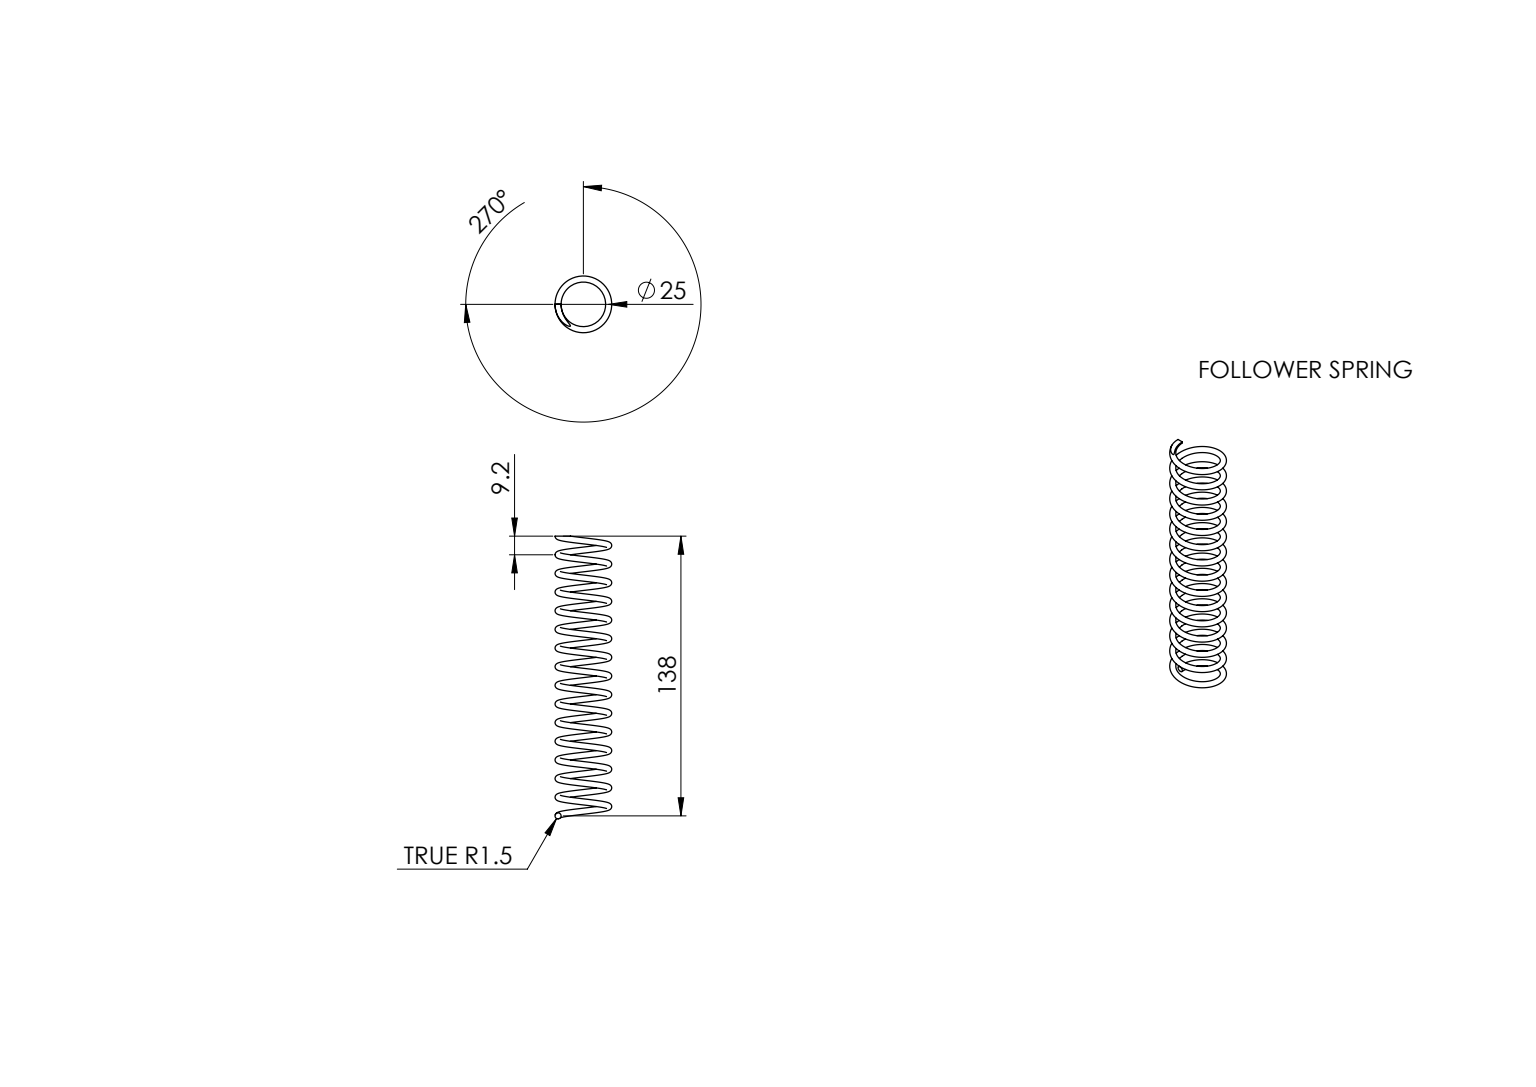
ISO-10303-21;
HEADER;
FILE_DESCRIPTION (('STEP AP214'),
    '1' );
FILE_NAME ('follower spring.step',
    '2026-10-31T03:36:27',
    ( '' ),
    ( '' ),
    'SwSTEP 2.0',
    'SolidWorks 2026',
    '' );
FILE_SCHEMA (( 'AUTOMOTIVE_DESIGN' ));
ENDSEC;

DATA;
#5=CARTESIAN_POINT ( 'NONE',  ( 6.840914352312096547, 71.36018628210143788, -6.594114490232313663 ) ) ;
#12=CARTESIAN_POINT ( 'NONE',  ( 1.715153634034445762, 36.67731371789854933, -9.534712964251895073 ) ) ;
#17=CARTESIAN_POINT ( 'NONE',  ( 6.932735513424201024, 37.25231371789855217, -10.69584247140429412 ) ) ;
#20=CARTESIAN_POINT ( 'NONE',  ( 13.23911966647199812, 140.7523137178985166, 8.632099005475788900 ) ) ;
#36=CARTESIAN_POINT ( 'NONE',  ( -13.23911966647199812, 25.75231371789854506, -8.632099005475788900 ) ) ;
#38=CARTESIAN_POINT ( 'NONE',  ( -9.500000000000005329, 141.5101862821014720, -0.1745138560725176813 ) ) ;
#39=CARTESIAN_POINT ( 'NONE',  ( 2.311890736173175753, 56.12268628210144072, 12.53471296425194836 ) ) ;
#49=CARTESIAN_POINT ( 'NONE',  ( 8.843639120294245259, 94.46481371789855075, 3.474262827703527901 ) ) ;
#56=CARTESIAN_POINT ( 'NONE',  ( -10.49813415416004858, 106.8273137178985479, 7.228626920338840023 ) ) ;
#60=CARTESIAN_POINT ( 'NONE',  ( 0.1745138560722779009, 68.58981371789856496, 12.50000000000000355 ) ) ;
#70=CARTESIAN_POINT ( 'NONE',  ( 12.53471296425194836, 44.62268628210144783, -2.311890736173178418 ) ) ;
#76=CARTESIAN_POINT ( 'NONE',  ( 0.1745138560722779009, 96.18981371789855928, 12.50000000000000355 ) ) ;
#82=CARTESIAN_POINT ( 'NONE',  ( -3.257655550456946880, 82.10231371789853938, -15.46528703574811736 ) ) ;
#86=CARTESIAN_POINT ( 'NONE',  ( -8.715434833791929847, 105.8601862821014521, -8.962234695871762469 ) ) ;
#87=CARTESIAN_POINT ( 'NONE',  ( 13.04141134922759804, 54.97268628210144215, 8.927990412390657937 ) ) ;
#92=CARTESIAN_POINT ( 'NONE',  ( -0.1745138560725817967, 74.81018628210145494, 15.50000000000000533 ) ) ;
#98=CARTESIAN_POINT ( 'NONE',  ( 11.48171059495397728, 45.48518628210145209, 4.944772684328674117 ) ) ;
#101=CARTESIAN_POINT ( 'NONE',  ( 9.534712964251900402, 140.1773137178985564, 1.715153634034445540 ) ) ;
#112=CARTESIAN_POINT ( 'NONE',  ( -12.53471296425194659, 67.62268628210145494, 2.311890736173176641 ) ) ;
#121=CARTESIAN_POINT ( 'NONE',  ( 8.632099005475788900, 46.45231371789854791, -13.23911966647199812 ) ) ;
#127=CARTESIAN_POINT ( 'NONE',  ( -3.474262827703527901, 23.16481371789855359, 8.843639120294245259 ) ) ;
#133=CARTESIAN_POINT ( 'NONE',  ( -3.257655550456946880, 137.3023137178985564, -15.46528703574811736 ) ) ;
#137=CARTESIAN_POINT ( 'NONE',  ( -4.622313124798576922, 42.03518628210144215, -11.61527771782819762 ) ) ;
#143=CARTESIAN_POINT ( 'NONE',  ( 8.710071997420127943, 82.28518628210146346, 3.796722387233375073 ) ) ;
#147=CARTESIAN_POINT ( 'NONE',  ( -12.53471296425194836, 86.02268628210146062, 2.311890736173176641 ) ) ;
#158=CARTESIAN_POINT ( 'NONE',  ( 0.1745138560722779009, 123.7898137178985678, 12.50000000000000355 ) ) ;
#159=CARTESIAN_POINT ( 'NONE',  ( -4.944772684328673229, 121.3851862821014578, 11.48171059495397728 ) ) ;
#166=CARTESIAN_POINT ( 'NONE',  ( -13.23911966647199812, 90.15231371789855075, -8.632099005475788900 ) ) ;
#171=CARTESIAN_POINT ( 'NONE',  ( 9.465287035748106703, 84.40231371789855075, -2.064181346179063237 ) ) ;
#174=CARTESIAN_POINT ( 'NONE',  ( 10.49813415416005213, 47.02731371789855075, -7.228626920338837358 ) ) ;
#178=CARTESIAN_POINT ( 'NONE',  ( 10.49813415415989581, 110.1726862821014521, 7.228626920339068285 ) ) ;
#181=CARTESIAN_POINT ( 'NONE',  ( -7.228626920339069173, 140.0726862821014720, 10.49813415415989581 ) ) ;
#183=CARTESIAN_POINT ( 'NONE',  ( -15.46528703574804986, 104.9976862821014549, -3.257655550457287497 ) ) ;
#184=CARTESIAN_POINT ( 'NONE',  ( 10.49813415415989581, 18.17268628210144499, 7.228626920339069173 ) ) ;
#187=CARTESIAN_POINT ( 'NONE',  ( 6.840914352312096547, 126.5601862821014834, -6.594114490232313663 ) ) ;
#192=CARTESIAN_POINT ( 'NONE',  ( -8.710071997420127943, 68.48518628210145209, -3.796722387233380402 ) ) ;
#202=CARTESIAN_POINT ( 'NONE',  ( -6.594114490232462877, 42.13981371789854791, 6.840914352311949109 ) ) ;
#207=CARTESIAN_POINT ( 'NONE',  ( -8.962234695871565293, 35.23981371789855643, -8.715434833792128799 ) ) ;
#210=CARTESIAN_POINT ( 'NONE',  ( 8.715434833792128799, 19.13981371789855146, -8.962234695871567070 ) ) ;
#225=CARTESIAN_POINT ( 'NONE',  ( -13.23911966647199812, 16.55231371789855643, -8.632099005475788900 ) ) ;
#228=CARTESIAN_POINT ( 'NONE',  ( 7.228626920339068285, 6.672686282101436106, -10.49813415415989581 ) ) ;
#229=CARTESIAN_POINT ( 'NONE',  ( 11.61527771782819940, 44.33518628210145351, -4.622313124798573369 ) ) ;
#241=CARTESIAN_POINT ( 'NONE',  ( -9.465287035748106703, 89.00231371789853085, 2.064181346179061460 ) ) ;
#246=CARTESIAN_POINT ( 'NONE',  ( -6.932735513424201912, 106.2523137178985593, 10.69584247140429412 ) ) ;
#250=CARTESIAN_POINT ( 'NONE',  ( -6.932735513424201912, 69.45231371789856212, 10.69584247140429412 ) ) ;
#258=CARTESIAN_POINT ( 'NONE',  ( 11.48171059495397728, 36.28518628210144925, 4.944772684328674117 ) ) ;
#265=CARTESIAN_POINT ( 'NONE',  ( 11.48171059495408208, 111.7148137178985650, -4.944772684328420986 ) ) ;
#270=CARTESIAN_POINT ( 'NONE',  ( 13.23911966647199812, 76.35231371789853938, 8.632099005475788900 ) ) ;
#274=CARTESIAN_POINT ( 'NONE',  ( -0.1745138560725500443, 111.6101862821014521, 12.50000000000000355 ) ) ;
#275=CARTESIAN_POINT ( 'NONE',  ( 3.257655550457285720, 52.09768628210144925, -15.46528703574804986 ) ) ;
#277=CARTESIAN_POINT ( 'NONE',  ( -13.23911966647218463, 67.04768628210143788, 8.632099005475506459 ) ) ;
#283=CARTESIAN_POINT ( 'NONE',  ( -7.228626920339069173, 48.07268628210143646, 10.49813415415989581 ) ) ;
#286=CARTESIAN_POINT ( 'NONE',  ( -6.840914352312096547, 11.56018628210145316, 6.594114490232313663 ) ) ;
#294=( BOUNDED_SURFACE ( )  B_SPLINE_SURFACE ( 3, 2, ( 
 ( #18814, #1535, #16329, #12732, #30357, #24662, #4381, #10074, #36214, #10256, #21466, #27877, #18433, #18626, #1349, #16146, #21832, #33386, #35842, #32814, #30167, #12921, #7426, #1908, #13478, #15771, #18995, #30552, #27696, #1724, #1160, #24484, #25030, #24849, #4194, #13293, #36399, #22020, #33573, #7609, #36589, #29974, #15579, #27133, #24299, #22575, #25406, #7981, #16516, #20099, #36957, #28063, #16704, #8533, #14222, #33939, #22389, #22760, #19554, #14040, #5486, #31648, #10818, #37144, #28252, #11003, #34121, #8171, #31103, #2098, #5675, #2466, #2281, #11186, #34309, #22946, #28609, #4934, #19746, #5124, #13858, #31283, #30915, #5311, #7796, #19926, #16889, #8353, #28425, #13676, #25589, #31464, #25224, #19373, #22207, #17069, #2646, #25772, #36773, #37324, #34492, #11374, #17256, #28795, #2833, #14405, #25961, #26889, #33756, #178, #26898, #12112, #21043, #17822, #35417, #8900, #545, #14592, #363, #20854, #5864, #23685, #18007, #29736, #12305, #26515, #35231, #26327, #9281, #34673, #20477, #29359, #11927, #32393, #23496, #6433, #3398, #35045, #9093, #6245, #20662, #26144, #29551, #3590, #14967, #15152, #26703, #23879, #734, #32208, #9468, #32580, #28981, #6621, #18197, #3770, #15344, #11556, #23130, #11744, #8718, #20290, #23313, #6047, #31830, #17442, #3022, #34860, #32016, #17633, #29165, #3209, #14783, #7565, #21417, #21604, #4335, #35987, #1117, #1490, #12683, #30311, #21789, #10402, #27092, #15914, #7011, #4153, #1302, #15724, #24254, #32772, #36355, #18770, #18580, #27463, #13064, #1679, #7380, #21233, #12871, #35798, #32960, #9840, #9655, #30122, #24065, #36169, #27274, #24621, #24438, #6807, #10023, #33153, #18383, #35611, #928, #7198, #10215, #33341, #29933, #18951, #13254, #30505, #4525, #21977, #16101, #27653, #24803, #3961, #33522, #19140, #16287, #30689, #4707, #12498, #15535, #25180, #16848, #30870, #16661, #37099, #22164, #2423, #34268, #8494, #28569, #5269, #28386, #5083, #13996, #13435, #36732, #8130, #28207, #25548, #2237, #11148, #34078, #13816, #25363, #22532, #36910, #4893, #22723, #8312, #19701, #19883, #31426, #2607, #31240, #10958, #5447, #25735, #7748, #17029, #14181, #37287, #11335, #22905, #34452, #16474, #20062, #1864, #28019, #22345, #31606, #5633, #27834, #2052, #24984, #10772, #33895, #36542, #10585, #33708, #7937, #19331, #13630, #19513, #31059, #23087, #11700, #3548, #9237, #28944, #6009, #32164, #23454, #17593, #3166, #11886, #31980, #20248, #3356, #23647, #35008, #506, #6202, #29507, #9051, #29124, #20622, #15111, #34631, #14739, #17774, #26287, #320, #29317, #14925, #31788, #26662, #28755, #17404, #23274, #26473, #12072, #35190, #5824, #32538, #14551, #34818, #20811, #692, #23834, #137, #32353, #6392, #17965, #12263, #8676, #8861, #35375, #9426, #2982, #26104, #21003, #20437, #17217, #2795, #14367, #25922, #37467, #11517, #9797, #6968, #21375, #29887, #883, #4982, #24394, #24207, #21563, #7656, #7842, #13524, #26854, #18536, #3918, #1073, #18339, #15301, #6765, #29695, #4799, #32914, #30776, #12643, #12455, #15491, #4110, #24024, #3729, #6578, #30075, #9982, #16377, #35569, #35942, #19415, #33108, #19233, #16565, #1953, #27923, #25080, #9614, #36635, #32728, #22437, #10674, #28110, #12826, #30964, #27047, #22253, #21188, #15682, #33805, #35752, #2141, #13721, #25270, #36821, #10863, #18154, #27233, #1257, #19601, #5356, #14273, #22807, #8580, #25452, #34541, #31511, #25824, #31150, #20149, #23178, #17306, #33983, #17492, #11791, #29027, #28659, #2333, #2697, #28295, #37192, #34171, #37005, #37372, #13904, #11424, #5534, #22991, #11235, #8027, #14641, #22624, #14453, #31696, #5724, #11603, #26190, #34723, #34356, #228, #17121, #28846, #3071, #8401, #11049, #5913, #8216, #2881, #5169, #26009, #19969 ),
 ( #38, #16747, #8767, #20341, #19791, #31883, #31328, #16934, #28476, #2515, #14086, #25637, #8956, #35276, #20902, #17681, #6673, #29218, #23738, #9333, #18246, #1166, #23359, #32443, #6487, #34911, #12164, #15015, #6097, #20527, #23550, #12357, #17869, #26566, #595, #32069, #27139, #24118, #3260, #29981, #3823, #14833, #35095, #26757, #26377, #18058, #29601, #29414, #411, #3638, #11978, #9522, #15208, #787, #23929, #32254, #32634, #35471, #21094, #4013, #29791, #9144, #15400, #26946, #20711, #976, #6295, #21284, #3445, #12552, #35661, #9708, #32820, #6865, #18440, #15585, #7431, #12738, #30173, #1356, #13115, #7245, #36038, #18633, #24305, #27328, #24491, #21651, #4576, #27702, #12927, #18819, #15965, #30363, #10082, #7063, #33205, #30558, #21839, #15778, #4387, #1543, #27518, #24669, #36221, #16153, #4201, #10263, #33391, #19001, #35848, #9890, #21474, #33013, #7003, #26887, #26694, #24055, #9646, #9831, #15527, #29351, #21034, #32385, #3581, #20843, #17809, #9272, #32200, #6799, #35409, #32763, #15144, #3390, #17999, #6612, #26506, #6235, #9085, #32571, #12488, #18373, #14960, #920, #21409, #35601, #21223, #18572, #3952, #29921, #27082, #12104, #1107, #35222, #24430, #12675, #30115, #15335, #32948, #6425, #24244, #23677, #9457, #35789, #538, #4144, #15716, #27267, #1292, #12864, #20654, #23868, #29542, #723, #12296, #18187, #29728, #3761, #7622, #13121, #7810, #10455, #36229, #25236, #21658, #16528, #33770, #10270, #18825, #10640, #1737, #21845, #36600, #33398, #2109, #30369, #7437, #25045, #15972, #22031, #33584, #27708, #4392, #19198, #27524, #19387, #30746, #16341, #13305, #30565, #30929, #4946, #22218, #2296, #28075, #19007, #27890, #13688, #4583, #36785, #1549, #24675, #10830, #4768, #13488, #16159, #22403, #33952, #7993, #33211, #5136, #36973, #16717, #1920, #24863, #19567, #36411, #31117, #28264, #13871, #25421, #7251, #25973, #8547, #5, #14239, #22591, #29183, #37160, #28995, #14419, #11571, #26159, #3225, #192, #25788, #14798, #31661, #5689, #6062, #37337, #5325, #20493, #28624, #34507, #2481, #34687, #11387, #25604, #14608, #11016, #5879, #23145, #11201, #8184, #8733, #2662, #22774, #20305, #34322, #14054, #17272, #2847, #26343, #31846, #11759, #34136, #17458, #8368, #32032, #19758, #19939, #31297, #16901, #28441, #22960, #20113, #31478, #3037, #5502, #28810, #23326, #34877, #17085, #8918, #17649, #12842, #16260, #27248, #30092, #20676, #379, #1087, #27430, #32931, #4124, #15697, #35061, #4678, #1653, #18354, #7539, #1271, #24409, #9110, #11946, #13227, #29903, #19111, #18925, #32743, #12657, #4307, #6779, #35958, #9996, #6983, #3933, #21577, #15507, #24592, #33123, #7168, #18740, #9812, #10185, #13037, #15886, #30661, #1463, #24222, #30281, #36143, #27061, #4497, #35768, #21390, #21762, #33312, #7352, #18552, #30476, #27623, #16074, #23515, #21948, #24776, #33493, #36326, #10373, #34051, #22135, #31030, #27991, #30842, #8098, #7721, #5239, #25335, #16816, #5051, #1838, #8460, #16446, #8280, #31210, #28358, #5415, #20030, #16996, #16634, #31575, #10929, #22504, #22872, #28176, #33681, #37256, #7910, #13787, #19304, #13968, #2206, #4866, #31396, #27810, #22693, #2394, #2021, #24956, #25517, #19483, #13599, #37070, #25149, #36704, #19671, #11116, #5598, #34237, #28536, #13407, #19853, #10743, #11304, #36514, #22316, #10558, #33868, #36883, #2580, #14150, #25704, #34423, #11486, #17556, #29091, #12039, #32499, #17184, #3134, #14702, #28724, #5976, #8831, #37437, #2762, #17370, #6166, #11665, #23055, #26251, #286, #23239, #25888, #11852, #14334, #3320, #23421, #34972, #20403, #26073, #26439, #29280, #32128, #35335, #17740, #28911, #9015, #14891, #5790, #20772, #34601, #8643, #471, #20585, #23606, #20211, #35152, #6357, #9203 ),
 ( #32316, #3508, #14517, #17928, #31760, #29472, #15076, #2947, #26625, #655, #9392, #12226, #23798, #20966, #31944, #101, #34787, #15456, #24361, #32880, #7298, #18689, #15644, #10136, #6927, #30038, #1219, #21341, #9578, #30231, #12986, #12792, #27380, #21528, #18872, #35904, #18499, #9947, #4443, #23989, #4072, #33074, #27194, #7118, #4256, #15832, #21152, #16022, #18118, #6733, #1035, #1410, #24543, #36092, #32689, #21892, #3882, #12606, #21709, #27571, #13168, #27008, #33259, #30421, #1600, #24723, #12418, #24172, #36274, #10319, #18306, #29846, #6545, #35716, #29660, #3696, #15264, #9764, #26817, #846, #35533, #33820, #36652, #19251, #19618, #22639, #16761, #33441, #16947, #11251, #28489, #28125, #1786, #2155, #27756, #10689, #33633, #36461, #13736, #13354, #10878, #30980, #22451, #22267, #7482, #14099, #22081, #13919, #36835, #33998, #11065, #25651, #34186, #7858, #37204, #16580, #25284, #2533, #19430, #24909, #5368, #13542, #4998, #10503, #31164, #8042, #7672, #37019, #19060, #28308, #5187, #30791, #30612, #2347, #25095, #4814, #25469, #16394, #27939, #8231, #19806, #4628, #31341, #16208, #1969, #32083, #34552, #6311, #31524, #8592, #22821, #17135, #8413, #34739, #20354, #28671, #6112, #2709, #23191, #8782, #17694, #610, #34370, #31896, #5925, #19982, #11616, #14467, #5550, #14285, #23003, #11805, #17318, #26021, #49, #25836, #26581, #23564, #37384, #29428, #3273, #11436, #20163, #26204, #31711, #17505, #29040, #28860, #5738, #3084, #2894, #8968, #14653, #241, #23375, #34924, #29233, #20540, #14846, #3462, #26394, #427, #11992, #35109, #9157, #20724, #32268, #17883, #15032, #9728, #4029, #9348, #32458, #3652, #12754, #21300, #15601, #20919, #35864, #1373, #33029, #12179, #33220, #27532, #7259, #6881, #18075, #18456, #6501, #15416, #12374, #15223, #29998, #29617, #27157, #32836, #1180, #26961, #23753, #30379, #803, #30189, #24322, #9906, #27342, #4401, #12944, #991, #15984, #21490, #7080, #18834, #12567, #26772, #21666, #29805, #35676, #23943, #18648, #24133, #35486, #15793, #35292, #4215, #24505, #9535, #21110, #36052, #3838, #32649, #10096, #6690, #18261, #33778, #30937, #16909, #4955, #16724, #13129, #10837, #13313, #22598, #10279, #24871, #1557, #33405, #24683, #13497, #36608, #7444, #22411, #19018, #1928, #25055, #33959, #36237, #21853, #10649, #22227, #30575, #27898, #30753, #4591, #16168, #1746, #28084, #33592, #4776, #16349, #27716, #5331, #2304, #36419, #8191, #19574, #10462, #22041, #16537, #7631, #7817, #19394, #19206, #2116, #13693, #25243, #36794, #8001, #31126, #5143, #28270, #13880, #25428, #36981, #19766, #11024, #34144, #31304, #29001, #17094, #32039, #29190, #17465, #3045, #387, #23334, #26166, #20313, #31486, #8742, #28633, #6269, #14614, #11953, #34695, #14806, #25795, #202, #5510, #17278, #11768, #22781, #34885, #8925, #9118, #3232, #5887, #20501, #5698, #6069, #14062, #37344, #31854, #28819, #26351, #17655, #12, #23522, #2854, #14426, #23153, #25982, #2671, #35069, #20684, #32230, #28450, #2487, #25611, #37168, #11578, #11208, #34330, #8374, #19946, #14246, #11395, #22967, #34514, #8554, #20121, #31669, #29384, #18032, #12328, #27114, #949, #6645, #20878, #33176, #15179, #23902, #18221, #27297, #24461, #760, #12524, #21256, #15369, #32606, #23711, #35444, #4175, #9862, #29575, #3613, #18407, #26726, #9679, #1137, #1328, #6461, #32795, #9492, #21068, #29761, #3792, #26919, #12136, #15746, #35632, #24087, #6831, #29955, #18603, #24277, #569, #3983, #15557, #12705, #35821, #26539, #21441, #3421, #32983, #7036, #30146, #12897, #35252, #36010, #10049, #9306, #14989, #17846, #21625, #32417, #16496, #15938, #36565, #28044, #1512, #7589, #19163, #2077, #22554, #7220, #30713, #4733, #18792, #33546, #36378, #27486 ),
 ( #10607, #13086, #16309, #27855, #13272, #24641, #1888, #4357, #30893, #13459, #25010, #10424, #16123, #13651, #19353, #22186, #25386, #33734, #7399, #7775, #4915, #33363, #10797, #36191, #10235, #25203, #36756, #22371, #21810, #33918, #7961, #19534, #30334, #28231, #18971, #2260, #31082, #30526, #5105, #4548, #21998, #27674, #1700, #16685, #24825, #13839, #36936, #10982, #37308, #8152, #14763, #22744, #14574, #37488, #23110, #11725, #26309, #23297, #11358, #345, #17238, #28779, #29147, #22929, #28407, #6031, #14205, #20084, #25570, #20273, #34474, #11170, #158, #34102, #28965, #8698, #34293, #31264, #34654, #25756, #8336, #11539, #19906, #37123, #2817, #25945, #11911, #31812, #34844, #19726, #5848, #31447, #17617, #5290, #5470, #16870, #2446, #14021, #8517, #31628, #17053, #8882, #28591, #17426, #2628, #3188, #5657, #14388, #3004, #26126, #20460, #32001, #21026, #17798, #6789, #29341, #23860, #35399, #18364, #1281, #23477, #9449, #32561, #35030, #12288, #15133, #6225, #9075, #23668, #12478, #17989, #26685, #715, #20644, #27258, #24233, #3380, #30104, #3942, #32191, #35213, #26878, #14948, #6603, #18178, #29532, #26496, #29718, #527, #9636, #3752, #15326, #909, #32377, #32752, #35591, #24046, #4135, #21213, #9262, #29912, #15518, #12094, #27072, #20834, #6416, #1097, #12665, #35778, #3573, #9821, #21399, #32939, #6993, #18563, #15707, #7921, #7548, #18750, #19121, #7178, #16083, #13047, #30672, #19314, #36524, #4688, #36715, #10196, #1848, #15896, #1662, #22144, #30292, #24965, #30852, #31042, #13612, #27819, #13417, #27633, #10567, #35969, #21772, #16270, #13236, #25160, #33692, #21958, #16457, #24786, #36336, #7731, #10382, #27442, #4877, #28001, #2033, #10755, #22327, #33879, #19495, #33503, #5561, #17146, #4317, #28682, #12853, #24421, #10006, #21588, #33135, #1473, #24603, #36152, #33322, #7361, #18933, #30486, #4507, #23573, #17702, #15042, #34933, #3095, #8978, #620, #20174, #14663, #20549, #26213, #17517, #29051, #23384, #17329, #12189, #14296, #2907, #34750, #12002, #32092, #250, #5750, #18084, #60, #8793, #11814, #23761, #9356, #23202, #6124, #29242, #3283, #14855, #8604, #20365, #26590, #32277, #14479, #26032, #26404, #11627, #437, #35118, #35300, #28872, #9167, #31908, #5938, #20734, #6320, #17892, #34564, #20927, #29437, #3473, #32466, #6509, #2721, #25849, #23014, #37397, #11447, #31722, #3847, #811, #29813, #15231, #27350, #18465, #15800, #35684, #12382, #999, #27164, #9544, #26781, #29625, #4036, #33038, #1380, #23952, #21497, #30387, #18655, #30196, #1564, #24512, #12951, #7087, #32657, #9913, #26970, #24329, #36060, #10104, #35871, #15991, #12575, #4222, #6698, #30006, #21673, #35494, #33227, #7266, #10286, #4408, #18841, #27539, #6889, #13136, #21118, #24142, #24691, #15608, #36244, #1187, #12761, #21860, #33413, #18269, #7451, #3660, #15424, #9736, #21308, #32844, #7825, #22049, #34337, #16358, #25063, #19402, #28458, #25618, #1937, #2124, #22419, #16546, #33787, #24879, #13505, #5339, #11031, #30762, #19216, #19581, #4784, #10845, #2313, #2494, #7639, #33966, #36616, #22236, #30946, #4964, #27906, #13321, #16917, #36802, #10657, #8008, #31133, #19774, #25436, #1755, #28092, #13701, #25252, #5150, #27725, #16731, #4598, #28277, #13887, #36988, #22606, #36428, #34151, #8198, #10471, #16175, #19025, #31311, #14069, #37175, #33600, #11216, #22788, #30582, #34893, #17852, #3240, #6078, #210, #11404, #26174, #5706, #3053, #14812, #32047, #14623, #32236, #17286, #8933, #22975, #34703, #17663, #2679, #20510, #26357, #26546, #9124, #23342, #29198, #23161, #393, #31494, #28827, #11776, #8750, #20691, #11959, #17474, #23529, #20321, #31862, #35075, #5896, #34523, #6275, #29391, #3427, #14995, #575, #12142, #23718, #29009, #8382 ),
 ( #2862, #19953, #5517, #17102, #28641, #14254, #14436, #25803, #37352, #20130, #8563, #31677, #25990, #20, #11586, #7227, #23909, #12714, #3799, #956, #35640, #12531, #21076, #29582, #33183, #15564, #15377, #24284, #35829, #36017, #4182, #18038, #9686, #32614, #29768, #9499, #6468, #35451, #20884, #32990, #24094, #21450, #26926, #3620, #6652, #32802, #15186, #32423, #35258, #21263, #1144, #7043, #26733, #27121, #10056, #9869, #18610, #18800, #30154, #15754, #27305, #767, #1336, #18228, #29962, #12906, #24470, #3990, #21632, #6838, #30341, #12335, #18416, #4366, #15945, #27498, #1519, #13093, #9313, #2086, #25212, #1895, #10805, #10242, #33557, #4922, #13466, #25394, #36763, #33742, #28240, #25018, #10616, #19360, #36574, #27681, #22378, #31089, #30901, #7968, #13659, #36944, #16503, #22195, #28051, #22561, #4556, #7782, #33926, #19542, #5113, #16692, #2269, #1707, #34108, #36198, #24833, #18979, #8160, #4740, #13846, #16131, #10989, #19734, #13279, #31272, #24648, #5297, #16878, #36385, #21818, #28413, #16316, #10432, #2454, #22005, #7596, #33370, #7407, #30536, #19172, #30720, #27863, #23304, #25762, #35036, #22750, #37315, #14027, #8342, #37130, #25952, #11546, #19912, #34850, #31454, #14395, #37495, #8889, #29348, #25576, #23119, #34662, #11176, #2824, #5665, #34299, #5477, #14213, #3011, #8525, #17245, #28787, #17060, #17805, #14771, #28597, #20651, #32007, #2634, #11365, #17432, #22936, #8707, #20280, #20091, #34482, #31819, #31636, #166, #5855, #28971, #14581, #26133, #20467, #11732, #6037, #32197, #17624, #29153, #3194, #26316, #353, #11918, #23484, #9081, #6231, #915, #32759, #533, #27079, #30111, #24240, #3387, #24427, #18756, #35975, #35598, #9268, #9643, #35219, #6609, #3578, #23865, #21405, #32382, #12100, #12484, #29917, #18183, #14957, #21593, #29539, #32945, #6795, #3948, #18569, #33143, #4141, #29724, #7186, #24052, #21220, #10012, #3758, #18370, #15524, #26503, #1104, #15713, #23674, #12672, #15138, #20840, #6422, #26691, #17996, #720, #12293, #15332, #35786, #35404, #9827, #9454, #26884, #6999, #27264, #21031, #32568, #1289, #12860, #8116, #19128, #21964, #13053, #30298, #30492, #19320, #24792, #33510, #7554, #27449, #34067, #31048, #10204, #36899, #10761, #1479, #4513, #33698, #24609, #30677, #4695, #36343, #36158, #16277, #21778, #16463, #27824, #24971, #1854, #1669, #2039, #4883, #7737, #10947, #30858, #16088, #36530, #28007, #18940, #33885, #33328, #7368, #13618, #13423, #22151, #27639, #25167, #19501, #36721, #4324, #13804, #15903, #25352, #10574, #13243, #22333, #10388, #7927, #5069, #16650, #28193, #2223, #22521, #17201, #8661, #22889, #31227, #304, #8297, #121, #23071, #20230, #34803, #11869, #8848, #34438, #23438, #2779, #14353, #14722, #8478, #13983, #29108, #37273, #5617, #11134, #5808, #20047, #34254, #23259, #19688, #14536, #31774, #19869, #16833, #17389, #11320, #31413, #34617, #5432, #22712, #31593, #25535, #14166, #5995, #11685, #17013, #28554, #28930, #2595, #11503, #2966, #3153, #25720, #26090, #28740, #25907, #37453, #20421, #31964, #37087, #17576, #26270, #34991, #5256, #28374, #2410, #15475, #29300, #20986, #32336, #3530, #20792, #17759, #9221, #32145, #6751, #35359, #32711, #15096, #3338, #17947, #6563, #26457, #6186, #9034, #32519, #12438, #18325, #14907, #867, #9783, #35553, #9598, #18520, #3903, #29869, #24007, #12057, #26838, #6374, #3714, #27029, #1053, #15284, #32899, #29492, #21171, #23630, #9410, #12627, #491, #24191, #35737, #27216, #21359, #6951, #30059, #23817, #4093, #35173, #26646, #15665, #18138, #1240, #12811, #29680, #24380, #20606, #675, #12246, #4464, #15852, #16227, #24929, #10342, #13374, #19079, #30811, #21913, #27591, #33462, #4834, #4277, #16042, #7504, #1620, #13191, #24745 ),
 ( #36294, #36482, #10711, #35925, #30631, #4647, #9967, #27778, #33093, #21547, #10155, #19271, #1807, #10524, #16413, #7138, #27960, #22102, #18710, #33651, #7690, #30250, #1991, #21730, #27399, #13563, #25116, #7319, #36674, #1430, #13007, #24563, #36114, #33280, #18893, #30443, #29419, #21291, #12365, #32449, #9716, #6493, #23744, #26952, #24124, #10088, #35666, #9896, #6303, #4020, #18067, #15785, #3452, #29609, #32259, #26572, #17874, #6681, #29797, #601, #15592, #12170, #32640, #18253, #27148, #15022, #35282, #3829, #15408, #9340, #21102, #23935, #20910, #3644, #15214, #32827, #26763, #35478, #9527, #794, #36044, #33019, #982, #1364, #12744, #12558, #6871, #18447, #29989, #1172, #24312, #35855, #21480, #7071, #18639, #30181, #4207, #27333, #12935, #24498, #18730, #18540, #6583, #1077, #1261, #29892, #27238, #9618, #23838, #12459, #12647, #21007, #26666, #3553, #15495, #6972, #12831, #12268, #32919, #4297, #30079, #4114, #13026, #35946, #24398, #15686, #18158, #21380, #887, #35757, #9986, #21567, #9801, #27419, #15115, #3733, #35573, #33112, #24212, #3922, #29699, #18914, #24028, #21193, #27051, #24582, #10175, #32732, #7156, #30271, #15874, #18344, #9429, #6769, #1451, #36134, #15306, #26858, #21750, #33302, #7341, #696, #35379, #32541, #7899, #36502, #33671, #30832, #7711, #16250, #24764, #28348, #10733, #10547, #19473, #31019, #31203, #36873, #13214, #4856, #27799, #24946, #8086, #5041, #33483, #27981, #28165, #19293, #16622, #22123, #36315, #1827, #2011, #10363, #16064, #30466, #16434, #33858, #2195, #1643, #22306, #5228, #13776, #25324, #2385, #10919, #22494, #34041, #7527, #19660, #13396, #25139, #16806, #13959, #36693, #25508, #13586, #37061, #19101, #11108, #22683, #21936, #34227, #8270, #4486, #27611, #30651, #4667, #34592, #5967, #5406, #28717, #92, #8635, #20576, #31935, #28902, #23412, #20203, #5782, #14507, #31752, #22864, #17546, #26242, #26063, #3124, #34778, #32119, #11654, #17360, #23230, #17729, #37246, #2937, #8821, #20394, #29082, #14692, #277, #34413, #29271, #11843, #34963, #12031, #9006, #6155, #23599, #3310, #14882, #26428, #23048, #14141, #463, #37427, #35144, #11295, #19843, #31386, #8452, #16988, #28528, #2570, #25695, #20021, #31567, #5589, #11476, #17176, #2754, #14325, #25879, #3874, #1026, #24535, #12599, #24354, #20763, #18490, #20958, #30222, #17919, #32489, #9195, #3499, #32308, #21143, #6725, #15068, #30030, #26618, #9569, #32681, #4062, #6349, #29463, #18298, #29838, #648, #35524, #839, #12218, #23789, #9382, #35707, #3689, #12407, #23980, #35328, #12978, #9939, #6537, #15822, #27186, #18110, #29653, #24163, #15256, #15448, #26999, #26809, #9758, #21333, #32872, #6919, #15635, #1211, #12784, #35896, #21519, #33065, #7109, #18680, #4248, #27372, #1402, #36642, #24716, #2147, #18864, #27563, #10681, #33623, #27930, #33250, #22260, #25276, #19422, #36084, #19608, #13910, #31156, #30783, #4434, #4806, #30411, #1779, #36266, #19053, #16571, #1592, #7290, #7664, #25087, #13345, #10127, #16753, #10311, #28116, #1961, #16386, #30972, #13532, #10870, #33812, #36453, #7849, #33990, #16015, #10493, #4988, #22072, #24902, #19241, #13728, #13160, #8034, #21701, #21883, #30604, #36828, #22443, #5176, #33433, #7474, #4621, #16199, #28301, #2339, #27749, #8406, #9104, #29371, #23510, #3220, #31333, #19973, #12317, #18019, #37197, #25643, #26527, #11240, #17835, #9294, #35432, #14091, #3409, #31516, #29178, #26339, #14792, #22813, #19797, #23891, #6258, #5540, #14978, #558, #26715, #32406, #8222, #374, #34360, #17127, #3601, #12124, #28482, #35056, #23699, #11941, #35242, #20671, #5361, #32219, #20867, #16939, #11056, #25460, #6446, #29564, #15167, #34178, #747, #9480, #21056, #32594, #6634, #18208, #29750, #3781 ),
 ( #37012, #22631, #2523, #16111, #30321, #15925, #30132, #1500, #938, #24265, #33163, #4164, #27663, #27474, #24448, #18961, #15734, #1315, #10034, #27284, #18394, #13076, #21800, #30515, #15355, #10225, #24631, #3972, #12512, #4346, #32970, #15545, #36180, #27103, #6819, #21613, #7209, #30699, #18781, #4535, #26910, #33352, #1127, #36366, #24076, #12692, #35621, #9667, #21244, #12883, #35998, #32783, #7388, #29944, #1687, #13262, #24814, #35809, #9851, #10413, #21988, #21429, #33535, #7023, #18590, #7575, #19151, #31252, #36743, #7947, #33906, #1875, #8506, #5457, #22175, #11345, #22731, #13447, #4902, #8140, #36553, #5093, #16672, #10783, #24997, #28219, #10594, #28395, #31070, #36922, #19523, #13639, #14006, #19893, #2064, #34280, #10968, #16484, #22542, #5279, #30880, #8323, #33720, #7761, #16858, #2247, #34090, #19341, #2433, #31435, #25558, #4719, #25744, #20071, #37296, #19712, #28032, #37110, #25191, #13826, #22357, #25373, #17039, #11158, #28578, #2616, #14192, #22917, #16296, #34462, #27844, #12082, #35018, #20633, #9249, #23848, #20822, #8871, #35386, #14752, #26296, #26672, #34829, #25933, #3560, #11710, #17605, #23098, #17786, #20448, #8686, #32177, #20260, #35199, #14375, #34641, #6213, #29136, #23465, #28765, #29329, #32363, #14937, #31616, #15121, #9435, #702, #332, #37476, #11898, #11528, #31990, #31798, #14562, #23656, #5836, #2805, #3176, #3366, #6019, #5644, #12275, #17414, #6402, #9062, #26484, #17975, #17227, #29519, #515, #28954, #2993, #26114, #147, #23285, #15312, #30473, #1084, #6980, #12465, #7165, #9809, #35579, #24589, #21013, #15883, #33120, #9624, #18164, #9993, #12654, #21201, #35955, #32740, #24034, #15694, #12840, #36323, #24406, #36141, #32547, #30278, #6776, #4494, #29705, #18351, #6590, #26865, #3739, #32928, #18549, #895, #4305, #29900, #21387, #30089, #27427, #3930, #15504, #4121, #27245, #27058, #1268, #24219, #35765, #21574, #18737, #1461, #13034, #10182, #21759, #33309, #24773, #7349, #18922, #27620, #16071, #1650, #13222, #13784, #4675, #10740, #22313, #16443, #19108, #33865, #7536, #34048, #36701, #5048, #2018, #19301, #19668, #25514, #7718, #28355, #16631, #10555, #28173, #2203, #25146, #13404, #8095, #16813, #25331, #31207, #36880, #22690, #10926, #7907, #22501, #8277, #27807, #19480, #5236, #31027, #2391, #13965, #37067, #24953, #19850, #21945, #22132, #4863, #11113, #34234, #31392, #36511, #25701, #30839, #27988, #5412, #16993, #28533, #13596, #2578, #14147, #10370, #33490, #16256, #30659, #1835, #33678, #11483, #37433, #283, #23052, #29088, #20582, #9202, #25885, #14699, #5787, #2944, #98, #14514, #34598, #31572, #35150, #17553, #17367, #26248, #11849, #469, #6163, #20027, #11662, #8640, #31757, #14888, #23418, #2759, #34784, #34969, #26070, #9012, #28908, #5595, #20208, #8828, #17181, #22869, #37253, #23236, #3131, #32126, #8457, #17737, #12037, #29277, #3317, #20770, #26435, #23605, #32314, #14331, #6355, #20400, #31941, #17926, #29470, #5973, #3506, #15074, #11301, #34419, #28721, #35902, #20964, #1217, #33072, #7296, #27378, #4070, #27192, #3880, #12790, #12224, #35531, #6925, #15453, #1408, #24359, #35714, #30229, #27006, #12605, #32497, #9945, #7116, #18870, #12984, #15642, #21525, #1033, #18687, #23795, #9576, #18496, #24170, #24540, #4254, #9763, #15829, #21339, #32878, #30036, #36090, #29658, #10134, #21707, #33257, #30419, #4440, #26624, #654, #35334, #9390, #6543, #18116, #3694, #15262, #26815, #844, #12415, #23987, #21149, #32687, #6731, #18304, #29844, #25282, #36649, #4812, #19058, #31339, #13352, #22079, #16392, #25467, #22637, #36459, #10687, #19428, #13539, #30789, #21890, #10499, #2345, #8040, #27754, #16206, #16577, #1784, #7855, #36833, #37017, #4626, #30978, #33630, #19248 ) ),
 .UNSPECIFIED., .T., .F., .F. ) 
 B_SPLINE_SURFACE_WITH_KNOTS ( ( 4, 3, 4 ),
 ( 3, 2, 2, 2, 2, 2, 2, 2, 2, 2, 2, 2, 2, 2, 2, 2, 2, 2, 2, 2, 2, 2, 2, 2, 2, 2, 2, 2, 2, 2, 2, 2, 2, 2, 2, 2, 2, 2, 2, 2, 2, 2, 2, 2, 2, 2, 2, 2, 2, 2, 2, 2, 2, 2, 2, 2, 2, 2, 2, 2, 2, 2, 2, 2, 2, 2, 2, 2, 2, 2, 2, 2, 2, 2, 2, 2, 2, 2, 2, 2, 2, 2, 2, 2, 2, 2, 2, 2, 2, 2, 2, 2, 2, 2, 2, 2, 2, 2, 2, 2, 2, 2, 2, 2, 2, 2, 2, 2, 2, 2, 2, 2, 2, 2, 2, 2, 2, 2, 2, 2, 2, 2, 2, 2, 2, 2, 2, 2, 2, 2, 2, 2, 2, 2, 2, 2, 2, 2, 2, 2, 2, 2, 2, 2, 2, 2, 2, 2, 2, 2, 2, 2, 2, 2, 2, 2, 2, 2, 2, 2, 2, 2, 2, 2, 2, 2, 2, 2, 2, 2, 2, 2, 2, 2, 2, 2, 2, 2, 2, 2, 2, 2, 2, 2, 2, 2, 2, 2, 2, 2, 2, 2, 2, 2, 2, 2, 2, 2, 2, 2, 2, 2, 2, 2, 2, 2, 2, 2, 2, 2, 2, 2, 2, 2, 2, 2, 2, 2, 2, 2, 2, 2, 2, 2, 2, 2, 2, 2, 2, 2, 2, 2, 2, 2, 2, 2, 2, 2, 2, 2, 3 ),
 ( 0.000000000000000000, 0.5000000000000000000, 1.000000000000000000 ),
 ( 0.000000000000000000, 0.004166666666666666609, 0.008333333333333333218, 0.01250000000000000069, 0.01666666666666666644, 0.02083333333333333218, 0.02500000000000000139, 0.02916666666666666713, 0.03333333333333333287, 0.03749999999999999861, 0.04166666666666666435, 0.04583333333333333010, 0.05000000000000000278, 0.05416666666666666852, 0.05833333333333333426, 0.06250000000000000000, 0.06666666666666666574, 0.07083333333333333148, 0.07499999999999999722, 0.07916666666666666297, 0.08333333333333332871, 0.08749999999999999445, 0.09166666666666666019, 0.09583333333333333981, 0.1000000000000000056, 0.1041666666666666713, 0.1083333333333333370, 0.1125000000000000028, 0.1166666666666666685, 0.1208333333333333343, 0.1250000000000000000, 0.1291666666666666796, 0.1333333333333333315, 0.1375000000000000111, 0.1416666666666666630, 0.1458333333333333426, 0.1499999999999999944, 0.1541666666666666741, 0.1583333333333333259, 0.1625000000000000056, 0.1666666666666666574, 0.1708333333333333370, 0.1749999999999999889, 0.1791666666666666685, 0.1833333333333333204, 0.1875000000000000000, 0.1916666666666666796, 0.1958333333333333315, 0.2000000000000000111, 0.2041666666666666630, 0.2083333333333333426, 0.2124999999999999944, 0.2166666666666666741, 0.2208333333333333259, 0.2250000000000000056, 0.2291666666666666574, 0.2333333333333333370, 0.2374999999999999889, 0.2416666666666666685, 0.2458333333333333204, 0.2500000000000000000, 0.2541666666666666519, 0.2583333333333333592, 0.2625000000000000111, 0.2666666666666666630, 0.2708333333333333148, 0.2750000000000000222, 0.2791666666666666741, 0.2833333333333333259, 0.2874999999999999778, 0.2916666666666666852, 0.2958333333333333370, 0.2999999999999999889, 0.3041666666666666408, 0.3083333333333333481, 0.3125000000000000000, 0.3166666666666666519, 0.3208333333333333592, 0.3250000000000000111, 0.3291666666666666630, 0.3333333333333333148, 0.3375000000000000222, 0.3416666666666666741, 0.3458333333333333259, 0.3499999999999999778, 0.3541666666666666852, 0.3583333333333333370, 0.3624999999999999889, 0.3666666666666666408, 0.3708333333333333481, 0.3750000000000000000, 0.3791666666666666519, 0.3833333333333333592, 0.3875000000000000111, 0.3916666666666666630, 0.3958333333333333148, 0.4000000000000000222, 0.4041666666666666741, 0.4083333333333333259, 0.4124999999999999778, 0.4166666666666666852, 0.4208333333333333370, 0.4249999999999999889, 0.4291666666666666408, 0.4333333333333333481, 0.4375000000000000000, 0.4416666666666666519, 0.4458333333333333592, 0.4500000000000000111, 0.4541666666666666630, 0.4583333333333333148, 0.4625000000000000222, 0.4666666666666666741, 0.4708333333333333259, 0.4749999999999999778, 0.4791666666666666852, 0.4833333333333333370, 0.4874999999999999889, 0.4916666666666666408, 0.4958333333333333481, 0.5000000000000000000, 0.5041666666666666519, 0.5083333333333333037, 0.5124999999999999556, 0.5166666666666667185, 0.5208333333333333703, 0.5250000000000000222, 0.5291666666666666741, 0.5333333333333333259, 0.5374999999999999778, 0.5416666666666666297, 0.5458333333333332815, 0.5500000000000000444, 0.5541666666666666963, 0.5583333333333333481, 0.5625000000000000000, 0.5666666666666666519, 0.5708333333333333037, 0.5749999999999999556, 0.5791666666666667185, 0.5833333333333333703, 0.5875000000000000222, 0.5916666666666666741, 0.5958333333333333259, 0.5999999999999999778, 0.6041666666666666297, 0.6083333333333332815, 0.6125000000000000444, 0.6166666666666666963, 0.6208333333333333481, 0.6250000000000000000, 0.6291666666666666519, 0.6333333333333333037, 0.6374999999999999556, 0.6416666666666667185, 0.6458333333333333703, 0.6500000000000000222, 0.6541666666666666741, 0.6583333333333333259, 0.6624999999999999778, 0.6666666666666666297, 0.6708333333333332815, 0.6750000000000000444, 0.6791666666666666963, 0.6833333333333333481, 0.6875000000000000000, 0.6916666666666666519, 0.6958333333333333037, 0.6999999999999999556, 0.7041666666666667185, 0.7083333333333333703, 0.7125000000000000222, 0.7166666666666666741, 0.7208333333333333259, 0.7249999999999999778, 0.7291666666666666297, 0.7333333333333332815, 0.7375000000000000444, 0.7416666666666666963, 0.7458333333333333481, 0.7500000000000000000, 0.7541666666666666519, 0.7583333333333333037, 0.7624999999999999556, 0.7666666666666667185, 0.7708333333333333703, 0.7750000000000000222, 0.7791666666666666741, 0.7833333333333333259, 0.7874999999999999778, 0.7916666666666666297, 0.7958333333333332815, 0.8000000000000000444, 0.8041666666666666963, 0.8083333333333333481, 0.8125000000000000000, 0.8166666666666666519, 0.8208333333333333037, 0.8249999999999999556, 0.8291666666666667185, 0.8333333333333333703, 0.8375000000000000222, 0.8416666666666666741, 0.8458333333333333259, 0.8499999999999999778, 0.8541666666666666297, 0.8583333333333332815, 0.8625000000000000444, 0.8666666666666666963, 0.8708333333333333481, 0.8750000000000000000, 0.8791666666666666519, 0.8833333333333333037, 0.8874999999999999556, 0.8916666666666667185, 0.8958333333333333703, 0.9000000000000000222, 0.9041666666666666741, 0.9083333333333333259, 0.9124999999999999778, 0.9166666666666666297, 0.9208333333333332815, 0.9250000000000000444, 0.9291666666666666963, 0.9333333333333333481, 0.9375000000000000000, 0.9416666666666666519, 0.9458333333333333037, 0.9499999999999999556, 0.9541666666666667185, 0.9583333333333333703, 0.9625000000000000222, 0.9666666666666666741, 0.9708333333333333259, 0.9749999999999999778, 0.9791666666666666297, 0.9833333333333332815, 0.9875000000000000444, 0.9916666666666666963, 0.9958333333333333481, 1.000000000000000000 ),
 .UNSPECIFIED. ) 
 GEOMETRIC_REPRESENTATION_ITEM ( )  RATIONAL_B_SPLINE_SURFACE ( (
 ( 1.000000000000000000, 0.9807852804032304306, 1.000000000000000000, 0.9807852804032304306, 1.000000000000000000, 0.9807852804032304306, 1.000000000000000000, 0.9807852804032304306, 1.000000000000000000, 0.9807852804032304306, 1.000000000000000000, 0.9807852804032304306, 1.000000000000000000, 0.9807852804032304306, 1.000000000000000000, 0.9807852804032304306, 1.000000000000000000, 0.9807852804032304306, 1.000000000000000000, 0.9807852804032304306, 1.000000000000000000, 0.9807852804032304306, 1.000000000000000000, 0.9807852804032304306, 1.000000000000000000, 0.9807852804032304306, 1.000000000000000000, 0.9807852804032304306, 1.000000000000000000, 0.9807852804032304306, 1.000000000000000000, 0.9807852804032304306, 1.000000000000000000, 0.9807852804032304306, 1.000000000000000000, 0.9807852804032304306, 1.000000000000000000, 0.9807852804032304306, 1.000000000000000000, 0.9807852804032304306, 1.000000000000000000, 0.9807852804032304306, 1.000000000000000000, 0.9807852804032304306, 1.000000000000000000, 0.9807852804032304306, 1.000000000000000000, 0.9807852804032304306, 1.000000000000000000, 0.9807852804032304306, 1.000000000000000000, 0.9807852804032304306, 1.000000000000000000, 0.9807852804032304306, 1.000000000000000000, 0.9807852804032304306, 1.000000000000000000, 0.9807852804032304306, 1.000000000000000000, 0.9807852804032304306, 1.000000000000000000, 0.9807852804032304306, 1.000000000000000000, 0.9807852804032304306, 1.000000000000000000, 0.9807852804032304306, 1.000000000000000000, 0.9807852804032304306, 1.000000000000000000, 0.9807852804032304306, 1.000000000000000000, 0.9807852804032304306, 1.000000000000000000, 0.9807852804032304306, 1.000000000000000000, 0.9807852804032304306, 1.000000000000000000, 0.9807852804032304306, 1.000000000000000000, 0.9807852804032304306, 1.000000000000000000, 0.9807852804032304306, 1.000000000000000000, 0.9807852804032304306, 1.000000000000000000, 0.9807852804032304306, 1.000000000000000000, 0.9807852804032304306, 1.000000000000000000, 0.9807852804032304306, 1.000000000000000000, 0.9807852804032304306, 1.000000000000000000, 0.9807852804032304306, 1.000000000000000000, 0.9807852804032304306, 1.000000000000000000, 0.9807852804032304306, 1.000000000000000000, 0.9807852804032304306, 1.000000000000000000, 0.9807852804032304306, 1.000000000000000000, 0.9807852804032304306, 1.000000000000000000, 0.9807852804032304306, 1.000000000000000000, 0.9807852804032304306, 1.000000000000000000, 0.9807852804032304306, 1.000000000000000000, 0.9807852804032304306, 1.000000000000000000, 0.9807852804032304306, 1.000000000000000000, 0.9807852804032304306, 1.000000000000000000, 0.9807852804032304306, 1.000000000000000000, 0.9807852804032304306, 1.000000000000000000, 0.9807852804032304306, 1.000000000000000000, 0.9807852804032304306, 1.000000000000000000, 0.9807852804032304306, 1.000000000000000000, 0.9807852804032304306, 1.000000000000000000, 0.9807852804032304306, 1.000000000000000000, 0.9807852804032304306, 1.000000000000000000, 0.9807852804032304306, 1.000000000000000000, 0.9807852804032304306, 1.000000000000000000, 0.9807852804032304306, 1.000000000000000000, 0.9807852804032304306, 1.000000000000000000, 0.9807852804032304306, 1.000000000000000000, 0.9807852804032304306, 1.000000000000000000, 0.9807852804032304306, 1.000000000000000000, 0.9807852804032304306, 1.000000000000000000, 0.9807852804032304306, 1.000000000000000000, 0.9807852804032304306, 1.000000000000000000, 0.9807852804032304306, 1.000000000000000000, 0.9807852804032304306, 1.000000000000000000, 0.9807852804032304306, 1.000000000000000000, 0.9807852804032304306, 1.000000000000000000, 0.9807852804032304306, 1.000000000000000000, 0.9807852804032304306, 1.000000000000000000, 0.9807852804032304306, 1.000000000000000000, 0.9807852804032304306, 1.000000000000000000, 0.9807852804032304306, 1.000000000000000000, 0.9807852804032304306, 1.000000000000000000, 0.9807852804032304306, 1.000000000000000000, 0.9807852804032304306, 1.000000000000000000, 0.9807852804032304306, 1.000000000000000000, 0.9807852804032304306, 1.000000000000000000, 0.9807852804032304306, 1.000000000000000000, 0.9807852804032304306, 1.000000000000000000, 0.9807852804032304306, 1.000000000000000000, 0.9807852804032304306, 1.000000000000000000, 0.9807852804032304306, 1.000000000000000000, 0.9807852804032304306, 1.000000000000000000, 0.9807852804032304306, 1.000000000000000000, 0.9807852804032304306, 1.000000000000000000, 0.9807852804032304306, 1.000000000000000000, 0.9807852804032304306, 1.000000000000000000, 0.9807852804032304306, 1.000000000000000000, 0.9807852804032304306, 1.000000000000000000, 0.9807852804032304306, 1.000000000000000000, 0.9807852804032304306, 1.000000000000000000, 0.9807852804032304306, 1.000000000000000000, 0.9807852804032304306, 1.000000000000000000, 0.9807852804032304306, 1.000000000000000000, 0.9807852804032304306, 1.000000000000000000, 0.9807852804032304306, 1.000000000000000000, 0.9807852804032304306, 1.000000000000000000, 0.9807852804032304306, 1.000000000000000000, 0.9807852804032304306, 1.000000000000000000, 0.9807852804032304306, 1.000000000000000000, 0.9807852804032304306, 1.000000000000000000, 0.9807852804032304306, 1.000000000000000000, 0.9807852804032304306, 1.000000000000000000, 0.9807852804032304306, 1.000000000000000000, 0.9807852804032304306, 1.000000000000000000, 0.9807852804032304306, 1.000000000000000000, 0.9807852804032304306, 1.000000000000000000, 0.9807852804032304306, 1.000000000000000000, 0.9807852804032304306, 1.000000000000000000, 0.9807852804032304306, 1.000000000000000000, 0.9807852804032304306, 1.000000000000000000, 0.9807852804032304306, 1.000000000000000000, 0.9807852804032304306, 1.000000000000000000, 0.9807852804032304306, 1.000000000000000000, 0.9807852804032304306, 1.000000000000000000, 0.9807852804032304306, 1.000000000000000000, 0.9807852804032304306, 1.000000000000000000, 0.9807852804032304306, 1.000000000000000000, 0.9807852804032304306, 1.000000000000000000, 0.9807852804032304306, 1.000000000000000000, 0.9807852804032304306, 1.000000000000000000, 0.9807852804032304306, 1.000000000000000000, 0.9807852804032304306, 1.000000000000000000, 0.9807852804032304306, 1.000000000000000000, 0.9807852804032304306, 1.000000000000000000, 0.9807852804032304306, 1.000000000000000000, 0.9807852804032304306, 1.000000000000000000, 0.9807852804032304306, 1.000000000000000000, 0.9807852804032304306, 1.000000000000000000, 0.9807852804032304306, 1.000000000000000000, 0.9807852804032304306, 1.000000000000000000, 0.9807852804032304306, 1.000000000000000000, 0.9807852804032304306, 1.000000000000000000, 0.9807852804032304306, 1.000000000000000000, 0.9807852804032304306, 1.000000000000000000, 0.9807852804032304306, 1.000000000000000000, 0.9807852804032304306, 1.000000000000000000, 0.9807852804032304306, 1.000000000000000000, 0.9807852804032304306, 1.000000000000000000, 0.9807852804032304306, 1.000000000000000000, 0.9807852804032304306, 1.000000000000000000, 0.9807852804032304306, 1.000000000000000000, 0.9807852804032304306, 1.000000000000000000, 0.9807852804032304306, 1.000000000000000000, 0.9807852804032304306, 1.000000000000000000, 0.9807852804032304306, 1.000000000000000000, 0.9807852804032304306, 1.000000000000000000, 0.9807852804032304306, 1.000000000000000000, 0.9807852804032304306, 1.000000000000000000, 0.9807852804032304306, 1.000000000000000000, 0.9807852804032304306, 1.000000000000000000, 0.9807852804032304306, 1.000000000000000000, 0.9807852804032304306, 1.000000000000000000, 0.9807852804032304306, 1.000000000000000000, 0.9807852804032304306, 1.000000000000000000, 0.9807852804032304306, 1.000000000000000000, 0.9807852804032304306, 1.000000000000000000, 0.9807852804032304306, 1.000000000000000000, 0.9807852804032304306, 1.000000000000000000, 0.9807852804032304306, 1.000000000000000000, 0.9807852804032304306, 1.000000000000000000, 0.9807852804032304306, 1.000000000000000000, 0.9807852804032304306, 1.000000000000000000, 0.9807852804032304306, 1.000000000000000000, 0.9807852804032304306, 1.000000000000000000, 0.9807852804032304306, 1.000000000000000000, 0.9807852804032304306, 1.000000000000000000, 0.9807852804032304306, 1.000000000000000000, 0.9807852804032304306, 1.000000000000000000, 0.9807852804032304306, 1.000000000000000000, 0.9807852804032304306, 1.000000000000000000, 0.9807852804032304306, 1.000000000000000000, 0.9807852804032304306, 1.000000000000000000, 0.9807852804032304306, 1.000000000000000000, 0.9807852804032304306, 1.000000000000000000, 0.9807852804032304306, 1.000000000000000000, 0.9807852804032304306, 1.000000000000000000, 0.9807852804032304306, 1.000000000000000000, 0.9807852804032304306, 1.000000000000000000, 0.9807852804032304306, 1.000000000000000000, 0.9807852804032304306, 1.000000000000000000, 0.9807852804032304306, 1.000000000000000000, 0.9807852804032304306, 1.000000000000000000, 0.9807852804032304306, 1.000000000000000000, 0.9807852804032304306, 1.000000000000000000, 0.9807852804032304306, 1.000000000000000000, 0.9807852804032304306, 1.000000000000000000, 0.9807852804032304306, 1.000000000000000000, 0.9807852804032304306, 1.000000000000000000, 0.9807852804032304306, 1.000000000000000000, 0.9807852804032304306, 1.000000000000000000, 0.9807852804032304306, 1.000000000000000000, 0.9807852804032304306, 1.000000000000000000, 0.9807852804032304306, 1.000000000000000000, 0.9807852804032304306, 1.000000000000000000, 0.9807852804032304306, 1.000000000000000000, 0.9807852804032304306, 1.000000000000000000, 0.9807852804032304306, 1.000000000000000000, 0.9807852804032304306, 1.000000000000000000, 0.9807852804032304306, 1.000000000000000000, 0.9807852804032304306, 1.000000000000000000, 0.9807852804032304306, 1.000000000000000000, 0.9807852804032304306, 1.000000000000000000, 0.9807852804032304306, 1.000000000000000000, 0.9807852804032304306, 1.000000000000000000, 0.9807852804032304306, 1.000000000000000000, 0.9807852804032304306, 1.000000000000000000, 0.9807852804032304306, 1.000000000000000000, 0.9807852804032304306, 1.000000000000000000, 0.9807852804032304306, 1.000000000000000000, 0.9807852804032304306, 1.000000000000000000, 0.9807852804032304306, 1.000000000000000000, 0.9807852804032304306, 1.000000000000000000, 0.9807852804032304306, 1.000000000000000000, 0.9807852804032304306, 1.000000000000000000, 0.9807852804032304306, 1.000000000000000000, 0.9807852804032304306, 1.000000000000000000, 0.9807852804032304306, 1.000000000000000000, 0.9807852804032304306, 1.000000000000000000, 0.9807852804032304306, 1.000000000000000000, 0.9807852804032304306, 1.000000000000000000, 0.9807852804032304306, 1.000000000000000000, 0.9807852804032304306, 1.000000000000000000, 0.9807852804032304306, 1.000000000000000000, 0.9807852804032304306, 1.000000000000000000, 0.9807852804032304306, 1.000000000000000000, 0.9807852804032304306, 1.000000000000000000),
 ( 0.3333333333333333703, 0.3269284268010768657, 0.3333333333333333703, 0.3269284268010768657, 0.3333333333333333703, 0.3269284268010768657, 0.3333333333333333703, 0.3269284268010768657, 0.3333333333333333703, 0.3269284268010768657, 0.3333333333333333703, 0.3269284268010768657, 0.3333333333333333703, 0.3269284268010768657, 0.3333333333333333703, 0.3269284268010768657, 0.3333333333333333703, 0.3269284268010768657, 0.3333333333333333703, 0.3269284268010768657, 0.3333333333333333703, 0.3269284268010768657, 0.3333333333333333703, 0.3269284268010768657, 0.3333333333333333703, 0.3269284268010768657, 0.3333333333333333703, 0.3269284268010768657, 0.3333333333333333703, 0.3269284268010768657, 0.3333333333333333703, 0.3269284268010768657, 0.3333333333333333703, 0.3269284268010768657, 0.3333333333333333703, 0.3269284268010768657, 0.3333333333333333703, 0.3269284268010768657, 0.3333333333333333703, 0.3269284268010768657, 0.3333333333333333703, 0.3269284268010768657, 0.3333333333333333703, 0.3269284268010768657, 0.3333333333333333703, 0.3269284268010768657, 0.3333333333333333703, 0.3269284268010768657, 0.3333333333333333703, 0.3269284268010768657, 0.3333333333333333703, 0.3269284268010768657, 0.3333333333333333703, 0.3269284268010768657, 0.3333333333333333703, 0.3269284268010768657, 0.3333333333333333703, 0.3269284268010768657, 0.3333333333333333703, 0.3269284268010768657, 0.3333333333333333703, 0.3269284268010768657, 0.3333333333333333703, 0.3269284268010768657, 0.3333333333333333703, 0.3269284268010768657, 0.3333333333333333703, 0.3269284268010768657, 0.3333333333333333703, 0.3269284268010768657, 0.3333333333333333703, 0.3269284268010768657, 0.3333333333333333703, 0.3269284268010768657, 0.3333333333333333703, 0.3269284268010768657, 0.3333333333333333703, 0.3269284268010768657, 0.3333333333333333703, 0.3269284268010768657, 0.3333333333333333703, 0.3269284268010768657, 0.3333333333333333703, 0.3269284268010768657, 0.3333333333333333703, 0.3269284268010768657, 0.3333333333333333703, 0.3269284268010768657, 0.3333333333333333703, 0.3269284268010768657, 0.3333333333333333703, 0.3269284268010768657, 0.3333333333333333703, 0.3269284268010768657, 0.3333333333333333703, 0.3269284268010768657, 0.3333333333333333703, 0.3269284268010768657, 0.3333333333333333703, 0.3269284268010768657, 0.3333333333333333703, 0.3269284268010768657, 0.3333333333333333703, 0.3269284268010768657, 0.3333333333333333703, 0.3269284268010768657, 0.3333333333333333703, 0.3269284268010768657, 0.3333333333333333703, 0.3269284268010768657, 0.3333333333333333703, 0.3269284268010768657, 0.3333333333333333703, 0.3269284268010768657, 0.3333333333333333703, 0.3269284268010768657, 0.3333333333333333703, 0.3269284268010768657, 0.3333333333333333703, 0.3269284268010768657, 0.3333333333333333703, 0.3269284268010768657, 0.3333333333333333703, 0.3269284268010768657, 0.3333333333333333703, 0.3269284268010768657, 0.3333333333333333703, 0.3269284268010768657, 0.3333333333333333703, 0.3269284268010768657, 0.3333333333333333703, 0.3269284268010768657, 0.3333333333333333703, 0.3269284268010768657, 0.3333333333333333703, 0.3269284268010768657, 0.3333333333333333703, 0.3269284268010768657, 0.3333333333333333703, 0.3269284268010768657, 0.3333333333333333703, 0.3269284268010768657, 0.3333333333333333703, 0.3269284268010768657, 0.3333333333333333703, 0.3269284268010768657, 0.3333333333333333703, 0.3269284268010768657, 0.3333333333333333703, 0.3269284268010768657, 0.3333333333333333703, 0.3269284268010768657, 0.3333333333333333703, 0.3269284268010768657, 0.3333333333333333703, 0.3269284268010768657, 0.3333333333333333703, 0.3269284268010768657, 0.3333333333333333703, 0.3269284268010768657, 0.3333333333333333703, 0.3269284268010768657, 0.3333333333333333703, 0.3269284268010768657, 0.3333333333333333703, 0.3269284268010768657, 0.3333333333333333703, 0.3269284268010768657, 0.3333333333333333703, 0.3269284268010768657, 0.3333333333333333703, 0.3269284268010768657, 0.3333333333333333703, 0.3269284268010768657, 0.3333333333333333703, 0.3269284268010768657, 0.3333333333333333703, 0.3269284268010768657, 0.3333333333333333703, 0.3269284268010768657, 0.3333333333333333703, 0.3269284268010768657, 0.3333333333333333703, 0.3269284268010768657, 0.3333333333333333703, 0.3269284268010768657, 0.3333333333333333703, 0.3269284268010768657, 0.3333333333333333703, 0.3269284268010768657, 0.3333333333333333703, 0.3269284268010768657, 0.3333333333333333703, 0.3269284268010768657, 0.3333333333333333703, 0.3269284268010768657, 0.3333333333333333703, 0.3269284268010768657, 0.3333333333333333703, 0.3269284268010768657, 0.3333333333333333703, 0.3269284268010768657, 0.3333333333333333703, 0.3269284268010768657, 0.3333333333333333703, 0.3269284268010768657, 0.3333333333333333703, 0.3269284268010768657, 0.3333333333333333703, 0.3269284268010768657, 0.3333333333333333703, 0.3269284268010768657, 0.3333333333333333703, 0.3269284268010768657, 0.3333333333333333703, 0.3269284268010768657, 0.3333333333333333703, 0.3269284268010768657, 0.3333333333333333703, 0.3269284268010768657, 0.3333333333333333703, 0.3269284268010768657, 0.3333333333333333703, 0.3269284268010768657, 0.3333333333333333703, 0.3269284268010768657, 0.3333333333333333703, 0.3269284268010768657, 0.3333333333333333703, 0.3269284268010768657, 0.3333333333333333703, 0.3269284268010768657, 0.3333333333333333703, 0.3269284268010768657, 0.3333333333333333703, 0.3269284268010768657, 0.3333333333333333703, 0.3269284268010768657, 0.3333333333333333703, 0.3269284268010768657, 0.3333333333333333703, 0.3269284268010768657, 0.3333333333333333703, 0.3269284268010768657, 0.3333333333333333703, 0.3269284268010768657, 0.3333333333333333703, 0.3269284268010768657, 0.3333333333333333703, 0.3269284268010768657, 0.3333333333333333703, 0.3269284268010768657, 0.3333333333333333703, 0.3269284268010768657, 0.3333333333333333703, 0.3269284268010768657, 0.3333333333333333703, 0.3269284268010768657, 0.3333333333333333703, 0.3269284268010768657, 0.3333333333333333703, 0.3269284268010768657, 0.3333333333333333703, 0.3269284268010768657, 0.3333333333333333703, 0.3269284268010768657, 0.3333333333333333703, 0.3269284268010768657, 0.3333333333333333703, 0.3269284268010768657, 0.3333333333333333703, 0.3269284268010768657, 0.3333333333333333703, 0.3269284268010768657, 0.3333333333333333703, 0.3269284268010768657, 0.3333333333333333703, 0.3269284268010768657, 0.3333333333333333703, 0.3269284268010768657, 0.3333333333333333703, 0.3269284268010768657, 0.3333333333333333703, 0.3269284268010768657, 0.3333333333333333703, 0.3269284268010768657, 0.3333333333333333703, 0.3269284268010768657, 0.3333333333333333703, 0.3269284268010768657, 0.3333333333333333703, 0.3269284268010768657, 0.3333333333333333703, 0.3269284268010768657, 0.3333333333333333703, 0.3269284268010768657, 0.3333333333333333703, 0.3269284268010768657, 0.3333333333333333703, 0.3269284268010768657, 0.3333333333333333703, 0.3269284268010768657, 0.3333333333333333703, 0.3269284268010768657, 0.3333333333333333703, 0.3269284268010768657, 0.3333333333333333703, 0.3269284268010768657, 0.3333333333333333703, 0.3269284268010768657, 0.3333333333333333703, 0.3269284268010768657, 0.3333333333333333703, 0.3269284268010768657, 0.3333333333333333703, 0.3269284268010768657, 0.3333333333333333703, 0.3269284268010768657, 0.3333333333333333703, 0.3269284268010768657, 0.3333333333333333703, 0.3269284268010768657, 0.3333333333333333703, 0.3269284268010768657, 0.3333333333333333703, 0.3269284268010768657, 0.3333333333333333703, 0.3269284268010768657, 0.3333333333333333703, 0.3269284268010768657, 0.3333333333333333703, 0.3269284268010768657, 0.3333333333333333703, 0.3269284268010768657, 0.3333333333333333703, 0.3269284268010768657, 0.3333333333333333703, 0.3269284268010768657, 0.3333333333333333703, 0.3269284268010768657, 0.3333333333333333703, 0.3269284268010768657, 0.3333333333333333703, 0.3269284268010768657, 0.3333333333333333703, 0.3269284268010768657, 0.3333333333333333703, 0.3269284268010768657, 0.3333333333333333703, 0.3269284268010768657, 0.3333333333333333703, 0.3269284268010768657, 0.3333333333333333703, 0.3269284268010768657, 0.3333333333333333703, 0.3269284268010768657, 0.3333333333333333703, 0.3269284268010768657, 0.3333333333333333703, 0.3269284268010768657, 0.3333333333333333703, 0.3269284268010768657, 0.3333333333333333703, 0.3269284268010768657, 0.3333333333333333703, 0.3269284268010768657, 0.3333333333333333703, 0.3269284268010768657, 0.3333333333333333703, 0.3269284268010768657, 0.3333333333333333703, 0.3269284268010768657, 0.3333333333333333703, 0.3269284268010768657, 0.3333333333333333703, 0.3269284268010768657, 0.3333333333333333703, 0.3269284268010768657, 0.3333333333333333703, 0.3269284268010768657, 0.3333333333333333703, 0.3269284268010768657, 0.3333333333333333703, 0.3269284268010768657, 0.3333333333333333703, 0.3269284268010768657, 0.3333333333333333703, 0.3269284268010768657, 0.3333333333333333703, 0.3269284268010768657, 0.3333333333333333703, 0.3269284268010768657, 0.3333333333333333703, 0.3269284268010768657, 0.3333333333333333703, 0.3269284268010768657, 0.3333333333333333703, 0.3269284268010768657, 0.3333333333333333703, 0.3269284268010768657, 0.3333333333333333703, 0.3269284268010768657, 0.3333333333333333703, 0.3269284268010768657, 0.3333333333333333703, 0.3269284268010768657, 0.3333333333333333703, 0.3269284268010768657, 0.3333333333333333703, 0.3269284268010768657, 0.3333333333333333703, 0.3269284268010768657, 0.3333333333333333703, 0.3269284268010768657, 0.3333333333333333703, 0.3269284268010768657, 0.3333333333333333703, 0.3269284268010768657, 0.3333333333333333703, 0.3269284268010768657, 0.3333333333333333703, 0.3269284268010768657, 0.3333333333333333703, 0.3269284268010768657, 0.3333333333333333703, 0.3269284268010768657, 0.3333333333333333703, 0.3269284268010768657, 0.3333333333333333703, 0.3269284268010768657, 0.3333333333333333703, 0.3269284268010768657, 0.3333333333333333703, 0.3269284268010768657, 0.3333333333333333703, 0.3269284268010768657, 0.3333333333333333703, 0.3269284268010768657, 0.3333333333333333703, 0.3269284268010768657, 0.3333333333333333703, 0.3269284268010768657, 0.3333333333333333703, 0.3269284268010768657, 0.3333333333333333703, 0.3269284268010768657, 0.3333333333333333703, 0.3269284268010768657, 0.3333333333333333703, 0.3269284268010768657, 0.3333333333333333703, 0.3269284268010768657, 0.3333333333333333703, 0.3269284268010768657, 0.3333333333333333703, 0.3269284268010768657, 0.3333333333333333703, 0.3269284268010768657, 0.3333333333333333703, 0.3269284268010768657, 0.3333333333333333703, 0.3269284268010768657, 0.3333333333333333703, 0.3269284268010768657, 0.3333333333333333703, 0.3269284268010768657, 0.3333333333333333703, 0.3269284268010768657, 0.3333333333333333703, 0.3269284268010768657, 0.3333333333333333703, 0.3269284268010768657, 0.3333333333333333703, 0.3269284268010768657, 0.3333333333333333703, 0.3269284268010768657, 0.3333333333333333703, 0.3269284268010768657, 0.3333333333333333703, 0.3269284268010768657, 0.3333333333333333703),
 ( 0.3333333333333333703, 0.3269284268010768657, 0.3333333333333333703, 0.3269284268010768657, 0.3333333333333333703, 0.3269284268010768657, 0.3333333333333333703, 0.3269284268010768657, 0.3333333333333333703, 0.3269284268010768657, 0.3333333333333333703, 0.3269284268010768657, 0.3333333333333333703, 0.3269284268010768657, 0.3333333333333333703, 0.3269284268010768657, 0.3333333333333333703, 0.3269284268010768657, 0.3333333333333333703, 0.3269284268010768657, 0.3333333333333333703, 0.3269284268010768657, 0.3333333333333333703, 0.3269284268010768657, 0.3333333333333333703, 0.3269284268010768657, 0.3333333333333333703, 0.3269284268010768657, 0.3333333333333333703, 0.3269284268010768657, 0.3333333333333333703, 0.3269284268010768657, 0.3333333333333333703, 0.3269284268010768657, 0.3333333333333333703, 0.3269284268010768657, 0.3333333333333333703, 0.3269284268010768657, 0.3333333333333333703, 0.3269284268010768657, 0.3333333333333333703, 0.3269284268010768657, 0.3333333333333333703, 0.3269284268010768657, 0.3333333333333333703, 0.3269284268010768657, 0.3333333333333333703, 0.3269284268010768657, 0.3333333333333333703, 0.3269284268010768657, 0.3333333333333333703, 0.3269284268010768657, 0.3333333333333333703, 0.3269284268010768657, 0.3333333333333333703, 0.3269284268010768657, 0.3333333333333333703, 0.3269284268010768657, 0.3333333333333333703, 0.3269284268010768657, 0.3333333333333333703, 0.3269284268010768657, 0.3333333333333333703, 0.3269284268010768657, 0.3333333333333333703, 0.3269284268010768657, 0.3333333333333333703, 0.3269284268010768657, 0.3333333333333333703, 0.3269284268010768657, 0.3333333333333333703, 0.3269284268010768657, 0.3333333333333333703, 0.3269284268010768657, 0.3333333333333333703, 0.3269284268010768657, 0.3333333333333333703, 0.3269284268010768657, 0.3333333333333333703, 0.3269284268010768657, 0.3333333333333333703, 0.3269284268010768657, 0.3333333333333333703, 0.3269284268010768657, 0.3333333333333333703, 0.3269284268010768657, 0.3333333333333333703, 0.3269284268010768657, 0.3333333333333333703, 0.3269284268010768657, 0.3333333333333333703, 0.3269284268010768657, 0.3333333333333333703, 0.3269284268010768657, 0.3333333333333333703, 0.3269284268010768657, 0.3333333333333333703, 0.3269284268010768657, 0.3333333333333333703, 0.3269284268010768657, 0.3333333333333333703, 0.3269284268010768657, 0.3333333333333333703, 0.3269284268010768657, 0.3333333333333333703, 0.3269284268010768657, 0.3333333333333333703, 0.3269284268010768657, 0.3333333333333333703, 0.3269284268010768657, 0.3333333333333333703, 0.3269284268010768657, 0.3333333333333333703, 0.3269284268010768657, 0.3333333333333333703, 0.3269284268010768657, 0.3333333333333333703, 0.3269284268010768657, 0.3333333333333333703, 0.3269284268010768657, 0.3333333333333333703, 0.3269284268010768657, 0.3333333333333333703, 0.3269284268010768657, 0.3333333333333333703, 0.3269284268010768657, 0.3333333333333333703, 0.3269284268010768657, 0.3333333333333333703, 0.3269284268010768657, 0.3333333333333333703, 0.3269284268010768657, 0.3333333333333333703, 0.3269284268010768657, 0.3333333333333333703, 0.3269284268010768657, 0.3333333333333333703, 0.3269284268010768657, 0.3333333333333333703, 0.3269284268010768657, 0.3333333333333333703, 0.3269284268010768657, 0.3333333333333333703, 0.3269284268010768657, 0.3333333333333333703, 0.3269284268010768657, 0.3333333333333333703, 0.3269284268010768657, 0.3333333333333333703, 0.3269284268010768657, 0.3333333333333333703, 0.3269284268010768657, 0.3333333333333333703, 0.3269284268010768657, 0.3333333333333333703, 0.3269284268010768657, 0.3333333333333333703, 0.3269284268010768657, 0.3333333333333333703, 0.3269284268010768657, 0.3333333333333333703, 0.3269284268010768657, 0.3333333333333333703, 0.3269284268010768657, 0.3333333333333333703, 0.3269284268010768657, 0.3333333333333333703, 0.3269284268010768657, 0.3333333333333333703, 0.3269284268010768657, 0.3333333333333333703, 0.3269284268010768657, 0.3333333333333333703, 0.3269284268010768657, 0.3333333333333333703, 0.3269284268010768657, 0.3333333333333333703, 0.3269284268010768657, 0.3333333333333333703, 0.3269284268010768657, 0.3333333333333333703, 0.3269284268010768657, 0.3333333333333333703, 0.3269284268010768657, 0.3333333333333333703, 0.3269284268010768657, 0.3333333333333333703, 0.3269284268010768657, 0.3333333333333333703, 0.3269284268010768657, 0.3333333333333333703, 0.3269284268010768657, 0.3333333333333333703, 0.3269284268010768657, 0.3333333333333333703, 0.3269284268010768657, 0.3333333333333333703, 0.3269284268010768657, 0.3333333333333333703, 0.3269284268010768657, 0.3333333333333333703, 0.3269284268010768657, 0.3333333333333333703, 0.3269284268010768657, 0.3333333333333333703, 0.3269284268010768657, 0.3333333333333333703, 0.3269284268010768657, 0.3333333333333333703, 0.3269284268010768657, 0.3333333333333333703, 0.3269284268010768657, 0.3333333333333333703, 0.3269284268010768657, 0.3333333333333333703, 0.3269284268010768657, 0.3333333333333333703, 0.3269284268010768657, 0.3333333333333333703, 0.3269284268010768657, 0.3333333333333333703, 0.3269284268010768657, 0.3333333333333333703, 0.3269284268010768657, 0.3333333333333333703, 0.3269284268010768657, 0.3333333333333333703, 0.3269284268010768657, 0.3333333333333333703, 0.3269284268010768657, 0.3333333333333333703, 0.3269284268010768657, 0.3333333333333333703, 0.3269284268010768657, 0.3333333333333333703, 0.3269284268010768657, 0.3333333333333333703, 0.3269284268010768657, 0.3333333333333333703, 0.3269284268010768657, 0.3333333333333333703, 0.3269284268010768657, 0.3333333333333333703, 0.3269284268010768657, 0.3333333333333333703, 0.3269284268010768657, 0.3333333333333333703, 0.3269284268010768657, 0.3333333333333333703, 0.3269284268010768657, 0.3333333333333333703, 0.3269284268010768657, 0.3333333333333333703, 0.3269284268010768657, 0.3333333333333333703, 0.3269284268010768657, 0.3333333333333333703, 0.3269284268010768657, 0.3333333333333333703, 0.3269284268010768657, 0.3333333333333333703, 0.3269284268010768657, 0.3333333333333333703, 0.3269284268010768657, 0.3333333333333333703, 0.3269284268010768657, 0.3333333333333333703, 0.3269284268010768657, 0.3333333333333333703, 0.3269284268010768657, 0.3333333333333333703, 0.3269284268010768657, 0.3333333333333333703, 0.3269284268010768657, 0.3333333333333333703, 0.3269284268010768657, 0.3333333333333333703, 0.3269284268010768657, 0.3333333333333333703, 0.3269284268010768657, 0.3333333333333333703, 0.3269284268010768657, 0.3333333333333333703, 0.3269284268010768657, 0.3333333333333333703, 0.3269284268010768657, 0.3333333333333333703, 0.3269284268010768657, 0.3333333333333333703, 0.3269284268010768657, 0.3333333333333333703, 0.3269284268010768657, 0.3333333333333333703, 0.3269284268010768657, 0.3333333333333333703, 0.3269284268010768657, 0.3333333333333333703, 0.3269284268010768657, 0.3333333333333333703, 0.3269284268010768657, 0.3333333333333333703, 0.3269284268010768657, 0.3333333333333333703, 0.3269284268010768657, 0.3333333333333333703, 0.3269284268010768657, 0.3333333333333333703, 0.3269284268010768657, 0.3333333333333333703, 0.3269284268010768657, 0.3333333333333333703, 0.3269284268010768657, 0.3333333333333333703, 0.3269284268010768657, 0.3333333333333333703, 0.3269284268010768657, 0.3333333333333333703, 0.3269284268010768657, 0.3333333333333333703, 0.3269284268010768657, 0.3333333333333333703, 0.3269284268010768657, 0.3333333333333333703, 0.3269284268010768657, 0.3333333333333333703, 0.3269284268010768657, 0.3333333333333333703, 0.3269284268010768657, 0.3333333333333333703, 0.3269284268010768657, 0.3333333333333333703, 0.3269284268010768657, 0.3333333333333333703, 0.3269284268010768657, 0.3333333333333333703, 0.3269284268010768657, 0.3333333333333333703, 0.3269284268010768657, 0.3333333333333333703, 0.3269284268010768657, 0.3333333333333333703, 0.3269284268010768657, 0.3333333333333333703, 0.3269284268010768657, 0.3333333333333333703, 0.3269284268010768657, 0.3333333333333333703, 0.3269284268010768657, 0.3333333333333333703, 0.3269284268010768657, 0.3333333333333333703, 0.3269284268010768657, 0.3333333333333333703, 0.3269284268010768657, 0.3333333333333333703, 0.3269284268010768657, 0.3333333333333333703, 0.3269284268010768657, 0.3333333333333333703, 0.3269284268010768657, 0.3333333333333333703, 0.3269284268010768657, 0.3333333333333333703, 0.3269284268010768657, 0.3333333333333333703, 0.3269284268010768657, 0.3333333333333333703, 0.3269284268010768657, 0.3333333333333333703, 0.3269284268010768657, 0.3333333333333333703, 0.3269284268010768657, 0.3333333333333333703, 0.3269284268010768657, 0.3333333333333333703, 0.3269284268010768657, 0.3333333333333333703, 0.3269284268010768657, 0.3333333333333333703, 0.3269284268010768657, 0.3333333333333333703, 0.3269284268010768657, 0.3333333333333333703, 0.3269284268010768657, 0.3333333333333333703, 0.3269284268010768657, 0.3333333333333333703, 0.3269284268010768657, 0.3333333333333333703, 0.3269284268010768657, 0.3333333333333333703, 0.3269284268010768657, 0.3333333333333333703, 0.3269284268010768657, 0.3333333333333333703, 0.3269284268010768657, 0.3333333333333333703, 0.3269284268010768657, 0.3333333333333333703, 0.3269284268010768657, 0.3333333333333333703, 0.3269284268010768657, 0.3333333333333333703, 0.3269284268010768657, 0.3333333333333333703, 0.3269284268010768657, 0.3333333333333333703, 0.3269284268010768657, 0.3333333333333333703, 0.3269284268010768657, 0.3333333333333333703, 0.3269284268010768657, 0.3333333333333333703, 0.3269284268010768657, 0.3333333333333333703, 0.3269284268010768657, 0.3333333333333333703, 0.3269284268010768657, 0.3333333333333333703, 0.3269284268010768657, 0.3333333333333333703, 0.3269284268010768657, 0.3333333333333333703, 0.3269284268010768657, 0.3333333333333333703, 0.3269284268010768657, 0.3333333333333333703, 0.3269284268010768657, 0.3333333333333333703, 0.3269284268010768657, 0.3333333333333333703, 0.3269284268010768657, 0.3333333333333333703, 0.3269284268010768657, 0.3333333333333333703, 0.3269284268010768657, 0.3333333333333333703, 0.3269284268010768657, 0.3333333333333333703, 0.3269284268010768657, 0.3333333333333333703, 0.3269284268010768657, 0.3333333333333333703, 0.3269284268010768657, 0.3333333333333333703, 0.3269284268010768657, 0.3333333333333333703, 0.3269284268010768657, 0.3333333333333333703, 0.3269284268010768657, 0.3333333333333333703, 0.3269284268010768657, 0.3333333333333333703, 0.3269284268010768657, 0.3333333333333333703, 0.3269284268010768657, 0.3333333333333333703, 0.3269284268010768657, 0.3333333333333333703, 0.3269284268010768657, 0.3333333333333333703, 0.3269284268010768657, 0.3333333333333333703, 0.3269284268010768657, 0.3333333333333333703, 0.3269284268010768657, 0.3333333333333333703, 0.3269284268010768657, 0.3333333333333333703, 0.3269284268010768657, 0.3333333333333333703, 0.3269284268010768657, 0.3333333333333333703, 0.3269284268010768657, 0.3333333333333333703, 0.3269284268010768657, 0.3333333333333333703, 0.3269284268010768657, 0.3333333333333333703, 0.3269284268010768657, 0.3333333333333333703),
 ( 1.000000000000000000, 0.9807852804032304306, 1.000000000000000000, 0.9807852804032304306, 1.000000000000000000, 0.9807852804032304306, 1.000000000000000000, 0.9807852804032304306, 1.000000000000000000, 0.9807852804032304306, 1.000000000000000000, 0.9807852804032304306, 1.000000000000000000, 0.9807852804032304306, 1.000000000000000000, 0.9807852804032304306, 1.000000000000000000, 0.9807852804032304306, 1.000000000000000000, 0.9807852804032304306, 1.000000000000000000, 0.9807852804032304306, 1.000000000000000000, 0.9807852804032304306, 1.000000000000000000, 0.9807852804032304306, 1.000000000000000000, 0.9807852804032304306, 1.000000000000000000, 0.9807852804032304306, 1.000000000000000000, 0.9807852804032304306, 1.000000000000000000, 0.9807852804032304306, 1.000000000000000000, 0.9807852804032304306, 1.000000000000000000, 0.9807852804032304306, 1.000000000000000000, 0.9807852804032304306, 1.000000000000000000, 0.9807852804032304306, 1.000000000000000000, 0.9807852804032304306, 1.000000000000000000, 0.9807852804032304306, 1.000000000000000000, 0.9807852804032304306, 1.000000000000000000, 0.9807852804032304306, 1.000000000000000000, 0.9807852804032304306, 1.000000000000000000, 0.9807852804032304306, 1.000000000000000000, 0.9807852804032304306, 1.000000000000000000, 0.9807852804032304306, 1.000000000000000000, 0.9807852804032304306, 1.000000000000000000, 0.9807852804032304306, 1.000000000000000000, 0.9807852804032304306, 1.000000000000000000, 0.9807852804032304306, 1.000000000000000000, 0.9807852804032304306, 1.000000000000000000, 0.9807852804032304306, 1.000000000000000000, 0.9807852804032304306, 1.000000000000000000, 0.9807852804032304306, 1.000000000000000000, 0.9807852804032304306, 1.000000000000000000, 0.9807852804032304306, 1.000000000000000000, 0.9807852804032304306, 1.000000000000000000, 0.9807852804032304306, 1.000000000000000000, 0.9807852804032304306, 1.000000000000000000, 0.9807852804032304306, 1.000000000000000000, 0.9807852804032304306, 1.000000000000000000, 0.9807852804032304306, 1.000000000000000000, 0.9807852804032304306, 1.000000000000000000, 0.9807852804032304306, 1.000000000000000000, 0.9807852804032304306, 1.000000000000000000, 0.9807852804032304306, 1.000000000000000000, 0.9807852804032304306, 1.000000000000000000, 0.9807852804032304306, 1.000000000000000000, 0.9807852804032304306, 1.000000000000000000, 0.9807852804032304306, 1.000000000000000000, 0.9807852804032304306, 1.000000000000000000, 0.9807852804032304306, 1.000000000000000000, 0.9807852804032304306, 1.000000000000000000, 0.9807852804032304306, 1.000000000000000000, 0.9807852804032304306, 1.000000000000000000, 0.9807852804032304306, 1.000000000000000000, 0.9807852804032304306, 1.000000000000000000, 0.9807852804032304306, 1.000000000000000000, 0.9807852804032304306, 1.000000000000000000, 0.9807852804032304306, 1.000000000000000000, 0.9807852804032304306, 1.000000000000000000, 0.9807852804032304306, 1.000000000000000000, 0.9807852804032304306, 1.000000000000000000, 0.9807852804032304306, 1.000000000000000000, 0.9807852804032304306, 1.000000000000000000, 0.9807852804032304306, 1.000000000000000000, 0.9807852804032304306, 1.000000000000000000, 0.9807852804032304306, 1.000000000000000000, 0.9807852804032304306, 1.000000000000000000, 0.9807852804032304306, 1.000000000000000000, 0.9807852804032304306, 1.000000000000000000, 0.9807852804032304306, 1.000000000000000000, 0.9807852804032304306, 1.000000000000000000, 0.9807852804032304306, 1.000000000000000000, 0.9807852804032304306, 1.000000000000000000, 0.9807852804032304306, 1.000000000000000000, 0.9807852804032304306, 1.000000000000000000, 0.9807852804032304306, 1.000000000000000000, 0.9807852804032304306, 1.000000000000000000, 0.9807852804032304306, 1.000000000000000000, 0.9807852804032304306, 1.000000000000000000, 0.9807852804032304306, 1.000000000000000000, 0.9807852804032304306, 1.000000000000000000, 0.9807852804032304306, 1.000000000000000000, 0.9807852804032304306, 1.000000000000000000, 0.9807852804032304306, 1.000000000000000000, 0.9807852804032304306, 1.000000000000000000, 0.9807852804032304306, 1.000000000000000000, 0.9807852804032304306, 1.000000000000000000, 0.9807852804032304306, 1.000000000000000000, 0.9807852804032304306, 1.000000000000000000, 0.9807852804032304306, 1.000000000000000000, 0.9807852804032304306, 1.000000000000000000, 0.9807852804032304306, 1.000000000000000000, 0.9807852804032304306, 1.000000000000000000, 0.9807852804032304306, 1.000000000000000000, 0.9807852804032304306, 1.000000000000000000, 0.9807852804032304306, 1.000000000000000000, 0.9807852804032304306, 1.000000000000000000, 0.9807852804032304306, 1.000000000000000000, 0.9807852804032304306, 1.000000000000000000, 0.9807852804032304306, 1.000000000000000000, 0.9807852804032304306, 1.000000000000000000, 0.9807852804032304306, 1.000000000000000000, 0.9807852804032304306, 1.000000000000000000, 0.9807852804032304306, 1.000000000000000000, 0.9807852804032304306, 1.000000000000000000, 0.9807852804032304306, 1.000000000000000000, 0.9807852804032304306, 1.000000000000000000, 0.9807852804032304306, 1.000000000000000000, 0.9807852804032304306, 1.000000000000000000, 0.9807852804032304306, 1.000000000000000000, 0.9807852804032304306, 1.000000000000000000, 0.9807852804032304306, 1.000000000000000000, 0.9807852804032304306, 1.000000000000000000, 0.9807852804032304306, 1.000000000000000000, 0.9807852804032304306, 1.000000000000000000, 0.9807852804032304306, 1.000000000000000000, 0.9807852804032304306, 1.000000000000000000, 0.9807852804032304306, 1.000000000000000000, 0.9807852804032304306, 1.000000000000000000, 0.9807852804032304306, 1.000000000000000000, 0.9807852804032304306, 1.000000000000000000, 0.9807852804032304306, 1.000000000000000000, 0.9807852804032304306, 1.000000000000000000, 0.9807852804032304306, 1.000000000000000000, 0.9807852804032304306, 1.000000000000000000, 0.9807852804032304306, 1.000000000000000000, 0.9807852804032304306, 1.000000000000000000, 0.9807852804032304306, 1.000000000000000000, 0.9807852804032304306, 1.000000000000000000, 0.9807852804032304306, 1.000000000000000000, 0.9807852804032304306, 1.000000000000000000, 0.9807852804032304306, 1.000000000000000000, 0.9807852804032304306, 1.000000000000000000, 0.9807852804032304306, 1.000000000000000000, 0.9807852804032304306, 1.000000000000000000, 0.9807852804032304306, 1.000000000000000000, 0.9807852804032304306, 1.000000000000000000, 0.9807852804032304306, 1.000000000000000000, 0.9807852804032304306, 1.000000000000000000, 0.9807852804032304306, 1.000000000000000000, 0.9807852804032304306, 1.000000000000000000, 0.9807852804032304306, 1.000000000000000000, 0.9807852804032304306, 1.000000000000000000, 0.9807852804032304306, 1.000000000000000000, 0.9807852804032304306, 1.000000000000000000, 0.9807852804032304306, 1.000000000000000000, 0.9807852804032304306, 1.000000000000000000, 0.9807852804032304306, 1.000000000000000000, 0.9807852804032304306, 1.000000000000000000, 0.9807852804032304306, 1.000000000000000000, 0.9807852804032304306, 1.000000000000000000, 0.9807852804032304306, 1.000000000000000000, 0.9807852804032304306, 1.000000000000000000, 0.9807852804032304306, 1.000000000000000000, 0.9807852804032304306, 1.000000000000000000, 0.9807852804032304306, 1.000000000000000000, 0.9807852804032304306, 1.000000000000000000, 0.9807852804032304306, 1.000000000000000000, 0.9807852804032304306, 1.000000000000000000, 0.9807852804032304306, 1.000000000000000000, 0.9807852804032304306, 1.000000000000000000, 0.9807852804032304306, 1.000000000000000000, 0.9807852804032304306, 1.000000000000000000, 0.9807852804032304306, 1.000000000000000000, 0.9807852804032304306, 1.000000000000000000, 0.9807852804032304306, 1.000000000000000000, 0.9807852804032304306, 1.000000000000000000, 0.9807852804032304306, 1.000000000000000000, 0.9807852804032304306, 1.000000000000000000, 0.9807852804032304306, 1.000000000000000000, 0.9807852804032304306, 1.000000000000000000, 0.9807852804032304306, 1.000000000000000000, 0.9807852804032304306, 1.000000000000000000, 0.9807852804032304306, 1.000000000000000000, 0.9807852804032304306, 1.000000000000000000, 0.9807852804032304306, 1.000000000000000000, 0.9807852804032304306, 1.000000000000000000, 0.9807852804032304306, 1.000000000000000000, 0.9807852804032304306, 1.000000000000000000, 0.9807852804032304306, 1.000000000000000000, 0.9807852804032304306, 1.000000000000000000, 0.9807852804032304306, 1.000000000000000000, 0.9807852804032304306, 1.000000000000000000, 0.9807852804032304306, 1.000000000000000000, 0.9807852804032304306, 1.000000000000000000, 0.9807852804032304306, 1.000000000000000000, 0.9807852804032304306, 1.000000000000000000, 0.9807852804032304306, 1.000000000000000000, 0.9807852804032304306, 1.000000000000000000, 0.9807852804032304306, 1.000000000000000000, 0.9807852804032304306, 1.000000000000000000, 0.9807852804032304306, 1.000000000000000000, 0.9807852804032304306, 1.000000000000000000, 0.9807852804032304306, 1.000000000000000000, 0.9807852804032304306, 1.000000000000000000, 0.9807852804032304306, 1.000000000000000000, 0.9807852804032304306, 1.000000000000000000, 0.9807852804032304306, 1.000000000000000000, 0.9807852804032304306, 1.000000000000000000, 0.9807852804032304306, 1.000000000000000000, 0.9807852804032304306, 1.000000000000000000, 0.9807852804032304306, 1.000000000000000000, 0.9807852804032304306, 1.000000000000000000, 0.9807852804032304306, 1.000000000000000000, 0.9807852804032304306, 1.000000000000000000, 0.9807852804032304306, 1.000000000000000000, 0.9807852804032304306, 1.000000000000000000, 0.9807852804032304306, 1.000000000000000000, 0.9807852804032304306, 1.000000000000000000, 0.9807852804032304306, 1.000000000000000000, 0.9807852804032304306, 1.000000000000000000, 0.9807852804032304306, 1.000000000000000000, 0.9807852804032304306, 1.000000000000000000, 0.9807852804032304306, 1.000000000000000000, 0.9807852804032304306, 1.000000000000000000, 0.9807852804032304306, 1.000000000000000000, 0.9807852804032304306, 1.000000000000000000, 0.9807852804032304306, 1.000000000000000000, 0.9807852804032304306, 1.000000000000000000, 0.9807852804032304306, 1.000000000000000000, 0.9807852804032304306, 1.000000000000000000, 0.9807852804032304306, 1.000000000000000000, 0.9807852804032304306, 1.000000000000000000, 0.9807852804032304306, 1.000000000000000000, 0.9807852804032304306, 1.000000000000000000, 0.9807852804032304306, 1.000000000000000000, 0.9807852804032304306, 1.000000000000000000, 0.9807852804032304306, 1.000000000000000000, 0.9807852804032304306, 1.000000000000000000, 0.9807852804032304306, 1.000000000000000000, 0.9807852804032304306, 1.000000000000000000, 0.9807852804032304306, 1.000000000000000000, 0.9807852804032304306, 1.000000000000000000, 0.9807852804032304306, 1.000000000000000000, 0.9807852804032304306, 1.000000000000000000),
 ( 0.3333333333333333703, 0.3269284268010768657, 0.3333333333333333703, 0.3269284268010768657, 0.3333333333333333703, 0.3269284268010768657, 0.3333333333333333703, 0.3269284268010768657, 0.3333333333333333703, 0.3269284268010768657, 0.3333333333333333703, 0.3269284268010768657, 0.3333333333333333703, 0.3269284268010768657, 0.3333333333333333703, 0.3269284268010768657, 0.3333333333333333703, 0.3269284268010768657, 0.3333333333333333703, 0.3269284268010768657, 0.3333333333333333703, 0.3269284268010768657, 0.3333333333333333703, 0.3269284268010768657, 0.3333333333333333703, 0.3269284268010768657, 0.3333333333333333703, 0.3269284268010768657, 0.3333333333333333703, 0.3269284268010768657, 0.3333333333333333703, 0.3269284268010768657, 0.3333333333333333703, 0.3269284268010768657, 0.3333333333333333703, 0.3269284268010768657, 0.3333333333333333703, 0.3269284268010768657, 0.3333333333333333703, 0.3269284268010768657, 0.3333333333333333703, 0.3269284268010768657, 0.3333333333333333703, 0.3269284268010768657, 0.3333333333333333703, 0.3269284268010768657, 0.3333333333333333703, 0.3269284268010768657, 0.3333333333333333703, 0.3269284268010768657, 0.3333333333333333703, 0.3269284268010768657, 0.3333333333333333703, 0.3269284268010768657, 0.3333333333333333703, 0.3269284268010768657, 0.3333333333333333703, 0.3269284268010768657, 0.3333333333333333703, 0.3269284268010768657, 0.3333333333333333703, 0.3269284268010768657, 0.3333333333333333703, 0.3269284268010768657, 0.3333333333333333703, 0.3269284268010768657, 0.3333333333333333703, 0.3269284268010768657, 0.3333333333333333703, 0.3269284268010768657, 0.3333333333333333703, 0.3269284268010768657, 0.3333333333333333703, 0.3269284268010768657, 0.3333333333333333703, 0.3269284268010768657, 0.3333333333333333703, 0.3269284268010768657, 0.3333333333333333703, 0.3269284268010768657, 0.3333333333333333703, 0.3269284268010768657, 0.3333333333333333703, 0.3269284268010768657, 0.3333333333333333703, 0.3269284268010768657, 0.3333333333333333703, 0.3269284268010768657, 0.3333333333333333703, 0.3269284268010768657, 0.3333333333333333703, 0.3269284268010768657, 0.3333333333333333703, 0.3269284268010768657, 0.3333333333333333703, 0.3269284268010768657, 0.3333333333333333703, 0.3269284268010768657, 0.3333333333333333703, 0.3269284268010768657, 0.3333333333333333703, 0.3269284268010768657, 0.3333333333333333703, 0.3269284268010768657, 0.3333333333333333703, 0.3269284268010768657, 0.3333333333333333703, 0.3269284268010768657, 0.3333333333333333703, 0.3269284268010768657, 0.3333333333333333703, 0.3269284268010768657, 0.3333333333333333703, 0.3269284268010768657, 0.3333333333333333703, 0.3269284268010768657, 0.3333333333333333703, 0.3269284268010768657, 0.3333333333333333703, 0.3269284268010768657, 0.3333333333333333703, 0.3269284268010768657, 0.3333333333333333703, 0.3269284268010768657, 0.3333333333333333703, 0.3269284268010768657, 0.3333333333333333703, 0.3269284268010768657, 0.3333333333333333703, 0.3269284268010768657, 0.3333333333333333703, 0.3269284268010768657, 0.3333333333333333703, 0.3269284268010768657, 0.3333333333333333703, 0.3269284268010768657, 0.3333333333333333703, 0.3269284268010768657, 0.3333333333333333703, 0.3269284268010768657, 0.3333333333333333703, 0.3269284268010768657, 0.3333333333333333703, 0.3269284268010768657, 0.3333333333333333703, 0.3269284268010768657, 0.3333333333333333703, 0.3269284268010768657, 0.3333333333333333703, 0.3269284268010768657, 0.3333333333333333703, 0.3269284268010768657, 0.3333333333333333703, 0.3269284268010768657, 0.3333333333333333703, 0.3269284268010768657, 0.3333333333333333703, 0.3269284268010768657, 0.3333333333333333703, 0.3269284268010768657, 0.3333333333333333703, 0.3269284268010768657, 0.3333333333333333703, 0.3269284268010768657, 0.3333333333333333703, 0.3269284268010768657, 0.3333333333333333703, 0.3269284268010768657, 0.3333333333333333703, 0.3269284268010768657, 0.3333333333333333703, 0.3269284268010768657, 0.3333333333333333703, 0.3269284268010768657, 0.3333333333333333703, 0.3269284268010768657, 0.3333333333333333703, 0.3269284268010768657, 0.3333333333333333703, 0.3269284268010768657, 0.3333333333333333703, 0.3269284268010768657, 0.3333333333333333703, 0.3269284268010768657, 0.3333333333333333703, 0.3269284268010768657, 0.3333333333333333703, 0.3269284268010768657, 0.3333333333333333703, 0.3269284268010768657, 0.3333333333333333703, 0.3269284268010768657, 0.3333333333333333703, 0.3269284268010768657, 0.3333333333333333703, 0.3269284268010768657, 0.3333333333333333703, 0.3269284268010768657, 0.3333333333333333703, 0.3269284268010768657, 0.3333333333333333703, 0.3269284268010768657, 0.3333333333333333703, 0.3269284268010768657, 0.3333333333333333703, 0.3269284268010768657, 0.3333333333333333703, 0.3269284268010768657, 0.3333333333333333703, 0.3269284268010768657, 0.3333333333333333703, 0.3269284268010768657, 0.3333333333333333703, 0.3269284268010768657, 0.3333333333333333703, 0.3269284268010768657, 0.3333333333333333703, 0.3269284268010768657, 0.3333333333333333703, 0.3269284268010768657, 0.3333333333333333703, 0.3269284268010768657, 0.3333333333333333703, 0.3269284268010768657, 0.3333333333333333703, 0.3269284268010768657, 0.3333333333333333703, 0.3269284268010768657, 0.3333333333333333703, 0.3269284268010768657, 0.3333333333333333703, 0.3269284268010768657, 0.3333333333333333703, 0.3269284268010768657, 0.3333333333333333703, 0.3269284268010768657, 0.3333333333333333703, 0.3269284268010768657, 0.3333333333333333703, 0.3269284268010768657, 0.3333333333333333703, 0.3269284268010768657, 0.3333333333333333703, 0.3269284268010768657, 0.3333333333333333703, 0.3269284268010768657, 0.3333333333333333703, 0.3269284268010768657, 0.3333333333333333703, 0.3269284268010768657, 0.3333333333333333703, 0.3269284268010768657, 0.3333333333333333703, 0.3269284268010768657, 0.3333333333333333703, 0.3269284268010768657, 0.3333333333333333703, 0.3269284268010768657, 0.3333333333333333703, 0.3269284268010768657, 0.3333333333333333703, 0.3269284268010768657, 0.3333333333333333703, 0.3269284268010768657, 0.3333333333333333703, 0.3269284268010768657, 0.3333333333333333703, 0.3269284268010768657, 0.3333333333333333703, 0.3269284268010768657, 0.3333333333333333703, 0.3269284268010768657, 0.3333333333333333703, 0.3269284268010768657, 0.3333333333333333703, 0.3269284268010768657, 0.3333333333333333703, 0.3269284268010768657, 0.3333333333333333703, 0.3269284268010768657, 0.3333333333333333703, 0.3269284268010768657, 0.3333333333333333703, 0.3269284268010768657, 0.3333333333333333703, 0.3269284268010768657, 0.3333333333333333703, 0.3269284268010768657, 0.3333333333333333703, 0.3269284268010768657, 0.3333333333333333703, 0.3269284268010768657, 0.3333333333333333703, 0.3269284268010768657, 0.3333333333333333703, 0.3269284268010768657, 0.3333333333333333703, 0.3269284268010768657, 0.3333333333333333703, 0.3269284268010768657, 0.3333333333333333703, 0.3269284268010768657, 0.3333333333333333703, 0.3269284268010768657, 0.3333333333333333703, 0.3269284268010768657, 0.3333333333333333703, 0.3269284268010768657, 0.3333333333333333703, 0.3269284268010768657, 0.3333333333333333703, 0.3269284268010768657, 0.3333333333333333703, 0.3269284268010768657, 0.3333333333333333703, 0.3269284268010768657, 0.3333333333333333703, 0.3269284268010768657, 0.3333333333333333703, 0.3269284268010768657, 0.3333333333333333703, 0.3269284268010768657, 0.3333333333333333703, 0.3269284268010768657, 0.3333333333333333703, 0.3269284268010768657, 0.3333333333333333703, 0.3269284268010768657, 0.3333333333333333703, 0.3269284268010768657, 0.3333333333333333703, 0.3269284268010768657, 0.3333333333333333703, 0.3269284268010768657, 0.3333333333333333703, 0.3269284268010768657, 0.3333333333333333703, 0.3269284268010768657, 0.3333333333333333703, 0.3269284268010768657, 0.3333333333333333703, 0.3269284268010768657, 0.3333333333333333703, 0.3269284268010768657, 0.3333333333333333703, 0.3269284268010768657, 0.3333333333333333703, 0.3269284268010768657, 0.3333333333333333703, 0.3269284268010768657, 0.3333333333333333703, 0.3269284268010768657, 0.3333333333333333703, 0.3269284268010768657, 0.3333333333333333703, 0.3269284268010768657, 0.3333333333333333703, 0.3269284268010768657, 0.3333333333333333703, 0.3269284268010768657, 0.3333333333333333703, 0.3269284268010768657, 0.3333333333333333703, 0.3269284268010768657, 0.3333333333333333703, 0.3269284268010768657, 0.3333333333333333703, 0.3269284268010768657, 0.3333333333333333703, 0.3269284268010768657, 0.3333333333333333703, 0.3269284268010768657, 0.3333333333333333703, 0.3269284268010768657, 0.3333333333333333703, 0.3269284268010768657, 0.3333333333333333703, 0.3269284268010768657, 0.3333333333333333703, 0.3269284268010768657, 0.3333333333333333703, 0.3269284268010768657, 0.3333333333333333703, 0.3269284268010768657, 0.3333333333333333703, 0.3269284268010768657, 0.3333333333333333703, 0.3269284268010768657, 0.3333333333333333703, 0.3269284268010768657, 0.3333333333333333703, 0.3269284268010768657, 0.3333333333333333703, 0.3269284268010768657, 0.3333333333333333703, 0.3269284268010768657, 0.3333333333333333703, 0.3269284268010768657, 0.3333333333333333703, 0.3269284268010768657, 0.3333333333333333703, 0.3269284268010768657, 0.3333333333333333703, 0.3269284268010768657, 0.3333333333333333703, 0.3269284268010768657, 0.3333333333333333703, 0.3269284268010768657, 0.3333333333333333703, 0.3269284268010768657, 0.3333333333333333703, 0.3269284268010768657, 0.3333333333333333703, 0.3269284268010768657, 0.3333333333333333703, 0.3269284268010768657, 0.3333333333333333703, 0.3269284268010768657, 0.3333333333333333703, 0.3269284268010768657, 0.3333333333333333703, 0.3269284268010768657, 0.3333333333333333703, 0.3269284268010768657, 0.3333333333333333703, 0.3269284268010768657, 0.3333333333333333703, 0.3269284268010768657, 0.3333333333333333703, 0.3269284268010768657, 0.3333333333333333703, 0.3269284268010768657, 0.3333333333333333703, 0.3269284268010768657, 0.3333333333333333703, 0.3269284268010768657, 0.3333333333333333703, 0.3269284268010768657, 0.3333333333333333703, 0.3269284268010768657, 0.3333333333333333703, 0.3269284268010768657, 0.3333333333333333703, 0.3269284268010768657, 0.3333333333333333703, 0.3269284268010768657, 0.3333333333333333703, 0.3269284268010768657, 0.3333333333333333703, 0.3269284268010768657, 0.3333333333333333703, 0.3269284268010768657, 0.3333333333333333703, 0.3269284268010768657, 0.3333333333333333703, 0.3269284268010768657, 0.3333333333333333703, 0.3269284268010768657, 0.3333333333333333703, 0.3269284268010768657, 0.3333333333333333703, 0.3269284268010768657, 0.3333333333333333703, 0.3269284268010768657, 0.3333333333333333703, 0.3269284268010768657, 0.3333333333333333703, 0.3269284268010768657, 0.3333333333333333703, 0.3269284268010768657, 0.3333333333333333703, 0.3269284268010768657, 0.3333333333333333703, 0.3269284268010768657, 0.3333333333333333703, 0.3269284268010768657, 0.3333333333333333703, 0.3269284268010768657, 0.3333333333333333703, 0.3269284268010768657, 0.3333333333333333703),
 ( 0.3333333333333333703, 0.3269284268010768657, 0.3333333333333333703, 0.3269284268010768657, 0.3333333333333333703, 0.3269284268010768657, 0.3333333333333333703, 0.3269284268010768657, 0.3333333333333333703, 0.3269284268010768657, 0.3333333333333333703, 0.3269284268010768657, 0.3333333333333333703, 0.3269284268010768657, 0.3333333333333333703, 0.3269284268010768657, 0.3333333333333333703, 0.3269284268010768657, 0.3333333333333333703, 0.3269284268010768657, 0.3333333333333333703, 0.3269284268010768657, 0.3333333333333333703, 0.3269284268010768657, 0.3333333333333333703, 0.3269284268010768657, 0.3333333333333333703, 0.3269284268010768657, 0.3333333333333333703, 0.3269284268010768657, 0.3333333333333333703, 0.3269284268010768657, 0.3333333333333333703, 0.3269284268010768657, 0.3333333333333333703, 0.3269284268010768657, 0.3333333333333333703, 0.3269284268010768657, 0.3333333333333333703, 0.3269284268010768657, 0.3333333333333333703, 0.3269284268010768657, 0.3333333333333333703, 0.3269284268010768657, 0.3333333333333333703, 0.3269284268010768657, 0.3333333333333333703, 0.3269284268010768657, 0.3333333333333333703, 0.3269284268010768657, 0.3333333333333333703, 0.3269284268010768657, 0.3333333333333333703, 0.3269284268010768657, 0.3333333333333333703, 0.3269284268010768657, 0.3333333333333333703, 0.3269284268010768657, 0.3333333333333333703, 0.3269284268010768657, 0.3333333333333333703, 0.3269284268010768657, 0.3333333333333333703, 0.3269284268010768657, 0.3333333333333333703, 0.3269284268010768657, 0.3333333333333333703, 0.3269284268010768657, 0.3333333333333333703, 0.3269284268010768657, 0.3333333333333333703, 0.3269284268010768657, 0.3333333333333333703, 0.3269284268010768657, 0.3333333333333333703, 0.3269284268010768657, 0.3333333333333333703, 0.3269284268010768657, 0.3333333333333333703, 0.3269284268010768657, 0.3333333333333333703, 0.3269284268010768657, 0.3333333333333333703, 0.3269284268010768657, 0.3333333333333333703, 0.3269284268010768657, 0.3333333333333333703, 0.3269284268010768657, 0.3333333333333333703, 0.3269284268010768657, 0.3333333333333333703, 0.3269284268010768657, 0.3333333333333333703, 0.3269284268010768657, 0.3333333333333333703, 0.3269284268010768657, 0.3333333333333333703, 0.3269284268010768657, 0.3333333333333333703, 0.3269284268010768657, 0.3333333333333333703, 0.3269284268010768657, 0.3333333333333333703, 0.3269284268010768657, 0.3333333333333333703, 0.3269284268010768657, 0.3333333333333333703, 0.3269284268010768657, 0.3333333333333333703, 0.3269284268010768657, 0.3333333333333333703, 0.3269284268010768657, 0.3333333333333333703, 0.3269284268010768657, 0.3333333333333333703, 0.3269284268010768657, 0.3333333333333333703, 0.3269284268010768657, 0.3333333333333333703, 0.3269284268010768657, 0.3333333333333333703, 0.3269284268010768657, 0.3333333333333333703, 0.3269284268010768657, 0.3333333333333333703, 0.3269284268010768657, 0.3333333333333333703, 0.3269284268010768657, 0.3333333333333333703, 0.3269284268010768657, 0.3333333333333333703, 0.3269284268010768657, 0.3333333333333333703, 0.3269284268010768657, 0.3333333333333333703, 0.3269284268010768657, 0.3333333333333333703, 0.3269284268010768657, 0.3333333333333333703, 0.3269284268010768657, 0.3333333333333333703, 0.3269284268010768657, 0.3333333333333333703, 0.3269284268010768657, 0.3333333333333333703, 0.3269284268010768657, 0.3333333333333333703, 0.3269284268010768657, 0.3333333333333333703, 0.3269284268010768657, 0.3333333333333333703, 0.3269284268010768657, 0.3333333333333333703, 0.3269284268010768657, 0.3333333333333333703, 0.3269284268010768657, 0.3333333333333333703, 0.3269284268010768657, 0.3333333333333333703, 0.3269284268010768657, 0.3333333333333333703, 0.3269284268010768657, 0.3333333333333333703, 0.3269284268010768657, 0.3333333333333333703, 0.3269284268010768657, 0.3333333333333333703, 0.3269284268010768657, 0.3333333333333333703, 0.3269284268010768657, 0.3333333333333333703, 0.3269284268010768657, 0.3333333333333333703, 0.3269284268010768657, 0.3333333333333333703, 0.3269284268010768657, 0.3333333333333333703, 0.3269284268010768657, 0.3333333333333333703, 0.3269284268010768657, 0.3333333333333333703, 0.3269284268010768657, 0.3333333333333333703, 0.3269284268010768657, 0.3333333333333333703, 0.3269284268010768657, 0.3333333333333333703, 0.3269284268010768657, 0.3333333333333333703, 0.3269284268010768657, 0.3333333333333333703, 0.3269284268010768657, 0.3333333333333333703, 0.3269284268010768657, 0.3333333333333333703, 0.3269284268010768657, 0.3333333333333333703, 0.3269284268010768657, 0.3333333333333333703, 0.3269284268010768657, 0.3333333333333333703, 0.3269284268010768657, 0.3333333333333333703, 0.3269284268010768657, 0.3333333333333333703, 0.3269284268010768657, 0.3333333333333333703, 0.3269284268010768657, 0.3333333333333333703, 0.3269284268010768657, 0.3333333333333333703, 0.3269284268010768657, 0.3333333333333333703, 0.3269284268010768657, 0.3333333333333333703, 0.3269284268010768657, 0.3333333333333333703, 0.3269284268010768657, 0.3333333333333333703, 0.3269284268010768657, 0.3333333333333333703, 0.3269284268010768657, 0.3333333333333333703, 0.3269284268010768657, 0.3333333333333333703, 0.3269284268010768657, 0.3333333333333333703, 0.3269284268010768657, 0.3333333333333333703, 0.3269284268010768657, 0.3333333333333333703, 0.3269284268010768657, 0.3333333333333333703, 0.3269284268010768657, 0.3333333333333333703, 0.3269284268010768657, 0.3333333333333333703, 0.3269284268010768657, 0.3333333333333333703, 0.3269284268010768657, 0.3333333333333333703, 0.3269284268010768657, 0.3333333333333333703, 0.3269284268010768657, 0.3333333333333333703, 0.3269284268010768657, 0.3333333333333333703, 0.3269284268010768657, 0.3333333333333333703, 0.3269284268010768657, 0.3333333333333333703, 0.3269284268010768657, 0.3333333333333333703, 0.3269284268010768657, 0.3333333333333333703, 0.3269284268010768657, 0.3333333333333333703, 0.3269284268010768657, 0.3333333333333333703, 0.3269284268010768657, 0.3333333333333333703, 0.3269284268010768657, 0.3333333333333333703, 0.3269284268010768657, 0.3333333333333333703, 0.3269284268010768657, 0.3333333333333333703, 0.3269284268010768657, 0.3333333333333333703, 0.3269284268010768657, 0.3333333333333333703, 0.3269284268010768657, 0.3333333333333333703, 0.3269284268010768657, 0.3333333333333333703, 0.3269284268010768657, 0.3333333333333333703, 0.3269284268010768657, 0.3333333333333333703, 0.3269284268010768657, 0.3333333333333333703, 0.3269284268010768657, 0.3333333333333333703, 0.3269284268010768657, 0.3333333333333333703, 0.3269284268010768657, 0.3333333333333333703, 0.3269284268010768657, 0.3333333333333333703, 0.3269284268010768657, 0.3333333333333333703, 0.3269284268010768657, 0.3333333333333333703, 0.3269284268010768657, 0.3333333333333333703, 0.3269284268010768657, 0.3333333333333333703, 0.3269284268010768657, 0.3333333333333333703, 0.3269284268010768657, 0.3333333333333333703, 0.3269284268010768657, 0.3333333333333333703, 0.3269284268010768657, 0.3333333333333333703, 0.3269284268010768657, 0.3333333333333333703, 0.3269284268010768657, 0.3333333333333333703, 0.3269284268010768657, 0.3333333333333333703, 0.3269284268010768657, 0.3333333333333333703, 0.3269284268010768657, 0.3333333333333333703, 0.3269284268010768657, 0.3333333333333333703, 0.3269284268010768657, 0.3333333333333333703, 0.3269284268010768657, 0.3333333333333333703, 0.3269284268010768657, 0.3333333333333333703, 0.3269284268010768657, 0.3333333333333333703, 0.3269284268010768657, 0.3333333333333333703, 0.3269284268010768657, 0.3333333333333333703, 0.3269284268010768657, 0.3333333333333333703, 0.3269284268010768657, 0.3333333333333333703, 0.3269284268010768657, 0.3333333333333333703, 0.3269284268010768657, 0.3333333333333333703, 0.3269284268010768657, 0.3333333333333333703, 0.3269284268010768657, 0.3333333333333333703, 0.3269284268010768657, 0.3333333333333333703, 0.3269284268010768657, 0.3333333333333333703, 0.3269284268010768657, 0.3333333333333333703, 0.3269284268010768657, 0.3333333333333333703, 0.3269284268010768657, 0.3333333333333333703, 0.3269284268010768657, 0.3333333333333333703, 0.3269284268010768657, 0.3333333333333333703, 0.3269284268010768657, 0.3333333333333333703, 0.3269284268010768657, 0.3333333333333333703, 0.3269284268010768657, 0.3333333333333333703, 0.3269284268010768657, 0.3333333333333333703, 0.3269284268010768657, 0.3333333333333333703, 0.3269284268010768657, 0.3333333333333333703, 0.3269284268010768657, 0.3333333333333333703, 0.3269284268010768657, 0.3333333333333333703, 0.3269284268010768657, 0.3333333333333333703, 0.3269284268010768657, 0.3333333333333333703, 0.3269284268010768657, 0.3333333333333333703, 0.3269284268010768657, 0.3333333333333333703, 0.3269284268010768657, 0.3333333333333333703, 0.3269284268010768657, 0.3333333333333333703, 0.3269284268010768657, 0.3333333333333333703, 0.3269284268010768657, 0.3333333333333333703, 0.3269284268010768657, 0.3333333333333333703, 0.3269284268010768657, 0.3333333333333333703, 0.3269284268010768657, 0.3333333333333333703, 0.3269284268010768657, 0.3333333333333333703, 0.3269284268010768657, 0.3333333333333333703, 0.3269284268010768657, 0.3333333333333333703, 0.3269284268010768657, 0.3333333333333333703, 0.3269284268010768657, 0.3333333333333333703, 0.3269284268010768657, 0.3333333333333333703, 0.3269284268010768657, 0.3333333333333333703, 0.3269284268010768657, 0.3333333333333333703, 0.3269284268010768657, 0.3333333333333333703, 0.3269284268010768657, 0.3333333333333333703, 0.3269284268010768657, 0.3333333333333333703, 0.3269284268010768657, 0.3333333333333333703, 0.3269284268010768657, 0.3333333333333333703, 0.3269284268010768657, 0.3333333333333333703, 0.3269284268010768657, 0.3333333333333333703, 0.3269284268010768657, 0.3333333333333333703, 0.3269284268010768657, 0.3333333333333333703, 0.3269284268010768657, 0.3333333333333333703, 0.3269284268010768657, 0.3333333333333333703, 0.3269284268010768657, 0.3333333333333333703, 0.3269284268010768657, 0.3333333333333333703, 0.3269284268010768657, 0.3333333333333333703, 0.3269284268010768657, 0.3333333333333333703, 0.3269284268010768657, 0.3333333333333333703, 0.3269284268010768657, 0.3333333333333333703, 0.3269284268010768657, 0.3333333333333333703, 0.3269284268010768657, 0.3333333333333333703, 0.3269284268010768657, 0.3333333333333333703, 0.3269284268010768657, 0.3333333333333333703, 0.3269284268010768657, 0.3333333333333333703, 0.3269284268010768657, 0.3333333333333333703, 0.3269284268010768657, 0.3333333333333333703, 0.3269284268010768657, 0.3333333333333333703, 0.3269284268010768657, 0.3333333333333333703, 0.3269284268010768657, 0.3333333333333333703, 0.3269284268010768657, 0.3333333333333333703, 0.3269284268010768657, 0.3333333333333333703, 0.3269284268010768657, 0.3333333333333333703, 0.3269284268010768657, 0.3333333333333333703, 0.3269284268010768657, 0.3333333333333333703, 0.3269284268010768657, 0.3333333333333333703, 0.3269284268010768657, 0.3333333333333333703, 0.3269284268010768657, 0.3333333333333333703, 0.3269284268010768657, 0.3333333333333333703),
 ( 1.000000000000000000, 0.9807852804032304306, 1.000000000000000000, 0.9807852804032304306, 1.000000000000000000, 0.9807852804032304306, 1.000000000000000000, 0.9807852804032304306, 1.000000000000000000, 0.9807852804032304306, 1.000000000000000000, 0.9807852804032304306, 1.000000000000000000, 0.9807852804032304306, 1.000000000000000000, 0.9807852804032304306, 1.000000000000000000, 0.9807852804032304306, 1.000000000000000000, 0.9807852804032304306, 1.000000000000000000, 0.9807852804032304306, 1.000000000000000000, 0.9807852804032304306, 1.000000000000000000, 0.9807852804032304306, 1.000000000000000000, 0.9807852804032304306, 1.000000000000000000, 0.9807852804032304306, 1.000000000000000000, 0.9807852804032304306, 1.000000000000000000, 0.9807852804032304306, 1.000000000000000000, 0.9807852804032304306, 1.000000000000000000, 0.9807852804032304306, 1.000000000000000000, 0.9807852804032304306, 1.000000000000000000, 0.9807852804032304306, 1.000000000000000000, 0.9807852804032304306, 1.000000000000000000, 0.9807852804032304306, 1.000000000000000000, 0.9807852804032304306, 1.000000000000000000, 0.9807852804032304306, 1.000000000000000000, 0.9807852804032304306, 1.000000000000000000, 0.9807852804032304306, 1.000000000000000000, 0.9807852804032304306, 1.000000000000000000, 0.9807852804032304306, 1.000000000000000000, 0.9807852804032304306, 1.000000000000000000, 0.9807852804032304306, 1.000000000000000000, 0.9807852804032304306, 1.000000000000000000, 0.9807852804032304306, 1.000000000000000000, 0.9807852804032304306, 1.000000000000000000, 0.9807852804032304306, 1.000000000000000000, 0.9807852804032304306, 1.000000000000000000, 0.9807852804032304306, 1.000000000000000000, 0.9807852804032304306, 1.000000000000000000, 0.9807852804032304306, 1.000000000000000000, 0.9807852804032304306, 1.000000000000000000, 0.9807852804032304306, 1.000000000000000000, 0.9807852804032304306, 1.000000000000000000, 0.9807852804032304306, 1.000000000000000000, 0.9807852804032304306, 1.000000000000000000, 0.9807852804032304306, 1.000000000000000000, 0.9807852804032304306, 1.000000000000000000, 0.9807852804032304306, 1.000000000000000000, 0.9807852804032304306, 1.000000000000000000, 0.9807852804032304306, 1.000000000000000000, 0.9807852804032304306, 1.000000000000000000, 0.9807852804032304306, 1.000000000000000000, 0.9807852804032304306, 1.000000000000000000, 0.9807852804032304306, 1.000000000000000000, 0.9807852804032304306, 1.000000000000000000, 0.9807852804032304306, 1.000000000000000000, 0.9807852804032304306, 1.000000000000000000, 0.9807852804032304306, 1.000000000000000000, 0.9807852804032304306, 1.000000000000000000, 0.9807852804032304306, 1.000000000000000000, 0.9807852804032304306, 1.000000000000000000, 0.9807852804032304306, 1.000000000000000000, 0.9807852804032304306, 1.000000000000000000, 0.9807852804032304306, 1.000000000000000000, 0.9807852804032304306, 1.000000000000000000, 0.9807852804032304306, 1.000000000000000000, 0.9807852804032304306, 1.000000000000000000, 0.9807852804032304306, 1.000000000000000000, 0.9807852804032304306, 1.000000000000000000, 0.9807852804032304306, 1.000000000000000000, 0.9807852804032304306, 1.000000000000000000, 0.9807852804032304306, 1.000000000000000000, 0.9807852804032304306, 1.000000000000000000, 0.9807852804032304306, 1.000000000000000000, 0.9807852804032304306, 1.000000000000000000, 0.9807852804032304306, 1.000000000000000000, 0.9807852804032304306, 1.000000000000000000, 0.9807852804032304306, 1.000000000000000000, 0.9807852804032304306, 1.000000000000000000, 0.9807852804032304306, 1.000000000000000000, 0.9807852804032304306, 1.000000000000000000, 0.9807852804032304306, 1.000000000000000000, 0.9807852804032304306, 1.000000000000000000, 0.9807852804032304306, 1.000000000000000000, 0.9807852804032304306, 1.000000000000000000, 0.9807852804032304306, 1.000000000000000000, 0.9807852804032304306, 1.000000000000000000, 0.9807852804032304306, 1.000000000000000000, 0.9807852804032304306, 1.000000000000000000, 0.9807852804032304306, 1.000000000000000000, 0.9807852804032304306, 1.000000000000000000, 0.9807852804032304306, 1.000000000000000000, 0.9807852804032304306, 1.000000000000000000, 0.9807852804032304306, 1.000000000000000000, 0.9807852804032304306, 1.000000000000000000, 0.9807852804032304306, 1.000000000000000000, 0.9807852804032304306, 1.000000000000000000, 0.9807852804032304306, 1.000000000000000000, 0.9807852804032304306, 1.000000000000000000, 0.9807852804032304306, 1.000000000000000000, 0.9807852804032304306, 1.000000000000000000, 0.9807852804032304306, 1.000000000000000000, 0.9807852804032304306, 1.000000000000000000, 0.9807852804032304306, 1.000000000000000000, 0.9807852804032304306, 1.000000000000000000, 0.9807852804032304306, 1.000000000000000000, 0.9807852804032304306, 1.000000000000000000, 0.9807852804032304306, 1.000000000000000000, 0.9807852804032304306, 1.000000000000000000, 0.9807852804032304306, 1.000000000000000000, 0.9807852804032304306, 1.000000000000000000, 0.9807852804032304306, 1.000000000000000000, 0.9807852804032304306, 1.000000000000000000, 0.9807852804032304306, 1.000000000000000000, 0.9807852804032304306, 1.000000000000000000, 0.9807852804032304306, 1.000000000000000000, 0.9807852804032304306, 1.000000000000000000, 0.9807852804032304306, 1.000000000000000000, 0.9807852804032304306, 1.000000000000000000, 0.9807852804032304306, 1.000000000000000000, 0.9807852804032304306, 1.000000000000000000, 0.9807852804032304306, 1.000000000000000000, 0.9807852804032304306, 1.000000000000000000, 0.9807852804032304306, 1.000000000000000000, 0.9807852804032304306, 1.000000000000000000, 0.9807852804032304306, 1.000000000000000000, 0.9807852804032304306, 1.000000000000000000, 0.9807852804032304306, 1.000000000000000000, 0.9807852804032304306, 1.000000000000000000, 0.9807852804032304306, 1.000000000000000000, 0.9807852804032304306, 1.000000000000000000, 0.9807852804032304306, 1.000000000000000000, 0.9807852804032304306, 1.000000000000000000, 0.9807852804032304306, 1.000000000000000000, 0.9807852804032304306, 1.000000000000000000, 0.9807852804032304306, 1.000000000000000000, 0.9807852804032304306, 1.000000000000000000, 0.9807852804032304306, 1.000000000000000000, 0.9807852804032304306, 1.000000000000000000, 0.9807852804032304306, 1.000000000000000000, 0.9807852804032304306, 1.000000000000000000, 0.9807852804032304306, 1.000000000000000000, 0.9807852804032304306, 1.000000000000000000, 0.9807852804032304306, 1.000000000000000000, 0.9807852804032304306, 1.000000000000000000, 0.9807852804032304306, 1.000000000000000000, 0.9807852804032304306, 1.000000000000000000, 0.9807852804032304306, 1.000000000000000000, 0.9807852804032304306, 1.000000000000000000, 0.9807852804032304306, 1.000000000000000000, 0.9807852804032304306, 1.000000000000000000, 0.9807852804032304306, 1.000000000000000000, 0.9807852804032304306, 1.000000000000000000, 0.9807852804032304306, 1.000000000000000000, 0.9807852804032304306, 1.000000000000000000, 0.9807852804032304306, 1.000000000000000000, 0.9807852804032304306, 1.000000000000000000, 0.9807852804032304306, 1.000000000000000000, 0.9807852804032304306, 1.000000000000000000, 0.9807852804032304306, 1.000000000000000000, 0.9807852804032304306, 1.000000000000000000, 0.9807852804032304306, 1.000000000000000000, 0.9807852804032304306, 1.000000000000000000, 0.9807852804032304306, 1.000000000000000000, 0.9807852804032304306, 1.000000000000000000, 0.9807852804032304306, 1.000000000000000000, 0.9807852804032304306, 1.000000000000000000, 0.9807852804032304306, 1.000000000000000000, 0.9807852804032304306, 1.000000000000000000, 0.9807852804032304306, 1.000000000000000000, 0.9807852804032304306, 1.000000000000000000, 0.9807852804032304306, 1.000000000000000000, 0.9807852804032304306, 1.000000000000000000, 0.9807852804032304306, 1.000000000000000000, 0.9807852804032304306, 1.000000000000000000, 0.9807852804032304306, 1.000000000000000000, 0.9807852804032304306, 1.000000000000000000, 0.9807852804032304306, 1.000000000000000000, 0.9807852804032304306, 1.000000000000000000, 0.9807852804032304306, 1.000000000000000000, 0.9807852804032304306, 1.000000000000000000, 0.9807852804032304306, 1.000000000000000000, 0.9807852804032304306, 1.000000000000000000, 0.9807852804032304306, 1.000000000000000000, 0.9807852804032304306, 1.000000000000000000, 0.9807852804032304306, 1.000000000000000000, 0.9807852804032304306, 1.000000000000000000, 0.9807852804032304306, 1.000000000000000000, 0.9807852804032304306, 1.000000000000000000, 0.9807852804032304306, 1.000000000000000000, 0.9807852804032304306, 1.000000000000000000, 0.9807852804032304306, 1.000000000000000000, 0.9807852804032304306, 1.000000000000000000, 0.9807852804032304306, 1.000000000000000000, 0.9807852804032304306, 1.000000000000000000, 0.9807852804032304306, 1.000000000000000000, 0.9807852804032304306, 1.000000000000000000, 0.9807852804032304306, 1.000000000000000000, 0.9807852804032304306, 1.000000000000000000, 0.9807852804032304306, 1.000000000000000000, 0.9807852804032304306, 1.000000000000000000, 0.9807852804032304306, 1.000000000000000000, 0.9807852804032304306, 1.000000000000000000, 0.9807852804032304306, 1.000000000000000000, 0.9807852804032304306, 1.000000000000000000, 0.9807852804032304306, 1.000000000000000000, 0.9807852804032304306, 1.000000000000000000, 0.9807852804032304306, 1.000000000000000000, 0.9807852804032304306, 1.000000000000000000, 0.9807852804032304306, 1.000000000000000000, 0.9807852804032304306, 1.000000000000000000, 0.9807852804032304306, 1.000000000000000000, 0.9807852804032304306, 1.000000000000000000, 0.9807852804032304306, 1.000000000000000000, 0.9807852804032304306, 1.000000000000000000, 0.9807852804032304306, 1.000000000000000000, 0.9807852804032304306, 1.000000000000000000, 0.9807852804032304306, 1.000000000000000000, 0.9807852804032304306, 1.000000000000000000, 0.9807852804032304306, 1.000000000000000000, 0.9807852804032304306, 1.000000000000000000, 0.9807852804032304306, 1.000000000000000000, 0.9807852804032304306, 1.000000000000000000, 0.9807852804032304306, 1.000000000000000000, 0.9807852804032304306, 1.000000000000000000, 0.9807852804032304306, 1.000000000000000000, 0.9807852804032304306, 1.000000000000000000, 0.9807852804032304306, 1.000000000000000000, 0.9807852804032304306, 1.000000000000000000, 0.9807852804032304306, 1.000000000000000000, 0.9807852804032304306, 1.000000000000000000, 0.9807852804032304306, 1.000000000000000000, 0.9807852804032304306, 1.000000000000000000, 0.9807852804032304306, 1.000000000000000000, 0.9807852804032304306, 1.000000000000000000, 0.9807852804032304306, 1.000000000000000000, 0.9807852804032304306, 1.000000000000000000, 0.9807852804032304306, 1.000000000000000000, 0.9807852804032304306, 1.000000000000000000, 0.9807852804032304306, 1.000000000000000000, 0.9807852804032304306, 1.000000000000000000) ) ) 
 REPRESENTATION_ITEM ( '' )  SURFACE ( )  );
#297=CARTESIAN_POINT ( 'NONE',  ( 8.962234695871762469, 62.16018628210144215, -8.715434833791931624 ) ) ;
#304=CARTESIAN_POINT ( 'NONE',  ( 13.04141134922778988, 47.02731371789855075, -8.927990412390371944 ) ) ;
#310=CARTESIAN_POINT ( 'NONE',  ( 9.534712964251900402, 20.57731371789854435, 1.715153634034445540 ) ) ;
#318=CARTESIAN_POINT ( 'NONE',  ( 5.770363421894130873, 128.9648137178985792, -14.38691631536193860 ) ) ;
#320=CARTESIAN_POINT ( 'NONE',  ( -0.1745138560725500443, 47.21018628210143930, 12.50000000000000355 ) ) ;
#329=CARTESIAN_POINT ( 'NONE',  ( 3.796722387233379514, 52.38518628210145778, -8.710071997420127943 ) ) ;
#332=CARTESIAN_POINT ( 'NONE',  ( -2.660918448318275509, 93.49768628210145494, 12.46528703574805874 ) ) ;
#345=CARTESIAN_POINT ( 'NONE',  ( -7.228626920338836470, 127.5273137178985792, -10.49813415416005213 ) ) ;
#347=CARTESIAN_POINT ( 'NONE',  ( 0.1745138560725515708, 116.2101862821014606, -12.50000000000000355 ) ) ;
#353=CARTESIAN_POINT ( 'NONE',  ( 6.092822981423662299, 86.41481371789855359, 14.25334919248795096 ) ) ;
#358=CARTESIAN_POINT ( 'NONE',  ( 8.710071997420211432, 84.11481371789855643, -3.796722387233181895 ) ) ;
#361=CARTESIAN_POINT ( 'NONE',  ( 4.944772684328420986, 40.41481371789855359, 11.48171059495408208 ) ) ;
#363=CARTESIAN_POINT ( 'NONE',  ( 4.944772684328679446, 107.5851862821014464, -11.48171059495397373 ) ) ;
#366=CARTESIAN_POINT ( 'NONE',  ( -8.962234695871760692, 140.3601862821014379, 8.715434833791933400 ) ) ;
#368=CARTESIAN_POINT ( 'NONE',  ( 11.08355503943142750, 80.56018628210146915, -10.83675517735155225 ) ) ;
#372=CARTESIAN_POINT ( 'NONE',  ( -8.843639120294326972, 113.3351862821014606, 3.474262827703335166 ) ) ;
#374=CARTESIAN_POINT ( 'NONE',  ( -11.08355503943142573, 11.56018628210145316, 10.83675517735155402 ) ) ;
#379=CARTESIAN_POINT ( 'NONE',  ( 2.064181346179272847, 52.09768628210144925, -9.465287035748065847 ) ) ;
#387=CARTESIAN_POINT ( 'NONE',  ( 1.715153634034445762, 45.87731371789854506, -9.534712964251895073 ) ) ;
#391=CARTESIAN_POINT ( 'NONE',  ( 12.53471296425189330, 48.17731371789854222, 2.311890736173451533 ) ) ;
#393=CARTESIAN_POINT ( 'NONE',  ( 4.944772684328420986, 12.81481371789855395, 11.48171059495408208 ) ) ;
#409=CARTESIAN_POINT ( 'NONE',  ( 15.53471296425188797, 29.77731371789854364, 2.908627838312457747 ) ) ;
#411=CARTESIAN_POINT ( 'NONE',  ( 9.500000000000005329, 127.7101862821014606, 0.1745138560725188748 ) ) ;
#413=CARTESIAN_POINT ( 'NONE',  ( 8.715434833791931624, 27.66018628210144215, 8.962234695871760692 ) ) ;
#419=CARTESIAN_POINT ( 'NONE',  ( 2.064181346179272847, 15.29768628210142722, -9.465287035748065847 ) ) ;
#427=CARTESIAN_POINT ( 'NONE',  ( 2.064181346179061460, 86.70231371789851949, 9.465287035748106703 ) ) ;
#433=CARTESIAN_POINT ( 'NONE',  ( 7.228626920338837358, 95.32731371789856212, 10.49813415416005036 ) ) ;
#437=CARTESIAN_POINT ( 'NONE',  ( -4.944772684328424539, 63.41481371789856070, -11.48171059495408031 ) ) ;
#444=CARTESIAN_POINT ( 'NONE',  ( 4.944772684328679446, 43.18518628210144072, -11.48171059495397373 ) ) ;
#449=CARTESIAN_POINT ( 'NONE',  ( -11.48171059495408208, 107.1148137178985564, 4.944772684328421875 ) ) ;
#454=CARTESIAN_POINT ( 'NONE',  ( -14.38691631536193860, 71.46481371789856496, -5.770363421894132649 ) ) ;
#458=CARTESIAN_POINT ( 'NONE',  ( 11.48171059495397728, 109.8851862821014436, 4.944772684328674117 ) ) ;
#459=CARTESIAN_POINT ( 'NONE',  ( -15.53471296425195369, 49.22268628210144215, 2.908627838312118019 ) ) ;
#463=CARTESIAN_POINT ( 'NONE',  ( 15.53471296425195369, 63.02268628210144641, -2.908627838312120684 ) ) ;
#469=CARTESIAN_POINT ( 'NONE',  ( 2.660918448318279950, 42.89768628210143930, -12.46528703574805697 ) ) ;
#471=CARTESIAN_POINT ( 'NONE',  ( -3.474262827703337830, 5.235186282101429001, -8.843639120294326972 ) ) ;
#482=CARTESIAN_POINT ( 'NONE',  ( -2.311890736173176641, 42.32268628210145067, -12.53471296425194659 ) ) ;
#490=CARTESIAN_POINT ( 'NONE',  ( 4.622313124798573369, 101.8351862821014464, 11.61527771782819940 ) ) ;
#491=CARTESIAN_POINT ( 'NONE',  ( -8.927990412390371944, 17.12731371789855217, -13.04141134922778988 ) ) ;
#497=CARTESIAN_POINT ( 'NONE',  ( -9.500000000000005329, 15.68981371789854329, 0.1745138560723101806 ) ) ;
#503=CARTESIAN_POINT ( 'NONE',  ( -0.1745138560722442889, 128.3898137178985621, -15.50000000000000533 ) ) ;
#506=CARTESIAN_POINT ( 'NONE',  ( -10.49813415415989581, 50.37268628210145494, -7.228626920339068285 ) ) ;
#512=CARTESIAN_POINT ( 'NONE',  ( 5.233372021372432847, 64.74768628210144072, 8.152565276336710909 ) ) ;
#515=CARTESIAN_POINT ( 'NONE',  ( -10.49813415415989581, 87.17268628210143788, -7.228626920339068285 ) ) ;
#527=CARTESIAN_POINT ( 'NONE',  ( 8.715434833792128799, 101.9398137178985593, -8.962234695871567070 ) ) ;
#528=CARTESIAN_POINT ( 'NONE',  ( 7.228626920339069173, 126.2726862821014322, -10.49813415415989404 ) ) ;
#533=CARTESIAN_POINT ( 'NONE',  ( 15.46528703574811736, 84.40231371789855075, -3.257655550456947768 ) ) ;
#538=CARTESIAN_POINT ( 'NONE',  ( -6.840914352312096547, 94.36018628210146630, 6.594114490232313663 ) ) ;
#540=CARTESIAN_POINT ( 'NONE',  ( 9.465287035748106703, 75.20231371789854791, -2.064181346179063237 ) ) ;
#543=CARTESIAN_POINT ( 'NONE',  ( 8.715434833792128799, 46.73981371789854933, -8.962234695871567070 ) ) ;
#545=CARTESIAN_POINT ( 'NONE',  ( 8.962234695871762469, 108.1601862821014635, -8.715434833791931624 ) ) ;
#551=CARTESIAN_POINT ( 'NONE',  ( -15.53471296425195369, 76.82268628210144357, 2.908627838312118019 ) ) ;
#555=CARTESIAN_POINT ( 'NONE',  ( -1.715153634034234598, 106.7226862821014635, -9.534712964251941258 ) ) ;
#558=CARTESIAN_POINT ( 'NONE',  ( -15.50000000000000533, 12.71018628210143753, -0.1745138560725808530 ) ) ;
#569=CARTESIAN_POINT ( 'NONE',  ( -8.152565276336593669, 16.55231371789855643, -5.233372021372610483 ) ) ;
#573=CARTESIAN_POINT ( 'NONE',  ( 10.49813415416005213, 47.02731371789855075, -7.228626920338837358 ) ) ;
#575=CARTESIAN_POINT ( 'NONE',  ( -8.962234695871565293, 7.639813717898541690, -8.715434833792128799 ) ) ;
#592=CARTESIAN_POINT ( 'NONE',  ( -8.927990412390371944, 7.927313717898536005, -13.04141134922778988 ) ) ;
#595=CARTESIAN_POINT ( 'NONE',  ( -8.843639120294326972, 131.7351862821014663, 3.474262827703335166 ) ) ;
#597=CARTESIAN_POINT ( 'NONE',  ( -12.53471296425194836, 30.82268628210144001, 2.311890736173176641 ) ) ;
#601=CARTESIAN_POINT ( 'NONE',  ( -8.632099005475501130, 124.5476862821014663, -13.23911966647218996 ) ) ;
#603=CARTESIAN_POINT ( 'NONE',  ( 9.500000000000005329, 139.8898137178985621, -0.1745138560723090149 ) ) ;
#610=CARTESIAN_POINT ( 'NONE',  ( -9.465287035748106703, 98.20231371789854791, 2.064181346179061460 ) ) ;
#612=ORIENTED_EDGE ( 'NONE', *, *, #9923, .T. ) ;
#615=CARTESIAN_POINT ( 'NONE',  ( -2.311890736173447980, 105.6773137178985706, 12.53471296425189330 ) ) ;
#620=CARTESIAN_POINT ( 'NONE',  ( 4.622313124798831829, 73.76481371789856212, -11.61527771782809282 ) ) ;
#628=CARTESIAN_POINT ( 'NONE',  ( -2.660918448318275509, 38.29768628210145920, 12.46528703574805874 ) ) ;
#634=CARTESIAN_POINT ( 'NONE',  ( 7.228626920338837358, 76.92731371789857064, 10.49813415416005036 ) ) ;
#640=CARTESIAN_POINT ( 'NONE',  ( -13.04141134922778456, 60.82731371789854080, 8.927990412390377273 ) ) ;
#643=CARTESIAN_POINT ( 'NONE',  ( -4.622313124798576922, 88.03518628210144925, -11.61527771782819762 ) ) ;
#644=CARTESIAN_POINT ( 'NONE',  ( -13.04141134922759804, 41.17268628210143078, -8.927990412390657937 ) ) ;
#648=CARTESIAN_POINT ( 'NONE',  ( -14.25334919248782306, 50.08518628210143930, -6.092822981423979378 ) ) ;
#654=CARTESIAN_POINT ( 'NONE',  ( 10.69584247140445221, 16.44768628210144001, -6.932735513423970097 ) ) ;
#655=CARTESIAN_POINT ( 'NONE',  ( 2.064181346179061460, 141.9023137178985507, 9.465287035748106703 ) ) ;
#666=CARTESIAN_POINT ( 'NONE',  ( 12.53471296425194659, 44.62268628210144783, -2.311890736173178418 ) ) ;
#674=CARTESIAN_POINT ( 'NONE',  ( -7.228626920339069173, 103.2726862821014606, 10.49813415415989581 ) ) ;
#675=CARTESIAN_POINT ( 'NONE',  ( 13.23911966647199812, 11.95231371789853902, 8.632099005475788900 ) ) ;
#683=CARTESIAN_POINT ( 'NONE',  ( -8.843639120294245259, 7.064813717898548617, -3.474262827703533230 ) ) ;
#689=CARTESIAN_POINT ( 'NONE',  ( -3.257655550456946880, 128.1023137178985678, -15.46528703574811736 ) ) ;
#692=CARTESIAN_POINT ( 'NONE',  ( 0.1745138560725515708, 42.61018628210144499, -12.50000000000000355 ) ) ;
#696=CARTESIAN_POINT ( 'NONE',  ( -15.53471296425195369, 95.22268628210143504, 2.908627838312118019 ) ) ;
#699=CARTESIAN_POINT ( 'NONE',  ( 9.534712964251941258, 53.82268628210144357, -1.715153634034235708 ) ) ;
#702=CARTESIAN_POINT ( 'NONE',  ( -4.944772684328673229, 93.78518628210144925, 11.48171059495397728 ) ) ;
#715=CARTESIAN_POINT ( 'NONE',  ( -8.715434833792127023, 106.5398137178985536, 8.962234695871568846 ) ) ;
#716=CARTESIAN_POINT ( 'NONE',  ( 4.944772684328679446, 107.5851862821014464, -11.48171059495397373 ) ) ;
#720=CARTESIAN_POINT ( 'NONE',  ( -15.46528703574811736, 70.60231371789853938, 3.257655550456946436 ) ) ;
#723=CARTESIAN_POINT ( 'NONE',  ( 7.954856959092191815, 91.77268628210144641, 5.529263428287477744 ) ) ;
#726=CARTESIAN_POINT ( 'NONE',  ( 3.474262827703532341, 82.96481371789856496, -8.843639120294245259 ) ) ;
#729=CARTESIAN_POINT ( 'NONE',  ( -8.710071997420207879, 107.1148137178985564, 3.796722387233182339 ) ) ;
#731=CARTESIAN_POINT ( 'NONE',  ( -11.48171059495408208, 51.91481371789855359, 4.944772684328421875 ) ) ;
#734=CARTESIAN_POINT ( 'NONE',  ( 8.962234695871762469, 98.96018628210146062, -8.715434833791931624 ) ) ;
#737=CARTESIAN_POINT ( 'NONE',  ( 7.228626920339068285, 135.4726862821014493, -10.49813415415989581 ) ) ;
#739=CARTESIAN_POINT ( 'NONE',  ( 8.632099005475504683, 73.94768628210142936, 13.23911966647218996 ) ) ;
#744=CARTESIAN_POINT ( 'NONE',  ( 0.1745138560725194299, 116.2101862821014748, -9.500000000000005329 ) ) ;
#747=CARTESIAN_POINT ( 'NONE',  ( -2.908627838312119351, 5.522686282101450850, -15.53471296425195369 ) ) ;
#760=CARTESIAN_POINT ( 'NONE',  ( -8.843639120294245259, 25.46481371789855075, -3.474262827703533230 ) ) ;
#765=CARTESIAN_POINT ( 'NONE',  ( 10.69584247140429589, 30.35231371789855359, 6.932735513424201024 ) ) ;
#767=CARTESIAN_POINT ( 'NONE',  ( -13.23911966647199812, 126.9523137178985621, -8.632099005475788900 ) ) ;
#785=CARTESIAN_POINT ( 'NONE',  ( -11.08355503943142573, 140.3601862821014663, 10.83675517735155402 ) ) ;
#787=CARTESIAN_POINT ( 'NONE',  ( 5.529263428287477744, 126.2726862821014464, -7.954856959092191815 ) ) ;
#789=CARTESIAN_POINT ( 'NONE',  ( 10.69584247140445221, 34.84768628210143504, -6.932735513423970097 ) ) ;
#794=CARTESIAN_POINT ( 'NONE',  ( 15.46528703574804986, 118.7976862821014521, 3.257655550457285720 ) ) ;
#797=CARTESIAN_POINT ( 'NONE',  ( 8.710071997420211432, 139.3148137178985451, -3.796722387233181895 ) ) ;
#803=CARTESIAN_POINT ( 'NONE',  ( 9.500000000000005329, 75.48981371789854222, -0.1745138560723090149 ) ) ;
#807=CARTESIAN_POINT ( 'NONE',  ( 0.1745138560722779009, 96.18981371789855928, 12.50000000000000355 ) ) ;
#811=CARTESIAN_POINT ( 'NONE',  ( 12.46528703574811558, 56.80231371789856354, -2.660918448318005503 ) ) ;
#820=CARTESIAN_POINT ( 'NONE',  ( -12.46528703574805697, 40.59768628210144215, -2.660918448318280838 ) ) ;
#825=STYLED_ITEM ( 'NONE', ( #26368 ), #18760 ) ;
#827=CARTESIAN_POINT ( 'NONE',  ( -4.944772684328424539, 91.01481371789856212, -11.48171059495408031 ) ) ;
#832=CARTESIAN_POINT ( 'NONE',  ( 15.46528703574811736, 56.80231371789854933, -3.257655550456947768 ) ) ;
#835=CARTESIAN_POINT ( 'NONE',  ( -11.48171059495397373, 86.88518628210145778, -4.944772684328680334 ) ) ;
#836=CARTESIAN_POINT ( 'NONE',  ( 8.632099005475504683, 27.94768628210144001, 13.23911966647218996 ) ) ;
#839=CARTESIAN_POINT ( 'NONE',  ( -15.50000000000000533, 49.51018628210145067, -0.1745138560725808530 ) ) ;
#844=CARTESIAN_POINT ( 'NONE',  ( -6.932735513423968321, 14.14768628210144463, -10.69584247140445221 ) ) ;
#846=CARTESIAN_POINT ( 'NONE',  ( 9.534712964251900402, 121.7773137178985650, 1.715153634034445540 ) ) ;
#859=CARTESIAN_POINT ( 'NONE',  ( 4.622313124798573369, 55.83518628210144641, 11.61527771782819940 ) ) ;
#866=CARTESIAN_POINT ( 'NONE',  ( 10.49813415415989581, 100.9726862821014635, 7.228626920339068285 ) ) ;
#867=CARTESIAN_POINT ( 'NONE',  ( -5.770363421894122880, 23.16481371789855359, 14.38691631536194393 ) ) ;
#874=CARTESIAN_POINT ( 'NONE',  ( 5.233372021372610483, 9.652313717898541867, -8.152565276336593669 ) ) ;
#880=CARTESIAN_POINT ( 'NONE',  ( -8.632099005475794229, 115.4523137178985479, 13.23911966647199812 ) ) ;
#883=CARTESIAN_POINT ( 'NONE',  ( 12.53471296425194836, 35.42268628210144499, -2.311890736173178418 ) ) ;
#887=CARTESIAN_POINT ( 'NONE',  ( -15.50000000000000533, 104.7101862821014606, -0.1745138560725808530 ) ) ;
#891=CARTESIAN_POINT ( 'NONE',  ( 9.500000000000005329, 63.31018628210144783, 0.1745138560725188748 ) ) ;
#895=CARTESIAN_POINT ( 'NONE',  ( -2.660918448318275509, 75.09768628210143504, 12.46528703574805874 ) ) ;
#909=CARTESIAN_POINT ( 'NONE',  ( -0.1745138560722763466, 100.7898137178985536, -12.50000000000000355 ) ) ;
#910=CARTESIAN_POINT ( 'NONE',  ( -10.69584247140444866, 103.8476862821014493, 6.932735513423972762 ) ) ;
#915=CARTESIAN_POINT ( 'NONE',  ( 15.53471296425188797, 84.97731371789856780, 2.908627838312457747 ) ) ;
#920=CARTESIAN_POINT ( 'NONE',  ( 9.465287035748067623, 100.3976862821014606, 2.064181346179272847 ) ) ;
#922=CARTESIAN_POINT ( 'NONE',  ( 1.715153634034445762, 55.07731371789854080, -9.534712964251895073 ) ) ;
#924=CARTESIAN_POINT ( 'NONE',  ( -6.594114490232462877, 115.7398137178985564, 6.840914352311949109 ) ) ;
#926=CARTESIAN_POINT ( 'NONE',  ( 0.1745138560722779009, 22.58981371789854720, 12.50000000000000355 ) ) ;
#928=CARTESIAN_POINT ( 'NONE',  ( 0.1745138560725515708, 79.41018628210144925, -12.50000000000000355 ) ) ;
#931=CARTESIAN_POINT ( 'NONE',  ( -5.770363421893818234, 88.03518628210144925, -14.38691631536207005 ) ) ;
#936=CARTESIAN_POINT ( 'NONE',  ( 1.715153634034233487, 120.5226862821014322, 9.534712964251941258 ) ) ;
#938=CARTESIAN_POINT ( 'NONE',  ( -0.1745138560725500443, 139.2101862821014606, 12.50000000000000355 ) ) ;
#949=CARTESIAN_POINT ( 'NONE',  ( 5.233372021372610483, 28.05231371789855643, -8.152565276336593669 ) ) ;
#954=CARTESIAN_POINT ( 'NONE',  ( 7.228626920338837358, 30.92731371789854578, 10.49813415416005036 ) ) ;
#956=CARTESIAN_POINT ( 'NONE',  ( 13.04141134922778988, 139.0273137178985507, -8.927990412390371944 ) ) ;
#963=CARTESIAN_POINT ( 'NONE',  ( -8.962234695871760692, 131.1601862821014777, 8.715434833791933400 ) ) ;
#973=CARTESIAN_POINT ( 'NONE',  ( -14.38691631536207183, 131.7351862821014663, 5.770363421893814682 ) ) ;
#976=CARTESIAN_POINT ( 'NONE',  ( -9.534712964251941258, 122.8226862821014294, 1.715153634034234154 ) ) ;
#978=CARTESIAN_POINT ( 'NONE',  ( 12.50000000000000355, 35.71018628210144641, 0.1745138560725507937 ) ) ;
#982=CARTESIAN_POINT ( 'NONE',  ( 14.38691631536207538, 117.9351862821014407, -5.770363421893813793 ) ) ;
#984=CARTESIAN_POINT ( 'NONE',  ( -8.152565276336710909, 11.84768628210144747, 5.233372021372435512 ) ) ;
#991=CARTESIAN_POINT ( 'NONE',  ( 1.715153634034445762, 73.47731371789855359, -9.534712964251895073 ) ) ;
#995=CARTESIAN_POINT ( 'NONE',  ( 11.61527771782809637, 76.06481371789855928, 4.622313124798827388 ) ) ;
#999=CARTESIAN_POINT ( 'NONE',  ( -2.660918448318004614, 54.50231371789855217, -12.46528703574811558 ) ) ;
#1005=CARTESIAN_POINT ( 'NONE',  ( 2.660918448318279950, 24.49768628210144783, -12.46528703574805697 ) ) ;
#1010=CARTESIAN_POINT ( 'NONE',  ( 10.69584247140429589, 85.55231371789857064, 6.932735513424201024 ) ) ;
#1016=CARTESIAN_POINT ( 'NONE',  ( -8.632099005475794229, 60.25231371789854506, 13.23911966647199812 ) ) ;
#1020=CARTESIAN_POINT ( 'NONE',  ( -8.962234695871760692, 85.16018628210144925, 8.715434833791933400 ) ) ;
#1021=CARTESIAN_POINT ( 'NONE',  ( -13.23911966647218463, 21.04768628210144499, 8.632099005475506459 ) ) ;
#1026=CARTESIAN_POINT ( 'NONE',  ( -8.927990412390661490, 57.27268628210143220, 13.04141134922759804 ) ) ;
#1033=CARTESIAN_POINT ( 'NONE',  ( -11.48171059495397373, 22.48518628210144499, -4.944772684328680334 ) ) ;
#1035=CARTESIAN_POINT ( 'NONE',  ( 8.710071997420211432, 130.1148137178985564, -3.796722387233181895 ) ) ;
#1040=CARTESIAN_POINT ( 'NONE',  ( 12.53471296425189330, 140.1773137178985849, 2.311890736173451533 ) ) ;
#1045=CARTESIAN_POINT ( 'NONE',  ( -7.228626920339070061, 48.07268628210144357, 10.49813415415989404 ) ) ;
#1052=CARTESIAN_POINT ( 'NONE',  ( -4.622313124798576922, 78.83518628210146062, -11.61527771782819762 ) ) ;
#1053=CARTESIAN_POINT ( 'NONE',  ( 13.04141134922778988, 19.42731371789854933, -8.927990412390371944 ) ) ;
#1059=CARTESIAN_POINT ( 'NONE',  ( -11.48171059495408208, 143.9148137178985678, 4.944772684328421875 ) ) ;
#1068=CARTESIAN_POINT ( 'NONE',  ( 14.25334919248795451, 120.9148137178985678, -6.092822981423661410 ) ) ;
#1073=CARTESIAN_POINT ( 'NONE',  ( -8.715434833791929847, 32.26018628210145067, -8.962234695871762469 ) ) ;
#1077=CARTESIAN_POINT ( 'NONE',  ( -3.257655550457281723, 111.8976862821014606, 15.46528703574804986 ) ) ;
#1080=CARTESIAN_POINT ( 'NONE',  ( 3.474262827703335166, 46.63518628210144357, 8.843639120294326972 ) ) ;
#1084=CARTESIAN_POINT ( 'NONE',  ( -7.228626920339069173, 84.87268628210146915, 10.49813415415989581 ) ) ;
#1087=CARTESIAN_POINT ( 'NONE',  ( 0.1745138560725194299, 51.81018628210144783, -9.500000000000005329 ) ) ;
#1097=CARTESIAN_POINT ( 'NONE',  ( -4.622313124798826500, 96.76481371789854791, 11.61527771782809637 ) ) ;
#1098=CARTESIAN_POINT ( 'NONE',  ( 11.48171059495397728, 100.6851862821014691, 4.944772684328674117 ) ) ;
#1104=CARTESIAN_POINT ( 'NONE',  ( -0.1745138560722442889, 73.18981371789854506, -15.50000000000000533 ) ) ;
#1107=CARTESIAN_POINT ( 'NONE',  ( 0.1745138560725194299, 97.81018628210145494, -9.500000000000005329 ) ) ;
#1110=CARTESIAN_POINT ( 'NONE',  ( 3.474262827703532341, 64.56481371789854506, -8.843639120294245259 ) ) ;
#1113=CARTESIAN_POINT ( 'NONE',  ( 9.534712964251900402, 121.7773137178985650, 1.715153634034445540 ) ) ;
#1115=CARTESIAN_POINT ( 'NONE',  ( -4.944772684328424539, 35.81481371789854506, -11.48171059495408031 ) ) ;
#1117=CARTESIAN_POINT ( 'NONE',  ( 11.61527771782819940, 90.33518628210144641, -4.622313124798573369 ) ) ;
#1122=CARTESIAN_POINT ( 'NONE',  ( 4.944772684328679446, 6.385186282101440014, -11.48171059495397373 ) ) ;
#1125=CARTESIAN_POINT ( 'NONE',  ( -8.710071997420127943, 105.2851862821014777, -3.796722387233380402 ) ) ;
#1127=CARTESIAN_POINT ( 'NONE',  ( 4.622313124798573369, 129.4351862821014549, 11.61527771782819940 ) ) ;
#1137=CARTESIAN_POINT ( 'NONE',  ( 6.840914352311949109, 21.43981371789854506, 6.594114490232462877 ) ) ;
#1142=CARTESIAN_POINT ( 'NONE',  ( 6.932735513424201024, 18.85231371789855714, -10.69584247140429412 ) ) ;
#1144=CARTESIAN_POINT ( 'NONE',  ( 14.25334919248795451, 130.1148137178985564, -6.092822981423661410 ) ) ;
#1152=CARTESIAN_POINT ( 'NONE',  ( -7.228626920339069173, 140.0726862821014720, 10.49813415415989581 ) ) ;
#1157=SURFACE_STYLE_USAGE ( .BOTH. , #35084 ) ;
#1160=CARTESIAN_POINT ( 'NONE',  ( -11.48171059495397373, 132.8851862821014720, -4.944772684328680334 ) ) ;
#1164=CARTESIAN_POINT ( 'NONE',  ( 3.257655550457285720, 134.8976862821014606, -15.46528703574804986 ) ) ;
#1166=CARTESIAN_POINT ( 'NONE',  ( 5.529263428287477744, 135.4726862821014777, -7.954856959092191815 ) ) ;
#1168=CARTESIAN_POINT ( 'NONE',  ( -12.50000000000000355, 31.11018628210143788, -0.1745138560725492671 ) ) ;
#1172=CARTESIAN_POINT ( 'NONE',  ( -2.908627838312119351, 115.9226862821014521, -15.53471296425195369 ) ) ;
#1173=CARTESIAN_POINT ( 'NONE',  ( 5.529263428287300108, 141.3273137178985621, 7.954856959092309943 ) ) ;
#1180=CARTESIAN_POINT ( 'NONE',  ( 6.840914352311949109, 76.63981371789854791, 6.594114490232462877 ) ) ;
#1183=CARTESIAN_POINT ( 'NONE',  ( 4.622313124798831829, 73.76481371789856212, -11.61527771782809282 ) ) ;
#1187=CARTESIAN_POINT ( 'NONE',  ( -6.932735513424201912, 41.85231371789855359, 10.69584247140429412 ) ) ;
#1191=CARTESIAN_POINT ( 'NONE',  ( -0.1745138560725500443, 28.81018628210144072, 12.50000000000000355 ) ) ;
#1197=CARTESIAN_POINT ( 'NONE',  ( -10.69584247140429412, 80.95231371789856212, -6.932735513424201024 ) ) ;
#1202=CARTESIAN_POINT ( 'NONE',  ( 0.1745138560722461762, 50.18981371789855217, 15.50000000000000533 ) ) ;
#1206=CARTESIAN_POINT ( 'NONE',  ( 8.715434833791931624, 82.86018628210145209, 8.962234695871760692 ) ) ;
#1207=CARTESIAN_POINT ( 'NONE',  ( -14.25334919248782306, 22.48518628210144499, -6.092822981423979378 ) ) ;
#1210=VERTEX_POINT ( 'NONE', #23595 ) ;
#1211=CARTESIAN_POINT ( 'NONE',  ( -5.770363421893818234, 42.03518628210144925, -14.38691631536207005 ) ) ;
#1217=CARTESIAN_POINT ( 'NONE',  ( -7.228626920339069173, 29.67268628210144499, 10.49813415415989581 ) ) ;
#1219=CARTESIAN_POINT ( 'NONE',  ( -3.796722387233185003, 137.0148137178985621, -8.710071997420207879 ) ) ;
#1224=CARTESIAN_POINT ( 'NONE',  ( -2.311890736173447980, 133.2773137178985507, 12.53471296425189330 ) ) ;
#1230=CARTESIAN_POINT ( 'NONE',  ( 10.69584247140445221, 44.04768628210144499, -6.932735513423970097 ) ) ;
#1239=CARTESIAN_POINT ( 'NONE',  ( 0.1745138560725515708, 70.21018628210144641, -12.50000000000000355 ) ) ;
#1240=CARTESIAN_POINT ( 'NONE',  ( 0.1745138560722461762, 13.38981371789854613, 15.50000000000000533 ) ) ;
#1247=CARTESIAN_POINT ( 'NONE',  ( -11.48171059495408208, 134.7148137178985507, 4.944772684328421875 ) ) ;
#1254=CARTESIAN_POINT ( 'NONE',  ( -14.25334919248795096, 107.1148137178985564, 6.092822981423662299 ) ) ;
#1257=CARTESIAN_POINT ( 'NONE',  ( 8.715434833791931624, 18.46018628210144286, 8.962234695871760692 ) ) ;
#1261=CARTESIAN_POINT ( 'NONE',  ( -0.1745138560725817967, 111.6101862821014521, 15.50000000000000533 ) ) ;
#1264=CARTESIAN_POINT ( 'NONE',  ( -7.954856959092191815, 41.17268628210143078, -5.529263428287477744 ) ) ;
#1268=CARTESIAN_POINT ( 'NONE',  ( 11.61527771782819940, 71.93518628210145494, -4.622313124798573369 ) ) ;
#1271=CARTESIAN_POINT ( 'NONE',  ( -8.843639120294326972, 48.93518628210144072, 3.474262827703335166 ) ) ;
#1281=CARTESIAN_POINT ( 'NONE',  ( 2.311890736173452865, 110.2773137178985650, -12.53471296425189152 ) ) ;
#1282=CARTESIAN_POINT ( 'NONE',  ( -12.53471296425194659, 104.4226862821014521, 2.311890736173176641 ) ) ;
#1289=CARTESIAN_POINT ( 'NONE',  ( 13.23911966647199812, 67.15231371789852233, 8.632099005475788900 ) ) ;
#1292=CARTESIAN_POINT ( 'NONE',  ( -0.1745138560725182642, 93.21018628210146062, 9.500000000000005329 ) ) ;
#1295=CARTESIAN_POINT ( 'NONE',  ( -5.233372021372612259, 51.05231371789854222, 8.152565276336593669 ) ) ;
#1298=CARTESIAN_POINT ( 'NONE',  ( -6.840914352311947333, 108.8398137178985507, -6.594114490232462877 ) ) ;
#1300=CARTESIAN_POINT ( 'NONE',  ( -0.1745138560722763466, 36.38981371789855501, -12.50000000000000355 ) ) ;
#1302=CARTESIAN_POINT ( 'NONE',  ( -8.715434833791929847, 87.46018628210144641, -8.962234695871762469 ) ) ;
#1310=CARTESIAN_POINT ( 'NONE',  ( -12.50000000000000355, 6.489813717898557321, 0.1745138560722786503 ) ) ;
#1312=CARTESIAN_POINT ( 'NONE',  ( -3.796722387233375073, 102.9851862821014805, 8.710071997420127943 ) ) ;
#1315=CARTESIAN_POINT ( 'NONE',  ( 12.53471296425194836, 136.6226862821014834, -2.311890736173178418 ) ) ;
#1316=CARTESIAN_POINT ( 'NONE',  ( -6.422845572874366304, 142.9999999999996305, 10.72508787064079172 ) ) ;
#1328=CARTESIAN_POINT ( 'NONE',  ( 8.152565276336593669, 21.15231371789855430, 5.233372021372610483 ) ) ;
#1334=CARTESIAN_POINT ( 'NONE',  ( -11.61527771782809282, 25.46481371789855075, -4.622313124798832717 ) ) ;
#1336=CARTESIAN_POINT ( 'NONE',  ( -14.38691631536193860, 126.6648137178985820, -5.770363421894132649 ) ) ;
#1342=CARTESIAN_POINT ( 'NONE',  ( -4.622313124798576922, 134.0351862821014493, -11.61527771782819762 ) ) ;
#1349=CARTESIAN_POINT ( 'NONE',  ( 11.48171059495397728, 137.4851862821014663, 4.944772684328674117 ) ) ;
#1353=CARTESIAN_POINT ( 'NONE',  ( 8.632099005475504683, 129.1476862821014322, 13.23911966647218996 ) ) ;
#1356=CARTESIAN_POINT ( 'NONE',  ( 9.465287035748067623, 118.7976862821014521, 2.064181346179272847 ) ) ;
#1360=CARTESIAN_POINT ( 'NONE',  ( -10.49813415415989581, 13.57268628210145600, -7.228626920339068285 ) ) ;
#1364=CARTESIAN_POINT ( 'NONE',  ( 13.23911966647218996, 117.6476862821014322, -8.632099005475504683 ) ) ;
#1366=CARTESIAN_POINT ( 'NONE',  ( 9.500000000000005329, 8.110186282101443211, 0.1745138560725188748 ) ) ;
#1373=CARTESIAN_POINT ( 'NONE',  ( -5.529263428287297444, 81.52731371789856496, -7.954856959092311719 ) ) ;
#1377=CARTESIAN_POINT ( 'NONE',  ( 4.944772684328420986, 77.21481371789855075, 11.48171059495408208 ) ) ;
#1380=CARTESIAN_POINT ( 'NONE',  ( -12.50000000000000355, 52.48981371789855643, 0.1745138560722786503 ) ) ;
#1384=CARTESIAN_POINT ( 'NONE',  ( -11.61527771782819940, 21.33518628210144641, 4.622313124798574258 ) ) ;
#1389=CARTESIAN_POINT ( 'NONE',  ( 0.1745138560722779009, 77.78981371789855359, 12.50000000000000355 ) ) ;
#1394=CARTESIAN_POINT ( 'NONE',  ( 0.1745138560722461762, 59.38981371789856212, 15.50000000000000533 ) ) ;
#1397=CARTESIAN_POINT ( 'NONE',  ( -12.46528703574805697, 77.39768628210144641, -2.660918448318280838 ) ) ;
#1398=CARTESIAN_POINT ( 'NONE',  ( 13.23911966647218996, 34.84768628210143504, -8.632099005475504683 ) ) ;
#1402=CARTESIAN_POINT ( 'NONE',  ( -13.23911966647218463, 39.44768628210144357, 8.632099005475506459 ) ) ;
#1408=CARTESIAN_POINT ( 'NONE',  ( 12.53471296425194836, 26.22268628210144925, -2.311890736173178418 ) ) ;
#1410=CARTESIAN_POINT ( 'NONE',  ( 7.954856959092311719, 129.8273137178985905, -5.529263428287300108 ) ) ;
#1414=CARTESIAN_POINT ( 'NONE',  ( 4.944772684328420986, 141.6148137178985849, 11.48171059495408208 ) ) ;
#1420=CARTESIAN_POINT ( 'NONE',  ( -8.962234695871760692, 29.96018628210143930, 8.715434833791933400 ) ) ;
#1426=( GEOMETRIC_REPRESENTATION_CONTEXT ( 3 ) GLOBAL_UNCERTAINTY_ASSIGNED_CONTEXT ( ( #4017 ) ) GLOBAL_UNIT_ASSIGNED_CONTEXT ( ( #8757, #31502, #25813 ) ) REPRESENTATION_CONTEXT ( 'NONE', 'WORKASPACE' ) );
#1429=CARTESIAN_POINT ( 'NONE',  ( -12.53471296425194836, 86.02268628210146062, 2.311890736173176641 ) ) ;
#1430=CARTESIAN_POINT ( 'NONE',  ( -13.04141134922759804, 133.1726862821014663, -8.927990412390657937 ) ) ;
#1437=CARTESIAN_POINT ( 'NONE',  ( -8.962234695871565293, 136.4398137178985735, -8.715434833792128799 ) ) ;
#1443=CARTESIAN_POINT ( 'NONE',  ( 6.092822981423662299, 104.8148137178985593, 14.25334919248795096 ) ) ;
#1447=FACE_OUTER_BOUND ( 'NONE', #12667, .T. ) ;
#1451=CARTESIAN_POINT ( 'NONE',  ( -5.770363421893818234, 97.23518628210146630, -14.38691631536207005 ) ) ;
#1456=CARTESIAN_POINT ( 'NONE',  ( 2.064181346179272847, 42.89768628210143220, -9.465287035748065847 ) ) ;
#1461=CARTESIAN_POINT ( 'NONE',  ( 2.660918448318279950, 70.49768628210145494, -12.46528703574805697 ) ) ;
#1463=CARTESIAN_POINT ( 'NONE',  ( -7.954856959092191815, 41.17268628210143078, -5.529263428287477744 ) ) ;
#1473=CARTESIAN_POINT ( 'NONE',  ( 0.1745138560722779009, 77.78981371789855359, 12.50000000000000355 ) ) ;
#1474=CARTESIAN_POINT ( 'NONE',  ( 12.53471296425194659, 99.82268628210144357, -2.311890736173178418 ) ) ;
#1479=CARTESIAN_POINT ( 'NONE',  ( -15.53471296425188442, 61.97731371789853938, -2.908627838312459080 ) ) ;
#1485=CARTESIAN_POINT ( 'NONE',  ( -7.954856959092309943, 60.82731371789854080, 5.529263428287300108 ) ) ;
#1488=CARTESIAN_POINT ( 'NONE',  ( -7.954856959092309943, 106.8273137178985479, 5.529263428287300108 ) ) ;
#1489=CARTESIAN_POINT ( 'NONE',  ( 8.715434833792128799, 37.53981371789855359, -8.962234695871567070 ) ) ;
#1490=CARTESIAN_POINT ( 'NONE',  ( 10.69584247140445221, 90.04768628210145209, -6.932735513423970097 ) ) ;
#1498=CARTESIAN_POINT ( 'NONE',  ( 6.840914352312096547, 98.96018628210144641, -6.594114490232313663 ) ) ;
#1500=CARTESIAN_POINT ( 'NONE',  ( -2.660918448318275509, 139.4976862821014549, 12.46528703574805874 ) ) ;
#1512=CARTESIAN_POINT ( 'NONE',  ( 5.233372021372610483, 9.652313717898541867, -8.152565276336593669 ) ) ;
#1517=CARTESIAN_POINT ( 'NONE',  ( -2.660918448318005058, 26.90231371789854364, -12.46528703574811558 ) ) ;
#1519=CARTESIAN_POINT ( 'NONE',  ( 11.08355503943118769, 122.6398137178985479, 10.83675517735179028 ) ) ;
#1526=CARTESIAN_POINT ( 'NONE',  ( -12.53471296425194836, 132.0226862821014606, 2.311890736173176641 ) ) ;
#1535=CARTESIAN_POINT ( 'NONE',  ( -12.53471296425194836, 141.2226862821014493, 2.311890736173176641 ) ) ;
#1541=CARTESIAN_POINT ( 'NONE',  ( -2.908627838312119351, 115.9226862821014521, -15.53471296425195369 ) ) ;
#1543=CARTESIAN_POINT ( 'NONE',  ( -5.529263428287477744, 112.4726862821014635, 7.954856959092191815 ) ) ;
#1545=CARTESIAN_POINT ( 'NONE',  ( -7.228626920339069173, 20.47268628210144570, 10.49813415415989581 ) ) ;
#1549=CARTESIAN_POINT ( 'NONE',  ( -6.594114490232312775, 78.26018628210144357, -6.840914352312096547 ) ) ;
#1551=CARTESIAN_POINT ( 'NONE',  ( -5.529263428287297444, 127.5273137178985792, -7.954856959092311719 ) ) ;
#1557=CARTESIAN_POINT ( 'NONE',  ( -6.840914352311947333, 62.83981371789855785, -6.594114490232462877 ) ) ;
#1560=CARTESIAN_POINT ( 'NONE',  ( 12.46528703574811558, 84.40231371789853654, -2.660918448318005947 ) ) ;
#1564=CARTESIAN_POINT ( 'NONE',  ( -4.622313124798826500, 50.76481371789855501, 11.61527771782809637 ) ) ;
#1570=CARTESIAN_POINT ( 'NONE',  ( -8.715434833791929847, 23.06018628210145138, -8.962234695871762469 ) ) ;
#1575=CARTESIAN_POINT ( 'NONE',  ( 10.69584247140429589, 67.15231371789855075, 6.932735513424201024 ) ) ;
#1582=CARTESIAN_POINT ( 'NONE',  ( 3.257655550456945548, 31.50231371789854862, 15.46528703574811736 ) ) ;
#1585=CARTESIAN_POINT ( 'NONE',  ( -11.61527771782819940, 67.33518628210144641, 4.622313124798574258 ) ) ;
#1586=CARTESIAN_POINT ( 'NONE',  ( 13.23911966647218996, 25.64768628210144286, -8.632099005475504683 ) ) ;
#1592=CARTESIAN_POINT ( 'NONE',  ( -10.83675517735155047, 32.26018628210145067, -11.08355503943142750 ) ) ;
#1600=CARTESIAN_POINT ( 'NONE',  ( -9.500000000000005329, 126.0898137178985650, 0.1745138560723101806 ) ) ;
#1605=CARTESIAN_POINT ( 'NONE',  ( -4.944772684328424539, 137.0148137178985621, -11.48171059495408031 ) ) ;
#1611=CARTESIAN_POINT ( 'NONE',  ( 2.311890736173175753, 37.72268628210144215, 12.53471296425194659 ) ) ;
#1619=CARTESIAN_POINT ( 'NONE',  ( -4.944772684328673229, 75.38518628210144357, 11.48171059495397728 ) ) ;
#1620=CARTESIAN_POINT ( 'NONE',  ( -14.38691631536193860, 7.064813717898548617, -5.770363421894132649 ) ) ;
#1627=CARTESIAN_POINT ( 'NONE',  ( 12.53471296425189330, 121.7773137178985792, 2.311890736173451977 ) ) ;
#1634=CARTESIAN_POINT ( 'NONE',  ( 0.1745138560722461762, 105.3898137178985479, 15.50000000000000533 ) ) ;
#1639=CARTESIAN_POINT ( 'NONE',  ( -12.46528703574805697, 123.3976862821014606, -2.660918448318280838 ) ) ;
#1640=CARTESIAN_POINT ( 'NONE',  ( 8.927990412390657937, 80.27268628210143220, -13.04141134922759804 ) ) ;
#1643=CARTESIAN_POINT ( 'NONE',  ( -3.257655550457281723, 84.29768628210146630, 15.46528703574804986 ) ) ;
#1646=CARTESIAN_POINT ( 'NONE',  ( 9.500000000000005329, 44.91018628210144215, 0.1745138560725188748 ) ) ;
#1650=CARTESIAN_POINT ( 'NONE',  ( -12.53471296425194836, 67.62268628210145494, 2.311890736173176641 ) ) ;
#1653=CARTESIAN_POINT ( 'NONE',  ( -9.465287035748065847, 49.79768628210144499, -2.064181346179273735 ) ) ;
#1662=CARTESIAN_POINT ( 'NONE',  ( -12.53471296425189152, 89.57731371789856212, -2.311890736173453753 ) ) ;
#1663=CARTESIAN_POINT ( 'NONE',  ( -11.48171059495397373, 77.68518628210145494, -4.944772684328680334 ) ) ;
#1669=CARTESIAN_POINT ( 'NONE',  ( 13.23911966647199812, 57.95231371789854791, 8.632099005475788900 ) ) ;
#1674=CARTESIAN_POINT ( 'NONE',  ( -3.474262827703527901, 59.96481371789855075, 8.843639120294245259 ) ) ;
#1676=CARTESIAN_POINT ( 'NONE',  ( -6.594114490232462877, 88.13981371789856212, 6.840914352311949109 ) ) ;
#1678=CARTESIAN_POINT ( 'NONE',  ( -7.228626920338836470, 26.32731371789854791, -10.49813415416005213 ) ) ;
#1679=CARTESIAN_POINT ( 'NONE',  ( -7.228626920339069173, 84.87268628210146915, 10.49813415415989581 ) ) ;
#1685=CARTESIAN_POINT ( 'NONE',  ( 9.534712964251941258, 90.62268628210145494, -1.715153634034235708 ) ) ;
#1687=CARTESIAN_POINT ( 'NONE',  ( 4.944772684328679446, 125.9851862821014521, -11.48171059495397373 ) ) ;
#1700=CARTESIAN_POINT ( 'NONE',  ( 4.944772684328420986, 132.4148137178985678, 11.48171059495408208 ) ) ;
#1705=CARTESIAN_POINT ( 'NONE',  ( -12.50000000000000355, 15.68981371789854329, 0.1745138560722786503 ) ) ;
#1707=CARTESIAN_POINT ( 'NONE',  ( 15.46528703574811736, 112.0023137178985451, -3.257655550456947768 ) ) ;
#1715=CARTESIAN_POINT ( 'NONE',  ( -8.715434833791929847, 124.2601862821014578, -8.962234695871762469 ) ) ;
#1724=CARTESIAN_POINT ( 'NONE',  ( -10.49813415415989581, 133.1726862821014663, -7.228626920339068285 ) ) ;
#1730=CARTESIAN_POINT ( 'NONE',  ( -3.257655550457281723, 121.0976862821014635, 15.46528703574804986 ) ) ;
#1732=CARTESIAN_POINT ( 'NONE',  ( -2.660918448318275509, 19.89768628210143575, 12.46528703574805874 ) ) ;
#1737=CARTESIAN_POINT ( 'NONE',  ( -8.710071997420127943, 86.88518628210145778, -3.796722387233380402 ) ) ;
#1739=CARTESIAN_POINT ( 'NONE',  ( 5.529263428287300108, 122.9273137178985422, 7.954856959092309943 ) ) ;
#1746=CARTESIAN_POINT ( 'NONE',  ( 9.500000000000005329, 57.08981371789855075, -0.1745138560723090149 ) ) ;
#1750=CARTESIAN_POINT ( 'NONE',  ( 11.48171059495408208, 74.91481371789855359, -4.944772684328420986 ) ) ;
#1755=CARTESIAN_POINT ( 'NONE',  ( 2.311890736173452865, 27.47731371789855004, -12.53471296425189152 ) ) ;
#1758=CARTESIAN_POINT ( 'NONE',  ( 7.228626920339068285, 25.07268628210144712, -10.49813415415989581 ) ) ;
#1765=CARTESIAN_POINT ( 'NONE',  ( 12.46528703574811558, 75.20231371789856212, -2.660918448318005503 ) ) ;
#1770=CARTESIAN_POINT ( 'NONE',  ( 13.23911966647199812, 48.75231371789854506, 8.632099005475788900 ) ) ;
#1773=CARTESIAN_POINT ( 'NONE',  ( 10.69584247140445221, 62.44768628210145778, -6.932735513423970097 ) ) ;
#1774=CARTESIAN_POINT ( 'NONE',  ( 15.50000000000000533, 8.110186282101443211, 0.1745138560725827404 ) ) ;
#1779=CARTESIAN_POINT ( 'NONE',  ( 0.1745138560725837118, 33.41018628210144925, -15.50000000000000533 ) ) ;
#1784=CARTESIAN_POINT ( 'NONE',  ( -2.311890736173176641, 5.522686282101451738, -12.53471296425194836 ) ) ;
#1786=CARTESIAN_POINT ( 'NONE',  ( -6.840914352311947333, 118.0398137178985536, -6.594114490232462877 ) ) ;
#1792=CARTESIAN_POINT ( 'NONE',  ( -6.422845572874366304, 142.9999999999996305, 10.72508787064079172 ) ) ;
#1798=CARTESIAN_POINT ( 'NONE',  ( 10.69584247140445221, 34.84768628210144215, -6.932735513423970097 ) ) ;
#1806=CARTESIAN_POINT ( 'NONE',  ( -8.715434833791929847, 78.26018628210144357, -8.962234695871762469 ) ) ;
#1807=CARTESIAN_POINT ( 'NONE',  ( 10.83675517735155225, 138.0601862821014549, 11.08355503943142573 ) ) ;
#1813=CARTESIAN_POINT ( 'NONE',  ( 12.46528703574811558, 121.2023137178985621, -2.660918448318005503 ) ) ;
#1818=CARTESIAN_POINT ( 'NONE',  ( -14.25334919248795096, 97.91481371789856780, 6.092822981423662299 ) ) ;
#1822=CARTESIAN_POINT ( 'NONE',  ( -8.715434833791929847, 124.2601862821014578, -8.962234695871762469 ) ) ;
#1823=CARTESIAN_POINT ( 'NONE',  ( 13.23911966647218996, 62.44768628210144357, -8.632099005475504683 ) ) ;
#1827=CARTESIAN_POINT ( 'NONE',  ( -15.46528703574804986, 86.59768628210143504, -3.257655550457287497 ) ) ;
#1830=CARTESIAN_POINT ( 'NONE',  ( 6.594114490232313663, 46.06018628210144072, 6.840914352312096547 ) ) ;
#1835=CARTESIAN_POINT ( 'NONE',  ( -12.53471296425194836, 49.22268628210144215, 2.311890736173176641 ) ) ;
#1838=CARTESIAN_POINT ( 'NONE',  ( -7.954856959092191815, 31.97268628210143149, -5.529263428287477744 ) ) ;
#1848=CARTESIAN_POINT ( 'NONE',  ( -10.69584247140429412, 90.15231371789856496, -6.932735513424201024 ) ) ;
#1849=CARTESIAN_POINT ( 'NONE',  ( 8.715434833791931624, 92.06018628210145494, 8.962234695871760692 ) ) ;
#1854=CARTESIAN_POINT ( 'NONE',  ( 11.08355503943118769, 58.23981371789854222, 10.83675517735179028 ) ) ;
#1859=CARTESIAN_POINT ( 'NONE',  ( 8.710071997420211432, 38.11481371789853512, -3.796722387233181895 ) ) ;
#1861=CARTESIAN_POINT ( 'NONE',  ( -2.064181346179062349, 100.5023137178985451, -9.465287035748106703 ) ) ;
#1863=CARTESIAN_POINT ( 'NONE',  ( 6.932735513424201024, 9.652313717898541867, -10.69584247140429412 ) ) ;
#1864=CARTESIAN_POINT ( 'NONE',  ( -6.932735513423968321, 60.14768628210144641, -10.69584247140445221 ) ) ;
#1873=CARTESIAN_POINT ( 'NONE',  ( 3.474262827703335166, 92.63518628210147199, 8.843639120294326972 ) ) ;
#1875=CARTESIAN_POINT ( 'NONE',  ( -2.660918448318275509, 121.0976862821014635, 12.46528703574805874 ) ) ;
#1888=CARTESIAN_POINT ( 'NONE',  ( -4.622313124798826500, 142.7648137178985621, 11.61527771782809637 ) ) ;
#1889=CARTESIAN_POINT ( 'NONE',  ( 8.715434833791931624, 138.0601862821014549, 8.962234695871760692 ) ) ;
#1895=CARTESIAN_POINT ( 'NONE',  ( 15.46528703574811736, 121.2023137178985479, -3.257655550456947768 ) ) ;
#1902=CARTESIAN_POINT ( 'NONE',  ( 12.50000000000000355, 118.5101862821014578, 0.1745138560725507937 ) ) ;
#1908=CARTESIAN_POINT ( 'NONE',  ( 2.660918448318279950, 134.8976862821014890, -12.46528703574805697 ) ) ;
#1913=CARTESIAN_POINT ( 'NONE',  ( 10.83675517735155225, 119.6601862821014635, 11.08355503943142573 ) ) ;
#1916=CARTESIAN_POINT ( 'NONE',  ( -8.715434833791929847, 4.660186282101435928, -8.962234695871762469 ) ) ;
#1920=CARTESIAN_POINT ( 'NONE',  ( 1.715153634034233487, 74.52268628210144641, 9.534712964251941258 ) ) ;
#1922=CARTESIAN_POINT ( 'NONE',  ( -5.233372021372612259, 124.6523137178985650, 8.152565276336593669 ) ) ;
#1928=CARTESIAN_POINT ( 'NONE',  ( -6.594114490232462877, 60.53981371789856070, 6.840914352311949109 ) ) ;
#1933=CARTESIAN_POINT ( 'NONE',  ( -8.715434833792127023, 60.53981371789856070, 8.962234695871568846 ) ) ;
#1937=CARTESIAN_POINT ( 'NONE',  ( -0.1745138560722763466, 36.38981371789855501, -12.50000000000000355 ) ) ;
#1940=CARTESIAN_POINT ( 'NONE',  ( -11.48171059495397373, 4.085186282101443744, -4.944772684328680334 ) ) ;
#1945=CARTESIAN_POINT ( 'NONE',  ( -11.61527771782809282, 62.26481371789854791, -4.622313124798832717 ) ) ;
#1951=CARTESIAN_POINT ( 'NONE',  ( 15.46528703574811736, 47.60231371789853938, -3.257655550456947768 ) ) ;
#1953=CARTESIAN_POINT ( 'NONE',  ( 8.962234695871762469, 25.36018628210144499, -8.715434833791931624 ) ) ;
#1956=CARTESIAN_POINT ( 'NONE',  ( -10.49813415415989581, 59.57268628210145778, -7.228626920339068285 ) ) ;
#1957=CARTESIAN_POINT ( 'NONE',  ( 15.46528703574804986, 17.59768628210143504, 3.257655550457285720 ) ) ;
#1961=CARTESIAN_POINT ( 'NONE',  ( -8.927990412390661490, 29.67268628210143788, 13.04141134922759804 ) ) ;
#1969=CARTESIAN_POINT ( 'NONE',  ( 9.500000000000005329, 103.0898137178985792, -0.1745138560723090149 ) ) ;
#1975=CARTESIAN_POINT ( 'NONE',  ( -2.311890736173447980, 114.8773137178985735, 12.53471296425189330 ) ) ;
#1982=CARTESIAN_POINT ( 'NONE',  ( 12.46528703574805874, 26.79768628210144144, 2.660918448318279950 ) ) ;
#1990=CARTESIAN_POINT ( 'NONE',  ( 11.48171059495397728, 63.88518628210145067, 4.944772684328674117 ) ) ;
#1991=CARTESIAN_POINT ( 'NONE',  ( 6.092822981423978490, 135.1851862821014549, -14.25334919248782306 ) ) ;
#1997=CARTESIAN_POINT ( 'NONE',  ( 2.311890736173452865, 128.6773137178985564, -12.53471296425189152 ) ) ;
#2003=CARTESIAN_POINT ( 'NONE',  ( -13.04141134922778456, 88.42731371789855643, 8.927990412390377273 ) ) ;
#2007=CARTESIAN_POINT ( 'NONE',  ( 2.660918448318279950, 116.4976862821014549, -12.46528703574805697 ) ) ;
#2008=CARTESIAN_POINT ( 'NONE',  ( 10.83675517735155225, 73.66018628210144925, 11.08355503943142573 ) ) ;
#2011=CARTESIAN_POINT ( 'NONE',  ( -15.50000000000000533, 86.31018628210145494, -0.1745138560725808530 ) ) ;
#2015=CARTESIAN_POINT ( 'NONE',  ( 3.796722387233379514, 24.78518628210144215, -8.710071997420127943 ) ) ;
#2018=CARTESIAN_POINT ( 'NONE',  ( 11.48171059495397728, 63.88518628210145067, 4.944772684328674117 ) ) ;
#2021=CARTESIAN_POINT ( 'NONE',  ( 0.1745138560725194299, 24.21018628210144996, -9.500000000000005329 ) ) ;
#2033=CARTESIAN_POINT ( 'NONE',  ( -2.660918448318004614, 82.10231371789855359, -12.46528703574811558 ) ) ;
#2034=CARTESIAN_POINT ( 'NONE',  ( 6.932735513423970097, 83.14768628210144641, 10.69584247140445044 ) ) ;
#2039=CARTESIAN_POINT ( 'NONE',  ( 14.38691631536194393, 57.66481371789855359, 5.770363421894124656 ) ) ;
#2045=CARTESIAN_POINT ( 'NONE',  ( 6.840914352311949109, 39.83981371789855075, 6.594114490232462877 ) ) ;
#2047=CARTESIAN_POINT ( 'NONE',  ( 8.843639120294245259, 94.46481371789855075, 3.474262827703527901 ) ) ;
#2049=CARTESIAN_POINT ( 'NONE',  ( -10.49813415416004858, 14.82731371789855501, 7.228626920338839135 ) ) ;
#2052=CARTESIAN_POINT ( 'NONE',  ( -12.53471296425194836, 58.42268628210145209, 2.311890736173176641 ) ) ;
#2061=CARTESIAN_POINT ( 'NONE',  ( -9.465287035748065847, 86.59768628210143504, -2.064181346179273735 ) ) ;
#2064=CARTESIAN_POINT ( 'NONE',  ( -11.48171059495397373, 114.4851862821014521, -4.944772684328680334 ) ) ;
#2077=CARTESIAN_POINT ( 'NONE',  ( -0.1745138560723084320, 8.789813717898553591, -9.500000000000005329 ) ) ;
#2086=CARTESIAN_POINT ( 'NONE',  ( 15.53471296425188797, 121.7773137178985650, 2.908627838312457747 ) ) ;
#2092=CARTESIAN_POINT ( 'NONE',  ( 7.228626920339068285, 107.8726862821014549, -10.49813415415989581 ) ) ;
#2098=CARTESIAN_POINT ( 'NONE',  ( -7.228626920339069173, 121.6726862821014521, 10.49813415415989581 ) ) ;
#2103=CARTESIAN_POINT ( 'NONE',  ( -8.632099005475501130, 115.3476862821014493, -13.23911966647218996 ) ) ;
#2105=CARTESIAN_POINT ( 'NONE',  ( 10.49813415415989581, 8.972686282101431487, 7.228626920339068285 ) ) ;
#2109=CARTESIAN_POINT ( 'NONE',  ( -8.843639120294326972, 85.73518628210145209, 3.474262827703335166 ) ) ;
#2116=CARTESIAN_POINT ( 'NONE',  ( -8.710071997420207879, 51.91481371789856070, 3.796722387233182339 ) ) ;
#2120=CARTESIAN_POINT ( 'NONE',  ( 11.48171059495408208, 56.51481371789855501, -4.944772684328420986 ) ) ;
#2124=CARTESIAN_POINT ( 'NONE',  ( -2.660918448318004614, 36.10231371789853938, -12.46528703574811558 ) ) ;
#2134=CARTESIAN_POINT ( 'NONE',  ( 12.53471296425189330, 75.77731371789855075, 2.311890736173451977 ) ) ;
#2139=CARTESIAN_POINT ( 'NONE',  ( -8.927990412390371944, 35.52731371789855075, -13.04141134922778988 ) ) ;
#2141=CARTESIAN_POINT ( 'NONE',  ( -7.228626920339069173, 20.47268628210144570, 10.49813415415989581 ) ) ;
#2142=CARTESIAN_POINT ( 'NONE',  ( 7.228626920339068285, 61.87268628210145494, -10.49813415415989581 ) ) ;
#2143=CARTESIAN_POINT ( 'NONE',  ( -10.83675517735155047, 4.660186282101435928, -11.08355503943142750 ) ) ;
#2147=CARTESIAN_POINT ( 'NONE',  ( -6.092822981423970496, 38.58518628210143930, 14.25334919248782661 ) ) ;
#2155=CARTESIAN_POINT ( 'NONE',  ( -8.152565276336593669, 117.7523137178985735, -5.233372021372610483 ) ) ;
#2160=CARTESIAN_POINT ( 'NONE',  ( -4.622313124798826500, 115.1648137178985678, 11.61527771782809637 ) ) ;
#2174=CARTESIAN_POINT ( 'NONE',  ( 12.46528703574805874, 63.59768628210145636, 2.660918448318279950 ) ) ;
#2180=CARTESIAN_POINT ( 'NONE',  ( 11.48171059495408208, 130.1148137178985564, -4.944772684328420986 ) ) ;
#2186=CARTESIAN_POINT ( 'NONE',  ( 3.257655550456945548, 86.70231371789851949, 15.46528703574811736 ) ) ;
#2191=CARTESIAN_POINT ( 'NONE',  ( -8.962234695871760692, 131.1601862821014777, 8.715434833791933400 ) ) ;
#2192=CARTESIAN_POINT ( 'NONE',  ( -15.50000000000000533, 58.71018628210145351, -0.1745138560725808530 ) ) ;
#2195=CARTESIAN_POINT ( 'NONE',  ( -6.092822981423970496, 84.58518628210146062, 14.25334919248782661 ) ) ;
#2199=CARTESIAN_POINT ( 'NONE',  ( 9.465287035748067623, 17.59768628210143504, 2.064181346179272847 ) ) ;
#2203=CARTESIAN_POINT ( 'NONE',  ( 2.660918448318279950, 61.29768628210143788, -12.46528703574805697 ) ) ;
#2206=CARTESIAN_POINT ( 'NONE',  ( 8.843639120294328748, 25.93518628210144072, -3.474262827703334722 ) ) ;
#2217=CARTESIAN_POINT ( 'NONE',  ( -10.49813415415989404, 87.17268628210145209, -7.228626920339069173 ) ) ;
#2223=CARTESIAN_POINT ( 'NONE',  ( 13.23911966647199812, 48.75231371789854506, 8.632099005475788900 ) ) ;
#2230=CARTESIAN_POINT ( 'NONE',  ( -5.233372021372612259, 32.65231371789855075, 8.152565276336593669 ) ) ;
#2231=ADVANCED_FACE ( 'NONE', ( #15730 ), #27280, .F. ) ;
#2233=CARTESIAN_POINT ( 'NONE',  ( -0.1745138560723084320, 91.58981371789856496, -9.500000000000005329 ) ) ;
#2235=CARTESIAN_POINT ( 'NONE',  ( 4.622313124798831829, 18.56481371789855928, -11.61527771782809282 ) ) ;
#2237=CARTESIAN_POINT ( 'NONE',  ( -12.50000000000000355, 67.91018628210144925, -0.1745138560725492671 ) ) ;
#2245=CARTESIAN_POINT ( 'NONE',  ( -8.710071997420127943, 68.48518628210145209, -3.796722387233380402 ) ) ;
#2247=CARTESIAN_POINT ( 'NONE',  ( 2.311890736173175753, 111.3226862821014720, 12.53471296425194836 ) ) ;
#2260=CARTESIAN_POINT ( 'NONE',  ( -10.49813415416004858, 134.4273137178985849, 7.228626920338839135 ) ) ;
#2261=CARTESIAN_POINT ( 'NONE',  ( -10.69584247140444866, 140.6476862821014890, 6.932735513423972762 ) ) ;
#2269=CARTESIAN_POINT ( 'NONE',  ( 15.50000000000000533, 112.2898137178985678, -0.1745138560722452326 ) ) ;
#2275=CARTESIAN_POINT ( 'NONE',  ( -6.932735513423968321, 106.1476862821014606, -10.69584247140445221 ) ) ;
#2281=CARTESIAN_POINT ( 'NONE',  ( -0.1745138560725500443, 120.8101862821014691, 12.50000000000000355 ) ) ;
#2287=CARTESIAN_POINT ( 'NONE',  ( -3.257655550457281723, 111.8976862821014606, 15.46528703574804986 ) ) ;
#2288=CARTESIAN_POINT ( 'NONE',  ( -4.944772684328673229, 10.98518628210143433, 11.48171059495397728 ) ) ;
#2291=CARTESIAN_POINT ( 'NONE',  ( -7.954856959092191815, 123.9726862821014493, -5.529263428287477744 ) ) ;
#2296=CARTESIAN_POINT ( 'NONE',  ( 5.529263428287477744, 80.27268628210143220, -7.954856959092191815 ) ) ;
#2304=CARTESIAN_POINT ( 'NONE',  ( 1.715153634034445762, 55.07731371789854080, -9.534712964251895073 ) ) ;
#2306=AXIS2_PLACEMENT_3D ( 'NONE', #32116, #31750, #14880 ) ;
#2310=CARTESIAN_POINT ( 'NONE',  ( -12.53471296425189152, 71.17731371789855643, -2.311890736173453309 ) ) ;
#2313=CARTESIAN_POINT ( 'NONE',  ( -4.622313124798826500, 32.36481371789854933, 11.61527771782809637 ) ) ;
#2320=CARTESIAN_POINT ( 'NONE',  ( 8.715434833791931624, 9.260186282101429356, 8.962234695871760692 ) ) ;
#2328=AXIS2_PLACEMENT_3D ( 'NONE', #30872, #25550, #34270 ) ;
#2331=CARTESIAN_POINT ( 'NONE',  ( 15.53471296425188797, 38.97731371789853938, 2.908627838312457747 ) ) ;
#2333=CARTESIAN_POINT ( 'NONE',  ( -12.46528703574805697, 12.99768628210143362, -2.660918448318280838 ) ) ;
#2334=CARTESIAN_POINT ( 'NONE',  ( 11.48171059495397728, 63.88518628210145067, 4.944772684328674117 ) ) ;
#2335=CARTESIAN_POINT ( 'NONE',  ( -13.04141134922759804, 13.57268628210145422, -8.927990412390657937 ) ) ;
#2339=CARTESIAN_POINT ( 'NONE',  ( -14.38691631536207183, 21.33518628210144641, 5.770363421893814682 ) ) ;
#2345=CARTESIAN_POINT ( 'NONE',  ( 8.962234695871762469, 6.960186282101432198, -8.715434833791931624 ) ) ;
#2347=CARTESIAN_POINT ( 'NONE',  ( -5.233372021372612259, 106.2523137178985451, 8.152565276336593669 ) ) ;
#2352=CARTESIAN_POINT ( 'NONE',  ( -0.1745138560722763466, 119.1898137178985593, -12.50000000000000355 ) ) ;
#2365=CARTESIAN_POINT ( 'NONE',  ( 12.53471296425194836, 53.82268628210144357, -2.311890736173178418 ) ) ;
#2371=CARTESIAN_POINT ( 'NONE',  ( 8.962234695871567070, 122.6398137178985621, 8.715434833792127023 ) ) ;
#2376=CARTESIAN_POINT ( 'NONE',  ( -11.08355503943118592, 90.43981371789854506, -10.83675517735179383 ) ) ;
#2380=CARTESIAN_POINT ( 'NONE',  ( -12.50000000000000355, 113.9101862821014493, -0.1745138560725492671 ) ) ;
#2382=CARTESIAN_POINT ( 'NONE',  ( 13.04141134922759804, 73.37268628210144072, 8.927990412390657937 ) ) ;
#2385=CARTESIAN_POINT ( 'NONE',  ( 10.83675517735155225, 82.86018628210146630, 11.08355503943142573 ) ) ;
#2387=CARTESIAN_POINT ( 'NONE',  ( 0.1745138560725194299, 24.21018628210144996, -9.500000000000005329 ) ) ;
#2391=CARTESIAN_POINT ( 'NONE',  ( -0.1745138560725500443, 56.41018628210145636, 12.50000000000000355 ) ) ;
#2394=CARTESIAN_POINT ( 'NONE',  ( 2.064181346179272847, 24.49768628210144072, -9.465287035748065847 ) ) ;
#2405=CARTESIAN_POINT ( 'NONE',  ( -2.660918448318275509, 93.49768628210145494, 12.46528703574805874 ) ) ;
#2410=CARTESIAN_POINT ( 'NONE',  ( 14.38691631536194393, 30.06481371789855572, 5.770363421894124656 ) ) ;
#2417=CARTESIAN_POINT ( 'NONE',  ( 8.152565276336593669, 30.35231371789855359, 5.233372021372610483 ) ) ;
#2420=CARTESIAN_POINT ( 'NONE',  ( 7.954856959092311719, 102.2273137178985678, -5.529263428287300108 ) ) ;
#2422=CARTESIAN_POINT ( 'NONE',  ( 0.1745138560722461762, 142.1898137178985451, 15.50000000000000533 ) ) ;
#2423=CARTESIAN_POINT ( 'NONE',  ( 10.69584247140445221, 71.64768628210146062, -6.932735513423970097 ) ) ;
#2425=DIRECTION ( 'NONE',  ( 0.000000000000000000, -0.000000000000000000, 1.000000000000000000 ) ) ;
#2431=CARTESIAN_POINT ( 'NONE',  ( 0.1745138560725194299, 79.41018628210144925, -9.500000000000005329 ) ) ;
#2433=CARTESIAN_POINT ( 'NONE',  ( 8.715434833791931624, 110.4601862821014606, 8.962234695871760692 ) ) ;
#2446=CARTESIAN_POINT ( 'NONE',  ( -12.50000000000000355, 116.8898137178985621, 0.1745138560722786503 ) ) ;
#2447=CARTESIAN_POINT ( 'NONE',  ( 11.61527771782819940, 136.3351862821014606, -4.622313124798573369 ) ) ;
#2454=CARTESIAN_POINT ( 'NONE',  ( -5.770363421894122880, 105.9648137178985650, 14.38691631536194393 ) ) ;
#2459=CARTESIAN_POINT ( 'NONE',  ( -7.228626920339069173, 112.4726862821014493, 10.49813415415989581 ) ) ;
#2466=CARTESIAN_POINT ( 'NONE',  ( -2.660918448318275509, 121.0976862821014635, 12.46528703574805874 ) ) ;
#2472=CARTESIAN_POINT ( 'NONE',  ( -11.08355503943142573, 103.5601862821014407, 10.83675517735155402 ) ) ;
#2473=CARTESIAN_POINT ( 'NONE',  ( -2.311890736173176641, 14.72268628210143859, -12.53471296425194659 ) ) ;
#2476=CARTESIAN_POINT ( 'NONE',  ( -8.152565276336710909, 140.6476862821014322, 5.233372021372435512 ) ) ;
#2481=CARTESIAN_POINT ( 'NONE',  ( 1.715153634034233487, 65.32268628210144357, 9.534712964251941258 ) ) ;
#2486=DIRECTION ( 'NONE',  ( 1.047113545471812582E-14, 0.1163425707149433608, -0.9932091452657082487 ) ) ;
#2487=CARTESIAN_POINT ( 'NONE',  ( -8.710071997420207879, 33.51481371789854791, 3.796722387233182339 ) ) ;
#2491=CARTESIAN_POINT ( 'NONE',  ( -10.49813415416004858, 60.82731371789855501, 7.228626920338840023 ) ) ;
#2494=CARTESIAN_POINT ( 'NONE',  ( -2.311890736173448424, 32.07731371789855501, 12.53471296425189330 ) ) ;
#2498=CARTESIAN_POINT ( 'NONE',  ( -12.53471296425194836, 12.42268628210144321, 2.311890736173176641 ) ) ;
#2513=CARTESIAN_POINT ( 'NONE',  ( 14.25334919248795451, 19.71481371789854720, -6.092822981423661410 ) ) ;
#2515=CARTESIAN_POINT ( 'NONE',  ( 1.715153634034233487, 138.9226862821014663, 9.534712964251941258 ) ) ;
#2518=CARTESIAN_POINT ( 'NONE',  ( -6.932735513423968321, 41.74768628210144783, -10.69584247140445221 ) ) ;
#2523=CARTESIAN_POINT ( 'NONE',  ( -11.61527771782819940, 140.9351862821014834, 4.622313124798574258 ) ) ;
#2533=CARTESIAN_POINT ( 'NONE',  ( 5.233372021372610483, 110.8523137178985252, -8.152565276336593669 ) ) ;
#2539=CARTESIAN_POINT ( 'NONE',  ( -8.962234695871565293, 118.0398137178985678, -8.715434833792128799 ) ) ;
#2552=CARTESIAN_POINT ( 'NONE',  ( -10.69584247140444866, 57.84768628210144925, 6.932735513423972762 ) ) ;
#2557=CARTESIAN_POINT ( 'NONE',  ( 2.311890736173452865, 110.2773137178985650, -12.53471296425189152 ) ) ;
#2562=CARTESIAN_POINT ( 'NONE',  ( -2.908627838312453306, 87.27731371789855075, 15.53471296425188797 ) ) ;
#2566=CARTESIAN_POINT ( 'NONE',  ( 12.46528703574805874, 100.3976862821014464, 2.660918448318279950 ) ) ;
#2567=CARTESIAN_POINT ( 'NONE',  ( 15.46528703574804986, 72.79768628210145209, 3.257655550457285720 ) ) ;
#2570=CARTESIAN_POINT ( 'NONE',  ( -5.770363421893818234, 60.43518628210146204, -14.38691631536207005 ) ) ;
#2573=CARTESIAN_POINT ( 'NONE',  ( 1.715153634034233487, 19.32268628210144001, 9.534712964251941258 ) ) ;
#2578=CARTESIAN_POINT ( 'NONE',  ( -6.932735513423968321, 50.94768628210144357, -10.69584247140445221 ) ) ;
#2580=CARTESIAN_POINT ( 'NONE',  ( 8.710071997420127943, 17.88518628210143646, 3.796722387233375073 ) ) ;
#2590=CARTESIAN_POINT ( 'NONE',  ( 2.660918448318279950, 61.29768628210144499, -12.46528703574805874 ) ) ;
#2595=CARTESIAN_POINT ( 'NONE',  ( -13.23911966647199812, 34.95231371789854080, -8.632099005475788900 ) ) ;
#2601=CARTESIAN_POINT ( 'NONE',  ( -7.954856959092309943, 42.42731371789855643, 5.529263428287300108 ) ) ;
#2605=CARTESIAN_POINT ( 'NONE',  ( -0.1745138560722763466, 17.98981371789853867, -12.50000000000000355 ) ) ;
#2607=CARTESIAN_POINT ( 'NONE',  ( 10.49813415415989581, 64.17268628210143788, 7.228626920339068285 ) ) ;
#2614=CARTESIAN_POINT ( 'NONE',  ( 9.500000000000005329, 81.71018628210144641, 0.1745138560725188748 ) ) ;
#2616=CARTESIAN_POINT ( 'NONE',  ( -10.49813415415989581, 105.5726862821014578, -7.228626920339068285 ) ) ;
#2628=CARTESIAN_POINT ( 'NONE',  ( 0.1745138560722779009, 114.5898137178985650, 12.50000000000000355 ) ) ;
#2629=CARTESIAN_POINT ( 'NONE',  ( -11.61527771782819940, 122.5351862821014635, 4.622313124798574258 ) ) ;
#2634=CARTESIAN_POINT ( 'NONE',  ( 13.04141134922778988, 93.02731371789853654, -8.927990412390371944 ) ) ;
#2635=CARTESIAN_POINT ( 'NONE',  ( 12.53471296425194836, 90.62268628210146915, -2.311890736173178418 ) ) ;
#2640=CARTESIAN_POINT ( 'NONE',  ( -12.50000000000000355, 113.9101862821014493, -0.1745138560725492671 ) ) ;
#2646=CARTESIAN_POINT ( 'NONE',  ( -12.50000000000000355, 113.9101862821014493, -0.1745138560725492671 ) ) ;
#2651=CARTESIAN_POINT ( 'NONE',  ( -13.04141134922759804, 96.37268628210144072, -8.927990412390657937 ) ) ;
#2653=CARTESIAN_POINT ( 'NONE',  ( -6.932735513423968321, 23.34768628210144570, -10.69584247140445221 ) ) ;
#2656=CARTESIAN_POINT ( 'NONE',  ( -2.064181346179269738, 139.4976862821014549, 9.465287035748067623 ) ) ;
#2662=CARTESIAN_POINT ( 'NONE',  ( 6.840914352312096547, 62.16018628210144925, -6.594114490232313663 ) ) ;
#2671=CARTESIAN_POINT ( 'NONE',  ( -8.152565276336593669, 34.95231371789854080, -5.233372021372610483 ) ) ;
#2676=CARTESIAN_POINT ( 'NONE',  ( 2.311890736173452421, 45.87731371789855217, -12.53471296425189152 ) ) ;
#2679=CARTESIAN_POINT ( 'NONE',  ( -11.48171059495408208, 15.11481371789855110, 4.944772684328421875 ) ) ;
#2682=CARTESIAN_POINT ( 'NONE',  ( -12.50000000000000355, 3.510186282101451560, -0.1745138560725492671 ) ) ;
#2695=CARTESIAN_POINT ( 'NONE',  ( 10.83675517735179206, 28.33981371789855430, -11.08355503943118769 ) ) ;
#2697=CARTESIAN_POINT ( 'NONE',  ( -12.50000000000000355, 12.71018628210143753, -0.1745138560725492671 ) ) ;
#2698=CARTESIAN_POINT ( 'NONE',  ( -12.53471296425194836, 40.02268628210143930, 2.311890736173176641 ) ) ;
#2709=CARTESIAN_POINT ( 'NONE',  ( -8.152565276336593669, 99.35231371789856780, -5.233372021372610483 ) ) ;
#2716=CARTESIAN_POINT ( 'NONE',  ( -0.1745138560722763466, 109.9898137178985706, -12.50000000000000355 ) ) ;
#2721=CARTESIAN_POINT ( 'NONE',  ( 4.944772684328420986, 58.81481371789855217, 11.48171059495408208 ) ) ;
#2731=CARTESIAN_POINT ( 'NONE',  ( -7.228626920339069173, 57.27268628210144641, 10.49813415415989581 ) ) ;
#2739=CARTESIAN_POINT ( 'NONE',  ( -12.46528703574811558, 98.20231371789856212, 2.660918448318003726 ) ) ;
#2743=CARTESIAN_POINT ( 'NONE',  ( 15.53471296425188797, 84.97731371789856780, 2.908627838312457747 ) ) ;
#2748=CARTESIAN_POINT ( 'NONE',  ( 10.69584247140445221, 108.4476862821014578, -6.932735513423970097 ) ) ;
#2749=CARTESIAN_POINT ( 'NONE',  ( -6.092822981423970496, 38.58518628210143930, 14.25334919248782661 ) ) ;
#2754=CARTESIAN_POINT ( 'NONE',  ( -15.53471296425195369, 58.42268628210145209, 2.908627838312118019 ) ) ;
#2759=CARTESIAN_POINT ( 'NONE',  ( -12.46528703574805697, 40.59768628210144215, -2.660918448318280838 ) ) ;
#2762=CARTESIAN_POINT ( 'NONE',  ( -8.710071997420127943, 13.28518628210143149, -3.796722387233380402 ) ) ;
#2773=CARTESIAN_POINT ( 'NONE',  ( -4.622313124798576922, 69.63518628210145778, -11.61527771782819762 ) ) ;
#2779=CARTESIAN_POINT ( 'NONE',  ( -13.23911966647199812, 44.15231371789854364, -8.632099005475788900 ) ) ;
#2786=CARTESIAN_POINT ( 'NONE',  ( 6.840914352311949109, 12.23981371789853512, 6.594114490232462877 ) ) ;
#2791=CARTESIAN_POINT ( 'NONE',  ( -8.927990412390371944, 127.5273137178985792, -13.04141134922778988 ) ) ;
#2795=CARTESIAN_POINT ( 'NONE',  ( -0.1745138560725500443, 38.01018628210144357, 12.50000000000000355 ) ) ;
#2802=CARTESIAN_POINT ( 'NONE',  ( 7.954856959092191815, 73.37268628210144072, 5.529263428287477744 ) ) ;
#2805=CARTESIAN_POINT ( 'NONE',  ( 12.50000000000000355, 90.91018628210146346, 0.1745138560725507937 ) ) ;
#2817=CARTESIAN_POINT ( 'NONE',  ( 8.715434833792128799, 120.3398137178985650, -8.962234695871567070 ) ) ;
#2818=CARTESIAN_POINT ( 'NONE',  ( -4.622313124798576922, 124.8351862821014748, -11.61527771782819762 ) ) ;
#2824=CARTESIAN_POINT ( 'NONE',  ( -10.83675517735179028, 97.33981371789856496, 11.08355503943118947 ) ) ;
#2827=CARTESIAN_POINT ( 'NONE',  ( 5.529263428287300108, 76.92731371789854222, 7.954856959092309943 ) ) ;
#2830=CARTESIAN_POINT ( 'NONE',  ( -10.49813415416004858, 70.02731371789855075, 7.228626920338839135 ) ) ;
#2833=CARTESIAN_POINT ( 'NONE',  ( -0.1745138560725500443, 111.6101862821014521, 12.50000000000000355 ) ) ;
#2838=CARTESIAN_POINT ( 'NONE',  ( -15.50000000000000533, 95.51018628210147199, -0.1745138560725808530 ) ) ;
#2840=CARTESIAN_POINT ( 'NONE',  ( 2.311890736173175753, 10.12268628210144428, 12.53471296425194659 ) ) ;
#2843=CARTESIAN_POINT ( 'NONE',  ( 9.534712964251941258, 127.4226862821014521, -1.715153634034235708 ) ) ;
#2847=CARTESIAN_POINT ( 'NONE',  ( -3.474262827703337830, 60.43518628210146204, -8.843639120294326972 ) ) ;
#2854=CARTESIAN_POINT ( 'NONE',  ( -2.064181346179062349, 36.10231371789854649, -9.465287035748106703 ) ) ;
#2859=CARTESIAN_POINT ( 'NONE',  ( -4.622313124798826500, 41.56481371789855217, 11.61527771782809637 ) ) ;
#2862=CARTESIAN_POINT ( 'NONE',  ( -15.50000000000000533, 144.4898137178985280, 0.1745138560722471477 ) ) ;
#2878=CARTESIAN_POINT ( 'NONE',  ( -11.08355503943118592, 26.03981371789855714, -10.83675517735179383 ) ) ;
#2881=CARTESIAN_POINT ( 'NONE',  ( -10.49813415415989581, 4.372686282101440725, -7.228626920339068285 ) ) ;
#2882=CARTESIAN_POINT ( 'NONE',  ( 0.1745138560725515708, 51.81018628210144783, -12.50000000000000355 ) ) ;
#2894=CARTESIAN_POINT ( 'NONE',  ( -8.843639120294245259, 89.86481371789855643, -3.474262827703533230 ) ) ;
#2902=CARTESIAN_POINT ( 'NONE',  ( 4.944772684328420986, 95.61481371789857064, 11.48171059495408208 ) ) ;
#2907=CARTESIAN_POINT ( 'NONE',  ( -12.46528703574811558, 70.60231371789856780, 2.660918448318003726 ) ) ;
#2917=CARTESIAN_POINT ( 'NONE',  ( 2.311890736173175753, 46.92268628210145209, 12.53471296425194836 ) ) ;
#2923=CARTESIAN_POINT ( 'NONE',  ( -12.50000000000000355, 98.48981371789855643, 0.1745138560722786503 ) ) ;
#2929=CARTESIAN_POINT ( 'NONE',  ( 13.23911966647199812, 85.55231371789855643, 8.632099005475788900 ) ) ;
#2933=CARTESIAN_POINT ( 'NONE',  ( -4.622313124798576922, 106.4351862821014549, -11.61527771782819762 ) ) ;
#2934=CARTESIAN_POINT ( 'NONE',  ( 14.25334919248782661, 54.68518628210145494, 6.092822981423971385 ) ) ;
#2937=CARTESIAN_POINT ( 'NONE',  ( -14.25334919248782306, 68.48518628210145209, -6.092822981423979378 ) ) ;
#2944=CARTESIAN_POINT ( 'NONE',  ( 10.49813415415989581, 45.77268628210144641, 7.228626920339068285 ) ) ;
#2947=CARTESIAN_POINT ( 'NONE',  ( -1.715153634034442431, 142.4773137178985678, 9.534712964251900402 ) ) ;
#2958=CARTESIAN_POINT ( 'NONE',  ( -12.53471296425194659, 76.82268628210145778, 2.311890736173176641 ) ) ;
#2966=CARTESIAN_POINT ( 'NONE',  ( -15.53471296425188442, 34.37731371789854506, -2.908627838312459080 ) ) ;
#2972=CARTESIAN_POINT ( 'NONE',  ( 8.710071997420211432, 28.91481371789854649, -3.796722387233181895 ) ) ;
#2978=CARTESIAN_POINT ( 'NONE',  ( 13.04141134922778988, 129.8273137178985905, -8.927990412390371944 ) ) ;
#2982=CARTESIAN_POINT ( 'NONE',  ( -10.69584247140444866, 39.44768628210145067, 6.932735513423972762 ) ) ;
#2989=CARTESIAN_POINT ( 'NONE',  ( -5.233372021372430183, 69.34768628210143504, -8.152565276336710909 ) ) ;
#2993=CARTESIAN_POINT ( 'NONE',  ( -12.46528703574805697, 86.59768628210144925, -2.660918448318280838 ) ) ;
#3004=CARTESIAN_POINT ( 'NONE',  ( 8.962234695871567070, 113.4398137178985593, 8.715434833792127023 ) ) ;
#3006=CARTESIAN_POINT ( 'NONE',  ( 6.932735513423970097, 129.1476862821014890, 10.69584247140445044 ) ) ;
#3011=CARTESIAN_POINT ( 'NONE',  ( 3.257655550456945548, 95.90231371789855075, 15.46528703574811736 ) ) ;
#3016=CARTESIAN_POINT ( 'NONE',  ( 8.152565276336593669, 76.35231371789853938, 5.233372021372610483 ) ) ;
#3019=CARTESIAN_POINT ( 'NONE',  ( -2.660918448318004614, 45.30231371789855643, -12.46528703574811558 ) ) ;
#3022=CARTESIAN_POINT ( 'NONE',  ( -4.944772684328673229, 93.78518628210144925, 11.48171059495397728 ) ) ;
#3027=CARTESIAN_POINT ( 'NONE',  ( -0.1745138560725817967, 93.21018628210146062, 15.50000000000000533 ) ) ;
#3028=CARTESIAN_POINT ( 'NONE',  ( 7.228626920339069173, 6.672686282101436106, -10.49813415415989404 ) ) ;
#3031=CARTESIAN_POINT ( 'NONE',  ( -5.529263428287477744, 130.8726862821014834, 7.954856959092191815 ) ) ;
#3037=CARTESIAN_POINT ( 'NONE',  ( 3.474262827703335166, 55.83518628210145351, 8.843639120294326972 ) ) ;
#3040=DIRECTION ( 'NONE',  ( 0.000000000000000000, -0.9932091452657081376, -0.1163425707149433747 ) ) ;
#3045=CARTESIAN_POINT ( 'NONE',  ( 3.474262827703532341, 46.16481371789854649, -8.843639120294245259 ) ) ;
#3050=CARTESIAN_POINT ( 'NONE',  ( -2.660918448318005058, 36.10231371789854649, -12.46528703574811558 ) ) ;
#3053=CARTESIAN_POINT ( 'NONE',  ( -0.1745138560722763466, 17.98981371789853867, -12.50000000000000355 ) ) ;
#3069=CARTESIAN_POINT ( 'NONE',  ( -0.1745138560722442889, 17.98981371789853867, -15.50000000000000533 ) ) ;
#3071=CARTESIAN_POINT ( 'NONE',  ( 0.1745138560725515708, 5.810186282101447830, -12.50000000000000355 ) ) ;
#3072=CARTESIAN_POINT ( 'NONE',  ( 8.715434833791931624, 46.06018628210144072, 8.962234695871760692 ) ) ;
#3084=CARTESIAN_POINT ( 'NONE',  ( -8.152565276336593669, 90.15231371789855075, -5.233372021372610483 ) ) ;
#3091=CARTESIAN_POINT ( 'NONE',  ( 12.53471296425189330, 103.3773137178985593, 2.311890736173451533 ) ) ;
#3095=CARTESIAN_POINT ( 'NONE',  ( 8.715434833792128799, 74.33981371789855075, -8.962234695871567070 ) ) ;
#3103=CARTESIAN_POINT ( 'NONE',  ( 12.50000000000000355, 44.91018628210144215, 0.1745138560725507937 ) ) ;
#3111=CARTESIAN_POINT ( 'NONE',  ( -8.715434833792127023, 106.5398137178985536, 8.962234695871568846 ) ) ;
#3116=CARTESIAN_POINT ( 'NONE',  ( 15.46528703574811736, 84.40231371789855075, -3.257655550456947768 ) ) ;
#3120=CARTESIAN_POINT ( 'NONE',  ( -8.962234695871760692, 103.5601862821014549, 8.715434833791933400 ) ) ;
#3121=CARTESIAN_POINT ( 'NONE',  ( 10.83675517735155225, 55.26018628210144357, 11.08355503943142573 ) ) ;
#3124=CARTESIAN_POINT ( 'NONE',  ( 6.092822981423978490, 70.78518628210143504, -14.25334919248782306 ) ) ;
#3131=CARTESIAN_POINT ( 'NONE',  ( 8.715434833791931624, 36.86018628210144499, 8.962234695871760692 ) ) ;
#3134=CARTESIAN_POINT ( 'NONE',  ( 0.1745138560725194299, 15.01018628210143291, -9.500000000000005329 ) ) ;
#3145=CARTESIAN_POINT ( 'NONE',  ( -8.962234695871760692, 75.96018628210144641, 8.715434833791933400 ) ) ;
#3153=CARTESIAN_POINT ( 'NONE',  ( -15.50000000000000533, 34.08981371789853654, 0.1745138560722471477 ) ) ;
#3159=CARTESIAN_POINT ( 'NONE',  ( 6.840914352311949109, 21.43981371789854506, 6.594114490232462877 ) ) ;
#3164=CARTESIAN_POINT ( 'NONE',  ( 3.257655550456945548, 132.7023137178985337, 15.46528703574811736 ) ) ;
#3166=CARTESIAN_POINT ( 'NONE',  ( 4.944772684328679446, 52.38518628210145067, -11.48171059495397373 ) ) ;
#3173=CARTESIAN_POINT ( 'NONE',  ( 5.529263428287477744, 61.87268628210144783, -7.954856959092191815 ) ) ;
#3176=CARTESIAN_POINT ( 'NONE',  ( 12.53471296425194836, 90.62268628210146915, -2.311890736173178418 ) ) ;
#3188=CARTESIAN_POINT ( 'NONE',  ( 2.660918448318002838, 114.3023137178985564, 12.46528703574811558 ) ) ;
#3189=CARTESIAN_POINT ( 'NONE',  ( 4.944772684328679446, 116.7851862821014635, -11.48171059495397373 ) ) ;
#3194=CARTESIAN_POINT ( 'NONE',  ( 0.1745138560722461762, 86.98981371789857064, 15.50000000000000533 ) ) ;
#3201=CARTESIAN_POINT ( 'NONE',  ( -5.233372021372612259, 78.65231371789856496, 8.152565276336593669 ) ) ;
#3205=CARTESIAN_POINT ( 'NONE',  ( -11.48171059495408208, 42.71481371789855075, 4.944772684328421875 ) ) ;
#3209=CARTESIAN_POINT ( 'NONE',  ( 6.932735513423970097, 92.34768628210144925, 10.69584247140445044 ) ) ;
#3215=CARTESIAN_POINT ( 'NONE',  ( 8.632099005475504683, 92.34768628210142083, 13.23911966647218996 ) ) ;
#3218=CARTESIAN_POINT ( 'NONE',  ( -5.233372021372430183, 115.3476862821014493, -8.152565276336710909 ) ) ;
#3220=CARTESIAN_POINT ( 'NONE',  ( -0.1745138560725817967, 19.61018628210144144, 15.50000000000000533 ) ) ;
#3225=CARTESIAN_POINT ( 'NONE',  ( -7.954856959092191815, 68.77268628210143220, -5.529263428287477744 ) ) ;
#3232=CARTESIAN_POINT ( 'NONE',  ( 6.840914352311949109, 39.83981371789855075, 6.594114490232462877 ) ) ;
#3237=CARTESIAN_POINT ( 'NONE',  ( 12.50000000000000355, 47.88981371789854791, -0.1745138560722771515 ) ) ;
#3240=CARTESIAN_POINT ( 'NONE',  ( 11.48171059495408208, 19.71481371789854364, -4.944772684328420986 ) ) ;
#3256=CARTESIAN_POINT ( 'NONE',  ( -15.50000000000000533, 15.68981371789854329, 0.1745138560722471477 ) ) ;
#3260=CARTESIAN_POINT ( 'NONE',  ( -3.796722387233375073, 130.5851862821014606, 8.710071997420127943 ) ) ;
#3261=CARTESIAN_POINT ( 'NONE',  ( -11.48171059495397373, 40.88518628210144357, -4.944772684328680334 ) ) ;
#3267=CARTESIAN_POINT ( 'NONE',  ( -8.152565276336710909, 30.24768628210144783, 5.233372021372435512 ) ) ;
#3273=CARTESIAN_POINT ( 'NONE',  ( 6.594114490232462877, 92.73981371789854222, -6.840914352311949109 ) ) ;
#3278=CARTESIAN_POINT ( 'NONE',  ( 11.48171059495408208, 93.31481371789855928, -4.944772684328420986 ) ) ;
#3283=CARTESIAN_POINT ( 'NONE',  ( 12.50000000000000355, 66.28981371789855359, -0.1745138560722771515 ) ) ;
#3291=CARTESIAN_POINT ( 'NONE',  ( -0.1745138560725500443, 47.21018628210143930, 12.50000000000000355 ) ) ;
#3296=CARTESIAN_POINT ( 'NONE',  ( 8.715434833792128799, 101.9398137178985593, -8.962234695871567070 ) ) ;
#3302=CARTESIAN_POINT ( 'NONE',  ( -0.1745138560722442889, 73.18981371789854506, -15.50000000000000533 ) ) ;
#3306=CARTESIAN_POINT ( 'NONE',  ( 2.660918448318279950, 98.09768628210146346, -12.46528703574805697 ) ) ;
#3307=CARTESIAN_POINT ( 'NONE',  ( -5.770363421893818234, 42.03518628210144925, -14.38691631536207005 ) ) ;
#3310=CARTESIAN_POINT ( 'NONE',  ( 10.83675517735155225, 64.46018628210146062, 11.08355503943142573 ) ) ;
#3317=CARTESIAN_POINT ( 'NONE',  ( 11.61527771782819940, 35.13518628210143646, -4.622313124798573369 ) ) ;
#3320=CARTESIAN_POINT ( 'NONE',  ( 1.715153634034233487, 10.12268628210144428, 9.534712964251941258 ) ) ;
#3330=CARTESIAN_POINT ( 'NONE',  ( 6.932735513423970097, 46.34768628210144925, 10.69584247140445044 ) ) ;
#3337=CARTESIAN_POINT ( 'NONE',  ( -12.50000000000000355, 86.31018628210145494, -0.1745138560725492671 ) ) ;
#3338=CARTESIAN_POINT ( 'NONE',  ( -11.08355503943118592, 26.03981371789855714, -10.83675517735179383 ) ) ;
#3346=CARTESIAN_POINT ( 'NONE',  ( 5.233372021372610483, 18.85231371789855359, -8.152565276336593669 ) ) ;
#3353=CARTESIAN_POINT ( 'NONE',  ( 14.38691631536194393, 140.4648137178985507, 5.770363421894124656 ) ) ;
#3356=CARTESIAN_POINT ( 'NONE',  ( -4.622313124798576922, 51.23518628210143788, -11.61527771782819762 ) ) ;
#3363=CARTESIAN_POINT ( 'NONE',  ( -6.594114490232312775, 50.66018628210144925, -6.840914352312096547 ) ) ;
#3366=CARTESIAN_POINT ( 'NONE',  ( 11.61527771782819940, 90.33518628210144641, -4.622313124798573369 ) ) ;
#3370=AXIS2_PLACEMENT_3D ( 'NONE', #21253, #9114, #3040 ) ;
#3380=CARTESIAN_POINT ( 'NONE',  ( 0.1745138560722779009, 105.3898137178985621, 12.50000000000000355 ) ) ;
#3381=CARTESIAN_POINT ( 'NONE',  ( -10.49813415415989404, 114.7726862821014606, -7.228626920339069173 ) ) ;
#3387=CARTESIAN_POINT ( 'NONE',  ( 8.632099005475788900, 83.25231371789854506, -13.23911966647199812 ) ) ;
#3390=CARTESIAN_POINT ( 'NONE',  ( -5.529263428287477744, 103.2726862821014322, 7.954856959092191815 ) ) ;
#3393=CARTESIAN_POINT ( 'NONE',  ( 1.715153634034445762, 82.67731371789852801, -9.534712964251895073 ) ) ;
#3396=CARTESIAN_POINT ( 'NONE',  ( -2.311890736173448424, 50.47731371789855359, 12.53471296425189330 ) ) ;
#3398=CARTESIAN_POINT ( 'NONE',  ( -0.1745138560725500443, 102.4101862821014493, 12.50000000000000355 ) ) ;
#3404=CARTESIAN_POINT ( 'NONE',  ( 13.04141134922759804, 82.57268628210144357, 8.927990412390657937 ) ) ;
#3407=CARTESIAN_POINT ( 'NONE',  ( 1.715153634034233487, 111.3226862821014578, 9.534712964251941258 ) ) ;
#3409=CARTESIAN_POINT ( 'NONE',  ( 8.927990412390657937, 15.87268628210144605, -13.04141134922759804 ) ) ;
#3421=CARTESIAN_POINT ( 'NONE',  ( -6.594114490232462877, 14.53981371789855892, 6.840914352311949109 ) ) ;
#3425=CARTESIAN_POINT ( 'NONE',  ( -10.49813415416004858, 51.62731371789855217, 7.228626920338840023 ) ) ;
#3427=CARTESIAN_POINT ( 'NONE',  ( -4.944772684328424539, 8.214813717898532985, -11.48171059495408031 ) ) ;
#3443=CARTESIAN_POINT ( 'NONE',  ( 15.46528703574804986, 137.1976862821014436, 3.257655550457285720 ) ) ;
#3445=CARTESIAN_POINT ( 'NONE',  ( -6.840914352312096547, 121.9601862821014606, 6.594114490232313663 ) ) ;
#3447=CARTESIAN_POINT ( 'NONE',  ( 2.660918448318279950, 24.49768628210144783, -12.46528703574805697 ) ) ;
#3452=CARTESIAN_POINT ( 'NONE',  ( 11.08355503943142750, 126.5601862821014834, -10.83675517735155225 ) ) ;
#3455=CARTESIAN_POINT ( 'NONE',  ( 0.1745138560725194299, 5.810186282101448718, -9.500000000000005329 ) ) ;
#3462=CARTESIAN_POINT ( 'NONE',  ( -1.715153634034442431, 87.27731371789855075, 9.534712964251900402 ) ) ;
#3469=CARTESIAN_POINT ( 'NONE',  ( -4.944772684328424539, 100.2148137178985650, -11.48171059495408031 ) ) ;
#3473=CARTESIAN_POINT ( 'NONE',  ( -2.311890736173448424, 59.67731371789855643, 12.53471296425189330 ) ) ;
#3480=CARTESIAN_POINT ( 'NONE',  ( 10.69584247140445221, 34.84768628210143504, -6.932735513423970097 ) ) ;
#3485=CARTESIAN_POINT ( 'NONE',  ( -11.61527771782809282, 89.86481371789855643, -4.622313124798832717 ) ) ;
#3490=CARTESIAN_POINT ( 'NONE',  ( 10.83675517735179206, 74.33981371789855075, -11.08355503943118769 ) ) ;
#3493=CARTESIAN_POINT ( 'NONE',  ( 2.660918448318279950, 79.69768628210144357, -12.46528703574805697 ) ) ;
#3494=CARTESIAN_POINT ( 'NONE',  ( 15.50000000000000533, 44.91018628210144215, 0.1745138560725827404 ) ) ;
#3499=CARTESIAN_POINT ( 'NONE',  ( 15.50000000000000533, 54.11018628210144499, 0.1745138560725827404 ) ) ;
#3506=CARTESIAN_POINT ( 'NONE',  ( -11.48171059495397373, 31.68518628210144428, -4.944772684328680334 ) ) ;
#3508=CARTESIAN_POINT ( 'NONE',  ( -9.465287035748106703, 144.2023137178985905, 2.064181346179061460 ) ) ;
#3520=CARTESIAN_POINT ( 'NONE',  ( -12.50000000000000355, 58.71018628210145351, -0.1745138560725492671 ) ) ;
#3529=CARTESIAN_POINT ( 'NONE',  ( 11.61527771782819940, 99.53518628210144925, -4.622313124798573369 ) ) ;
#3530=CARTESIAN_POINT ( 'NONE',  ( 13.04141134922778988, 28.62731371789854506, -8.927990412390371944 ) ) ;
#3537=CARTESIAN_POINT ( 'NONE',  ( -4.622313124798826500, 142.7648137178985621, 11.61527771782809637 ) ) ;
#3545=CARTESIAN_POINT ( 'NONE',  ( 15.46528703574811736, 139.6023137178985394, -3.257655550456947768 ) ) ;
#3548=CARTESIAN_POINT ( 'NONE',  ( 12.46528703574805874, 54.39768628210146062, 2.660918448318279950 ) ) ;
#3551=AXIS2_PLACEMENT_3D ( 'NONE', #7751, #19885, #2425 ) ;
#3553=CARTESIAN_POINT ( 'NONE',  ( 15.53471296425195369, 109.0226862821014606, -2.908627838312120684 ) ) ;
#3556=CARTESIAN_POINT ( 'NONE',  ( -7.954856959092191815, 50.37268628210144783, -5.529263428287477744 ) ) ;
#3560=CARTESIAN_POINT ( 'NONE',  ( 12.50000000000000355, 100.1101862821014521, 0.1745138560725507937 ) ) ;
#3573=CARTESIAN_POINT ( 'NONE',  ( 2.660918448318002838, 95.90231371789856496, 12.46528703574811558 ) ) ;
#3574=CARTESIAN_POINT ( 'NONE',  ( -11.61527771782819940, 113.3351862821014606, 4.622313124798574258 ) ) ;
#3578=CARTESIAN_POINT ( 'NONE',  ( -14.38691631536193860, 80.66481371789856780, -5.770363421894132649 ) ) ;
#3581=CARTESIAN_POINT ( 'NONE',  ( -6.594114490232312775, 105.8601862821014379, -6.840914352312096547 ) ) ;
#3583=CARTESIAN_POINT ( 'NONE',  ( -3.796722387233185003, 72.61481371789855643, -8.710071997420207879 ) ) ;
#3586=CARTESIAN_POINT ( 'NONE',  ( -9.534712964251895073, 107.9773137178985394, -1.715153634034446428 ) ) ;
#3588=CARTESIAN_POINT ( 'NONE',  ( -11.61527771782809282, 53.06481371789854506, -4.622313124798832717 ) ) ;
#3590=CARTESIAN_POINT ( 'NONE',  ( 12.46528703574805874, 100.3976862821014464, 2.660918448318279950 ) ) ;
#3593=CARTESIAN_POINT ( 'NONE',  ( -11.61527771782819940, 140.9351862821014834, 4.622313124798574258 ) ) ;
#3595=CARTESIAN_POINT ( 'NONE',  ( -10.83675517735155047, 87.46018628210146062, -11.08355503943142750 ) ) ;
#3599=CARTESIAN_POINT ( 'NONE',  ( 7.954856959092191815, 110.1726862821014663, 5.529263428287477744 ) ) ;
#3601=CARTESIAN_POINT ( 'NONE',  ( -3.257655550457281723, 10.69768628210143646, 15.46528703574804986 ) ) ;
#3613=CARTESIAN_POINT ( 'NONE',  ( 0.1745138560723095977, 22.58981371789854364, 9.500000000000005329 ) ) ;
#3618=CARTESIAN_POINT ( 'NONE',  ( 0.1745138560722779009, 22.58981371789854720, 12.50000000000000355 ) ) ;
#3620=CARTESIAN_POINT ( 'NONE',  ( 8.927990412390371944, 132.1273137178985735, 13.04141134922778811 ) ) ;
#3628=SURFACE_STYLE_FILL_AREA ( #29208 ) ;
#3636=CARTESIAN_POINT ( 'NONE',  ( 11.08355503943142750, 135.7601862821014720, -10.83675517735155225 ) ) ;
#3638=CARTESIAN_POINT ( 'NONE',  ( 9.534712964251941258, 127.4226862821014521, -1.715153634034235708 ) ) ;
#3640=CARTESIAN_POINT ( 'NONE',  ( -10.69584247140444866, 30.24768628210144783, 6.932735513423972762 ) ) ;
#3644=CARTESIAN_POINT ( 'NONE',  ( 2.908627838312118019, 120.5226862821014322, 15.53471296425195369 ) ) ;
#3646=CARTESIAN_POINT ( 'NONE',  ( -8.843639120294326972, 12.13518628210144712, 3.474262827703335166 ) ) ;
#3652=CARTESIAN_POINT ( 'NONE',  ( 5.233372021372610483, 83.25231371789854506, -8.152565276336593669 ) ) ;
#3656=CARTESIAN_POINT ( 'NONE',  ( 11.61527771782809637, 103.6648137178985678, 4.622313124798827388 ) ) ;
#3660=CARTESIAN_POINT ( 'NONE',  ( 7.228626920338837358, 40.12731371789853796, 10.49813415416005036 ) ) ;
#3668=CARTESIAN_POINT ( 'NONE',  ( -11.48171059495397373, 31.68518628210144428, -4.944772684328680334 ) ) ;
#3674=CARTESIAN_POINT ( 'NONE',  ( -12.50000000000000355, 80.08981371789855075, 0.1745138560722786503 ) ) ;
#3681=CARTESIAN_POINT ( 'NONE',  ( -2.908627838312453306, 59.67731371789855643, 15.53471296425188797 ) ) ;
#3684=CARTESIAN_POINT ( 'NONE',  ( -0.1745138560725500443, 93.21018628210146062, 12.50000000000000355 ) ) ;
#3685=CARTESIAN_POINT ( 'NONE',  ( 13.04141134922759804, 27.37268628210144428, 8.927990412390657937 ) ) ;
#3689=CARTESIAN_POINT ( 'NONE',  ( -8.927990412390661490, 48.07268628210143646, 13.04141134922759804 ) ) ;
#3694=CARTESIAN_POINT ( 'NONE',  ( 0.1745138560725515708, 15.01018628210143468, -12.50000000000000355 ) ) ;
#3696=CARTESIAN_POINT ( 'NONE',  ( 5.529263428287300108, 122.9273137178985422, 7.954856959092309943 ) ) ;
#3705=CARTESIAN_POINT ( 'NONE',  ( -12.53471296425194659, 49.22268628210144215, 2.311890736173176641 ) ) ;
#3713=CARTESIAN_POINT ( 'NONE',  ( -6.932735513423968321, 87.74768628210145494, -10.69584247140445221 ) ) ;
#3714=CARTESIAN_POINT ( 'NONE',  ( 15.46528703574811736, 20.00231371789855217, -3.257655550456947768 ) ) ;
#3720=CARTESIAN_POINT ( 'NONE',  ( 7.228626920338837358, 132.1273137178986019, 10.49813415416005036 ) ) ;
#3725=CARTESIAN_POINT ( 'NONE',  ( 13.04141134922778988, 111.4273137178985422, -8.927990412390371944 ) ) ;
#3729=CARTESIAN_POINT ( 'NONE',  ( 2.311890736173175753, 28.52268628210144641, 12.53471296425194836 ) ) ;
#3733=CARTESIAN_POINT ( 'NONE',  ( -3.257655550457281723, 102.6976862821014294, 15.46528703574804986 ) ) ;
#3736=CARTESIAN_POINT ( 'NONE',  ( 9.465287035748067623, 54.39768628210144641, 2.064181346179272847 ) ) ;
#3739=CARTESIAN_POINT ( 'NONE',  ( -8.962234695871760692, 75.96018628210144641, 8.715434833791933400 ) ) ;
#3752=CARTESIAN_POINT ( 'NONE',  ( 4.622313124798831829, 101.3648137178985564, -11.61527771782809282 ) ) ;
#3753=CARTESIAN_POINT ( 'NONE',  ( -4.622313124798576922, 106.4351862821014549, -11.61527771782819762 ) ) ;
#3758=CARTESIAN_POINT ( 'NONE',  ( 10.83675517735179206, 74.33981371789855075, -11.08355503943118769 ) ) ;
#3761=CARTESIAN_POINT ( 'NONE',  ( 9.534712964251941258, 90.62268628210145494, -1.715153634034235708 ) ) ;
#3764=CARTESIAN_POINT ( 'NONE',  ( -5.529263428287297444, 63.12731371789852375, -7.954856959092311719 ) ) ;
#3766=CARTESIAN_POINT ( 'NONE',  ( 3.474262827703532341, 119.7648137178985905, -8.843639120294245259 ) ) ;
#3768=CARTESIAN_POINT ( 'NONE',  ( -11.61527771782809282, 43.86481371789854933, -4.622313124798832717 ) ) ;
#3770=CARTESIAN_POINT ( 'NONE',  ( -6.932735513423968321, 96.94768628210145778, -10.69584247140445221 ) ) ;
#3775=CARTESIAN_POINT ( 'NONE',  ( 2.908627838312118019, 83.72268628210143504, 15.53471296425195369 ) ) ;
#3779=CARTESIAN_POINT ( 'NONE',  ( -8.710071997420127943, 114.4851862821014663, -3.796722387233380402 ) ) ;
#3781=CARTESIAN_POINT ( 'NONE',  ( -15.50000000000000533, 3.510186282101451560, -0.1745138560725808530 ) ) ;
#3792=CARTESIAN_POINT ( 'NONE',  ( 7.954856959092311719, 19.42731371789854933, -5.529263428287300108 ) ) ;
#3797=CARTESIAN_POINT ( 'NONE',  ( 11.61527771782809637, 20.86481371789854222, 4.622313124798827388 ) ) ;
#3799=CARTESIAN_POINT ( 'NONE',  ( 14.25334919248795451, 139.3148137178985451, -6.092822981423661410 ) ) ;
#3807=CARTESIAN_POINT ( 'NONE',  ( -12.46528703574805697, 132.5976862821014777, -2.660918448318280838 ) ) ;
#3811=( NAMED_UNIT ( * ) SI_UNIT ( $, .STERADIAN. ) SOLID_ANGLE_UNIT ( ) );
#3819=CARTESIAN_POINT ( 'NONE',  ( -14.38691631536193860, 7.064813717898548617, -5.770363421894132649 ) ) ;
#3823=CARTESIAN_POINT ( 'NONE',  ( -0.1745138560725182642, 130.0101862821014436, 9.500000000000005329 ) ) ;
#3825=CARTESIAN_POINT ( 'NONE',  ( -0.1745138560725500443, 38.01018628210144357, 12.50000000000000355 ) ) ;
#3829=CARTESIAN_POINT ( 'NONE',  ( -13.23911966647218463, 122.2476862821014691, 8.632099005475506459 ) ) ;
#3832=CARTESIAN_POINT ( 'NONE',  ( 0.1745138560723095977, 142.1898137178985451, 9.500000000000005329 ) ) ;
#3838=CARTESIAN_POINT ( 'NONE',  ( 6.840914352311949109, 67.43981371789855928, 6.594114490232462877 ) ) ;
#3842=CARTESIAN_POINT ( 'NONE',  ( 10.49813415416005213, 74.62731371789855928, -7.228626920338837358 ) ) ;
#3847=CARTESIAN_POINT ( 'NONE',  ( 12.50000000000000355, 57.08981371789855075, -0.1745138560722771515 ) ) ;
#3853=CARTESIAN_POINT ( 'NONE',  ( 10.69584247140445221, 25.64768628210143930, -6.932735513423970097 ) ) ;
#3859=MECHANICAL_DESIGN_GEOMETRIC_PRESENTATION_REPRESENTATION('',(#825),#27462);
#3861=CARTESIAN_POINT ( 'NONE',  ( 10.49813415416005213, 93.02731371789856496, -7.228626920338837358 ) ) ;
#3867=CARTESIAN_POINT ( 'NONE',  ( -14.38691631536193860, 62.26481371789854791, -5.770363421894132649 ) ) ;
#3870=CARTESIAN_POINT ( 'NONE',  ( -12.50000000000000355, 86.31018628210145494, -0.1745138560725492671 ) ) ;
#3871=CARTESIAN_POINT ( 'NONE',  ( 3.257655550457285720, 33.69768628210143646, -15.46528703574804986 ) ) ;
#3874=CARTESIAN_POINT ( 'NONE',  ( -11.08355503943142573, 57.56018628210145494, 10.83675517735155402 ) ) ;
#3880=CARTESIAN_POINT ( 'NONE',  ( 6.932735513423970097, 27.94768628210143646, 10.69584247140445044 ) ) ;
#3882=CARTESIAN_POINT ( 'NONE',  ( -0.1745138560723084320, 128.3898137178985621, -9.500000000000005329 ) ) ;
#3889=CARTESIAN_POINT ( 'NONE',  ( -4.622313124798826500, 133.5648137178985735, 11.61527771782809637 ) ) ;
#3895=CARTESIAN_POINT ( 'NONE',  ( 2.660918448318279950, 52.09768628210144215, -12.46528703574805874 ) ) ;
#3902=CARTESIAN_POINT ( 'NONE',  ( -11.48171059495397373, 86.88518628210145778, -4.944772684328680334 ) ) ;
#3903=CARTESIAN_POINT ( 'NONE',  ( 8.927990412390371944, 21.72731371789853938, 13.04141134922778811 ) ) ;
#3909=CARTESIAN_POINT ( 'NONE',  ( -5.529263428287297444, 7.927313717898536005, -7.954856959092311719 ) ) ;
#3915=CARTESIAN_POINT ( 'NONE',  ( -15.53471296425188442, 107.9773137178985394, -2.908627838312459080 ) ) ;
#3918=CARTESIAN_POINT ( 'NONE',  ( -6.932735513423968321, 32.54768628210144499, -10.69584247140445221 ) ) ;
#3922=CARTESIAN_POINT ( 'NONE',  ( 8.632099005475504683, 101.5476862821014663, 13.23911966647218996 ) ) ;
#3925=CARTESIAN_POINT ( 'NONE',  ( -3.474262827703337830, 51.23518628210143788, -8.843639120294326972 ) ) ;
#3930=CARTESIAN_POINT ( 'NONE',  ( 10.49813415415989581, 73.37268628210144072, 7.228626920339068285 ) ) ;
#3933=CARTESIAN_POINT ( 'NONE',  ( 9.534712964251941258, 44.62268628210144783, -1.715153634034235708 ) ) ;
#3942=CARTESIAN_POINT ( 'NONE',  ( 4.944772684328420986, 104.8148137178985593, 11.48171059495408208 ) ) ;
#3943=CARTESIAN_POINT ( 'NONE',  ( 12.46528703574805874, 109.5976862821014493, 2.660918448318279950 ) ) ;
#3948=CARTESIAN_POINT ( 'NONE',  ( 8.927990412390371944, 76.92731371789854222, 13.04141134922778811 ) ) ;
#3952=CARTESIAN_POINT ( 'NONE',  ( 6.840914352312096547, 98.96018628210144641, -6.594114490232313663 ) ) ;
#3954=CARTESIAN_POINT ( 'NONE',  ( 8.710071997420211432, 56.51481371789856212, -3.796722387233181895 ) ) ;
#3957=CARTESIAN_POINT ( 'NONE',  ( -6.840914352311947333, 118.0398137178985536, -6.594114490232462877 ) ) ;
#3959=CARTESIAN_POINT ( 'NONE',  ( -2.311890736173448424, 32.07731371789855501, 12.53471296425189330 ) ) ;
#3961=CARTESIAN_POINT ( 'NONE',  ( -7.228626920339069173, 75.67268628210146630, 10.49813415415989581 ) ) ;
#3969=CARTESIAN_POINT ( 'NONE',  ( -7.954856959092191815, 105.5726862821014294, -5.529263428287477744 ) ) ;
#3972=CARTESIAN_POINT ( 'NONE',  ( -6.932735513423968321, 133.7476862821014549, -10.69584247140445221 ) ) ;
#3983=CARTESIAN_POINT ( 'NONE',  ( -8.843639120294245259, 16.26481371789853370, -3.474262827703533230 ) ) ;
#3988=CARTESIAN_POINT ( 'NONE',  ( -10.69584247140429412, 16.55231371789855999, -6.932735513424201024 ) ) ;
#3990=CARTESIAN_POINT ( 'NONE',  ( -13.04141134922778456, 125.2273137178985394, 8.927990412390377273 ) ) ;
#3997=CARTESIAN_POINT ( 'NONE',  ( 4.944772684328679446, 125.9851862821014521, -11.48171059495397373 ) ) ;
#4009=CARTESIAN_POINT ( 'NONE',  ( -13.23911966647218463, 140.6476862821014322, 8.632099005475506459 ) ) ;
#4013=CARTESIAN_POINT ( 'NONE',  ( -5.233372021372430183, 124.5476862821014663, -8.152565276336710909 ) ) ;
#4015=CARTESIAN_POINT ( 'NONE',  ( -4.944772684328673229, 29.38518628210144712, 11.48171059495397728 ) ) ;
#4017=UNCERTAINTY_MEASURE_WITH_UNIT (LENGTH_MEASURE( 1.000000000000000082E-05 ), #8757, 'distance_accuracy_value', 'NONE');
#4020=CARTESIAN_POINT ( 'NONE',  ( 15.53471296425195369, 127.4226862821014521, -2.908627838312120684 ) ) ;
#4022=CARTESIAN_POINT ( 'NONE',  ( 8.152565276336593669, 140.7523137178985166, 5.233372021372610483 ) ) ;
#4029=CARTESIAN_POINT ( 'NONE',  ( 8.710071997420211432, 84.11481371789855643, -3.796722387233181895 ) ) ;
#4032=CARTESIAN_POINT ( 'NONE',  ( -8.715434833792127023, 78.93981371789855928, 8.962234695871568846 ) ) ;
#4036=CARTESIAN_POINT ( 'NONE',  ( -11.61527771782809282, 53.06481371789854506, -4.622313124798832717 ) ) ;
#4042=CARTESIAN_POINT ( 'NONE',  ( 4.944772684328679446, 15.58518628210145351, -11.48171059495397373 ) ) ;
#4047=CARTESIAN_POINT ( 'NONE',  ( 4.622313124798831829, 92.16481371789855359, -11.61527771782809282 ) ) ;
#4052=CARTESIAN_POINT ( 'NONE',  ( -13.04141134922778456, 51.62731371789855928, 8.927990412390377273 ) ) ;
#4057=CARTESIAN_POINT ( 'NONE',  ( 6.932735513423970097, 83.14768628210144641, 10.69584247140445044 ) ) ;
#4058=CARTESIAN_POINT ( 'NONE',  ( -13.23911966647218463, 30.24768628210144783, 8.632099005475506459 ) ) ;
#4062=CARTESIAN_POINT ( 'NONE',  ( -2.908627838312119351, 51.52268628210144641, -15.53471296425195369 ) ) ;
#4070=CARTESIAN_POINT ( 'NONE',  ( 2.311890736173175753, 28.52268628210144641, 12.53471296425194836 ) ) ;
#4072=CARTESIAN_POINT ( 'NONE',  ( 0.1745138560723095977, 132.9898137178985564, 9.500000000000005329 ) ) ;
#4078=CARTESIAN_POINT ( 'NONE',  ( 12.50000000000000355, 130.6898137178985735, -0.1745138560722771515 ) ) ;
#4084=CARTESIAN_POINT ( 'NONE',  ( -8.715434833791929847, 50.66018628210144925, -8.962234695871762469 ) ) ;
#4092=CARTESIAN_POINT ( 'NONE',  ( -8.962234695871760692, 75.96018628210144641, 8.715434833791933400 ) ) ;
#4093=CARTESIAN_POINT ( 'NONE',  ( -13.04141134922778456, 14.82731371789855324, 8.927990412390377273 ) ) ;
#4100=CARTESIAN_POINT ( 'NONE',  ( 9.465287035748106703, 10.80231371789855466, -2.064181346179063237 ) ) ;
#4106=CARTESIAN_POINT ( 'NONE',  ( -13.23911966647199812, 117.7523137178985735, -8.632099005475788900 ) ) ;
#4110=CARTESIAN_POINT ( 'NONE',  ( -2.660918448318275509, 29.09768628210144925, 12.46528703574805874 ) ) ;
#4114=CARTESIAN_POINT ( 'NONE',  ( -2.908627838312119351, 106.7226862821014635, -15.53471296425195369 ) ) ;
#4117=CARTESIAN_POINT ( 'NONE',  ( -5.529263428287477744, 38.87268628210144072, 7.954856959092191815 ) ) ;
#4121=CARTESIAN_POINT ( 'NONE',  ( 12.46528703574805874, 72.79768628210146630, 2.660918448318279950 ) ) ;
#4124=CARTESIAN_POINT ( 'NONE',  ( -5.233372021372430183, 50.94768628210145067, -8.152565276336710909 ) ) ;
#4135=CARTESIAN_POINT ( 'NONE',  ( -10.69584247140429412, 99.35231371789855359, -6.932735513424201024 ) ) ;
#4136=CARTESIAN_POINT ( 'NONE',  ( 11.48171059495397728, 109.8851862821014436, 4.944772684328674117 ) ) ;
#4141=CARTESIAN_POINT ( 'NONE',  ( 14.38691631536194393, 76.06481371789855928, 5.770363421894124656 ) ) ;
#4144=CARTESIAN_POINT ( 'NONE',  ( -5.529263428287477744, 94.07268628210144357, 7.954856959092191815 ) ) ;
#4146=CARTESIAN_POINT ( 'NONE',  ( -9.500000000000005329, 52.48981371789855643, 0.1745138560723101806 ) ) ;
#4150=CARTESIAN_POINT ( 'NONE',  ( 8.710071997420211432, 111.7148137178985792, -3.796722387233181895 ) ) ;
#4152=CARTESIAN_POINT ( 'NONE',  ( 12.53471296425189330, 29.77731371789854720, 2.311890736173451977 ) ) ;
#4153=CARTESIAN_POINT ( 'NONE',  ( -6.932735513423968321, 87.74768628210145494, -10.69584247140445221 ) ) ;
#4162=CARTESIAN_POINT ( 'NONE',  ( 9.465287035748067623, 91.19768628210145778, 2.064181346179272847 ) ) ;
#4164=CARTESIAN_POINT ( 'NONE',  ( 6.932735513423970097, 138.3476862821014493, 10.69584247140445044 ) ) ;
#4175=CARTESIAN_POINT ( 'NONE',  ( -5.233372021372612259, 23.45231371789854435, 8.152565276336593669 ) ) ;
#4180=CARTESIAN_POINT ( 'NONE',  ( 6.932735513424201024, 28.05231371789855643, -10.69584247140429412 ) ) ;
#4182=CARTESIAN_POINT ( 'NONE',  ( -14.38691631536193860, 135.8648137178985849, -5.770363421894132649 ) ) ;
#4189=CARTESIAN_POINT ( 'NONE',  ( -6.932735513423968321, 133.7476862821014549, -10.69584247140445221 ) ) ;
#4194=CARTESIAN_POINT ( 'NONE',  ( -11.61527771782819940, 131.7351862821014663, 4.622313124798574258 ) ) ;
#4199=CARTESIAN_POINT ( 'NONE',  ( -5.770363421893818234, 134.0351862821014493, -14.38691631536207005 ) ) ;
#4201=CARTESIAN_POINT ( 'NONE',  ( 3.474262827703335166, 111.0351862821014635, 8.843639120294326972 ) ) ;
#4203=CARTESIAN_POINT ( 'NONE',  ( 10.69584247140445221, 25.64768628210143930, -6.932735513423970097 ) ) ;
#4207=CARTESIAN_POINT ( 'NONE',  ( -15.50000000000000533, 113.9101862821014493, -0.1745138560725808530 ) ) ;
#4209=CARTESIAN_POINT ( 'NONE',  ( 8.843639120294328748, 7.535186282101451916, -3.474262827703334722 ) ) ;
#4215=CARTESIAN_POINT ( 'NONE',  ( -1.715153634034442431, 68.87731371789855928, 9.534712964251900402 ) ) ;
#4218=CARTESIAN_POINT ( 'NONE',  ( -8.962234695871565293, 81.23981371789855643, -8.715434833792128799 ) ) ;
#4220=CARTESIAN_POINT ( 'NONE',  ( -6.443006283225887643, 143.0000000000001421, 10.75771091796995726 ) ) ;
#4222=CARTESIAN_POINT ( 'NONE',  ( 10.49813415416005213, 47.02731371789855075, -7.228626920338837358 ) ) ;
#4227=CARTESIAN_POINT ( 'NONE',  ( 8.715434833791931624, 18.46018628210144286, 8.962234695871760692 ) ) ;
#4233=CARTESIAN_POINT ( 'NONE',  ( 6.932735513424201024, 92.45231371789856212, -10.69584247140429412 ) ) ;
#4238=CARTESIAN_POINT ( 'NONE',  ( 14.38691631536194393, 66.86481371789854222, 5.770363421894124656 ) ) ;
#4240=AXIS2_PLACEMENT_3D ( 'NONE', #34513, #2486, #34694 ) ;
#4242=CARTESIAN_POINT ( 'NONE',  ( -8.715434833791929847, 78.26018628210144357, -8.962234695871762469 ) ) ;
#4243=CARTESIAN_POINT ( 'NONE',  ( 8.632099005475504683, 18.74768628210143362, 13.23911966647218996 ) ) ;
#4248=CARTESIAN_POINT ( 'NONE',  ( -15.53471296425195369, 40.02268628210144641, 2.908627838312118019 ) ) ;
#4254=CARTESIAN_POINT ( 'NONE',  ( -7.228626920339069173, 20.47268628210144570, 10.49813415415989581 ) ) ;
#4256=CARTESIAN_POINT ( 'NONE',  ( 6.840914352311949109, 131.8398137178985792, 6.594114490232462877 ) ) ;
#4261=CARTESIAN_POINT ( 'NONE',  ( 8.962234695871567070, 131.8398137178985792, 8.715434833792127023 ) ) ;
#4268=CARTESIAN_POINT ( 'NONE',  ( 12.53471296425194659, 26.22268628210144925, -2.311890736173178418 ) ) ;
#4276=CARTESIAN_POINT ( 'NONE',  ( 2.660918448318279950, 79.69768628210144357, -12.46528703574805697 ) ) ;
#4277=CARTESIAN_POINT ( 'NONE',  ( -8.927990412390371944, 7.927313717898536005, -13.04141134922778988 ) ) ;
#4283=CARTESIAN_POINT ( 'NONE',  ( -2.311890736173448424, 142.4773137178985678, 12.53471296425189330 ) ) ;
#4290=CARTESIAN_POINT ( 'NONE',  ( 8.632099005475788900, 110.8523137178985252, -13.23911966647199812 ) ) ;
#4297=CARTESIAN_POINT ( 'NONE',  ( 3.257655550457285720, 107.2976862821014521, -15.46528703574804986 ) ) ;
#4300=CARTESIAN_POINT ( 'NONE',  ( 8.710071997420127943, 36.28518628210144215, 3.796722387233375073 ) ) ;
#4305=CARTESIAN_POINT ( 'NONE',  ( -0.1745138560725500443, 74.81018628210145494, 12.50000000000000355 ) ) ;
#4307=CARTESIAN_POINT ( 'NONE',  ( 6.594114490232313663, 46.06018628210144072, 6.840914352312096547 ) ) ;
#4317=CARTESIAN_POINT ( 'NONE',  ( -12.46528703574811558, 79.80231371789857064, 2.660918448318003726 ) ) ;
#4318=CARTESIAN_POINT ( 'NONE',  ( 2.311890736173175753, 102.1226862821014549, 12.53471296425194659 ) ) ;
#4324=CARTESIAN_POINT ( 'NONE',  ( -15.46528703574811736, 52.20231371789854080, 3.257655550456946436 ) ) ;
#4329=CARTESIAN_POINT ( 'NONE',  ( -7.954856959092309943, 51.62731371789855928, 5.529263428287300108 ) ) ;
#4331=CARTESIAN_POINT ( 'NONE',  ( 8.710071997420211432, 120.9148137178985678, -3.796722387233181895 ) ) ;
#4333=CARTESIAN_POINT ( 'NONE',  ( -8.715434833792127023, 32.93981371789854506, 8.962234695871568846 ) ) ;
#4335=CARTESIAN_POINT ( 'NONE',  ( 12.50000000000000355, 90.91018628210146346, 0.1745138560725507937 ) ) ;
#4343=CARTESIAN_POINT ( 'NONE',  ( 8.710071997420127943, 91.48518628210145209, 3.796722387233375073 ) ) ;
#4346=CARTESIAN_POINT ( 'NONE',  ( -10.49813415415989581, 133.1726862821014663, -7.228626920339068285 ) ) ;
#4357=CARTESIAN_POINT ( 'NONE',  ( -2.311890736173448424, 142.4773137178985678, 12.53471296425189330 ) ) ;
#4363=CARTESIAN_POINT ( 'NONE',  ( -10.49813415416004858, 33.22731371789855359, 7.228626920338840023 ) ) ;
#4366=CARTESIAN_POINT ( 'NONE',  ( 3.257655550456945548, 123.5023137178985451, 15.46528703574811736 ) ) ;
#4373=CARTESIAN_POINT ( 'NONE',  ( 2.311890736173175753, 129.7226862821014777, 12.53471296425194836 ) ) ;
#4381=CARTESIAN_POINT ( 'NONE',  ( -4.944772684328673229, 139.7851862821014493, 11.48171059495397728 ) ) ;
#4385=CARTESIAN_POINT ( 'NONE',  ( -15.53471296425195369, 113.6226862821014549, 2.908627838312118019 ) ) ;
#4387=CARTESIAN_POINT ( 'NONE',  ( -6.840914352312096547, 112.7601862821014720, 6.594114490232313663 ) ) ;
#4388=CARTESIAN_POINT ( 'NONE',  ( 2.311890736173175753, 19.32268628210144712, 12.53471296425194836 ) ) ;
#4392=CARTESIAN_POINT ( 'NONE',  ( 3.474262827703335166, 83.43518628210145494, 8.843639120294326972 ) ) ;
#4394=CARTESIAN_POINT ( 'NONE',  ( -9.465287035748106703, 135.0023137178985166, 2.064181346179061460 ) ) ;
#4401=CARTESIAN_POINT ( 'NONE',  ( 5.233372021372610483, 74.05231371789854222, -8.152565276336593669 ) ) ;
#4404=CARTESIAN_POINT ( 'NONE',  ( -7.228626920338836470, 81.52731371789856496, -10.49813415416005213 ) ) ;
#4406=CARTESIAN_POINT ( 'NONE',  ( -13.83312331854208743, 143.0000000000000000, 2.380703716050323049 ) ) ;
#4408=CARTESIAN_POINT ( 'NONE',  ( -7.228626920338836470, 44.72731371789855359, -10.49813415416005213 ) ) ;
#4413=CARTESIAN_POINT ( 'NONE',  ( -8.715434833791929847, 13.86018628210145032, -8.962234695871762469 ) ) ;
#4420=CARTESIAN_POINT ( 'NONE',  ( 2.311890736173452865, 64.27731371789855075, -12.53471296425189152 ) ) ;
#4425=CARTESIAN_POINT ( 'NONE',  ( -15.46528703574811736, 61.40231371789855785, 3.257655550456946436 ) ) ;
#4429=CARTESIAN_POINT ( 'NONE',  ( 8.962234695871762469, 71.36018628210145209, -8.715434833791931624 ) ) ;
#4430=CARTESIAN_POINT ( 'NONE',  ( 10.83675517735155225, 36.86018628210144499, 11.08355503943142573 ) ) ;
#4434=CARTESIAN_POINT ( 'NONE',  ( 8.927990412390657937, 34.27268628210144641, -13.04141134922759804 ) ) ;
#4440=CARTESIAN_POINT ( 'NONE',  ( 12.53471296425194836, 17.02268628210144996, -2.311890736173178418 ) ) ;
#4443=CARTESIAN_POINT ( 'NONE',  ( -3.474262827703527901, 133.5648137178985735, 8.843639120294245259 ) ) ;
#4447=CARTESIAN_POINT ( 'NONE',  ( 10.69584247140429589, 140.7523137178985735, 6.932735513424201024 ) ) ;
#4453=CARTESIAN_POINT ( 'NONE',  ( -6.932735513423968321, 32.54768628210144499, -10.69584247140445221 ) ) ;
#4463=CARTESIAN_POINT ( 'NONE',  ( 10.49813415415989581, 82.57268628210145778, 7.228626920339068285 ) ) ;
#4464=CARTESIAN_POINT ( 'NONE',  ( 15.53471296425188797, 11.37731371789854506, 2.908627838312457747 ) ) ;
#4470=CARTESIAN_POINT ( 'NONE',  ( -10.69584247140429412, 126.9523137178985621, -6.932735513424201024 ) ) ;
#4476=CARTESIAN_POINT ( 'NONE',  ( 15.50000000000000533, 112.2898137178985678, -0.1745138560722452326 ) ) ;
#4482=CARTESIAN_POINT ( 'NONE',  ( -0.1745138560725817967, 84.01018628210145778, 15.50000000000000533 ) ) ;
#4486=CARTESIAN_POINT ( 'NONE',  ( -15.50000000000000533, 77.11018628210145209, -0.1745138560725808530 ) ) ;
#4487=PRODUCT_DEFINITION_FORMATION_WITH_SPECIFIED_SOURCE ( 'ANY', '', #34976, .NOT_KNOWN. ) ;
#4490=CARTESIAN_POINT ( 'NONE',  ( -6.840914352312096547, 48.36018628210145209, 6.594114490232313663 ) ) ;
#4494=CARTESIAN_POINT ( 'NONE',  ( -12.46528703574805697, 77.39768628210144641, -2.660918448318280838 ) ) ;
#4497=CARTESIAN_POINT ( 'NONE',  ( -8.843639120294326972, 39.73518628210145209, 3.474262827703335166 ) ) ;
#4507=CARTESIAN_POINT ( 'NONE',  ( 12.53471296425189330, 75.77731371789855075, 2.311890736173451977 ) ) ;
#4508=CARTESIAN_POINT ( 'NONE',  ( -6.932735513423968321, 78.54768628210145209, -10.69584247140445221 ) ) ;
#4513=CARTESIAN_POINT ( 'NONE',  ( -15.50000000000000533, 61.68981371789855928, 0.1745138560722471477 ) ) ;
#4520=CARTESIAN_POINT ( 'NONE',  ( -8.152565276336593669, 53.35231371789856780, -5.233372021372610483 ) ) ;
#4522=CARTESIAN_POINT ( 'NONE',  ( 7.954856959092311719, 93.02731371789853654, -5.529263428287300108 ) ) ;
#4524=CARTESIAN_POINT ( 'NONE',  ( -4.944772684328424539, 26.61481371789854578, -11.48171059495408031 ) ) ;
#4525=CARTESIAN_POINT ( 'NONE',  ( -12.50000000000000355, 77.11018628210145209, -0.1745138560725492671 ) ) ;
#4533=CARTESIAN_POINT ( 'NONE',  ( -6.840914352312096547, 94.36018628210146630, 6.594114490232313663 ) ) ;
#4535=CARTESIAN_POINT ( 'NONE',  ( -2.660918448318275509, 130.2976862821014379, 12.46528703574805874 ) ) ;
#4548=CARTESIAN_POINT ( 'NONE',  ( -2.311890736173448424, 133.2773137178985507, 12.53471296425189330 ) ) ;
#4549=CARTESIAN_POINT ( 'NONE',  ( 12.50000000000000355, 136.9101862821014777, 0.1745138560725507937 ) ) ;
#4554=CARTESIAN_POINT ( 'NONE',  ( -2.660918448318005058, 8.502313717898557499, -12.46528703574811558 ) ) ;
#4556=CARTESIAN_POINT ( 'NONE',  ( 6.092822981423662299, 114.0148137178985763, 14.25334919248795096 ) ) ;
#4561=CARTESIAN_POINT ( 'NONE',  ( -11.61527771782819940, 131.7351862821014663, 4.622313124798574258 ) ) ;
#4575=CARTESIAN_POINT ( 'NONE',  ( -6.092822981423970496, 121.3851862821014578, 14.25334919248782661 ) ) ;
#4576=CARTESIAN_POINT ( 'NONE',  ( 0.1745138560725194299, 116.2101862821014748, -9.500000000000005329 ) ) ;
#4579=CARTESIAN_POINT ( 'NONE',  ( 8.715434833791931624, 18.46018628210144286, 8.962234695871760692 ) ) ;
#4583=CARTESIAN_POINT ( 'NONE',  ( -3.474262827703337830, 78.83518628210146062, -8.843639120294326972 ) ) ;
#4585=CARTESIAN_POINT ( 'NONE',  ( 0.1745138560723095977, 132.9898137178985564, 9.500000000000005329 ) ) ;
#4591=CARTESIAN_POINT ( 'NONE',  ( 8.843639120294245259, 57.66481371789855359, 3.474262827703527901 ) ) ;
#4594=CARTESIAN_POINT ( 'NONE',  ( 0.1745138560722779009, 86.98981371789855643, 12.50000000000000355 ) ) ;
#4598=CARTESIAN_POINT ( 'NONE',  ( -11.61527771782809282, 25.46481371789855075, -4.622313124798832717 ) ) ;
#4601=CARTESIAN_POINT ( 'NONE',  ( -7.228626920339069173, 20.47268628210144570, 10.49813415415989581 ) ) ;
#4605=CARTESIAN_POINT ( 'NONE',  ( -11.61527771782809282, 71.46481371789856496, -4.622313124798832717 ) ) ;
#4610=CARTESIAN_POINT ( 'NONE',  ( -6.092822981423666739, 45.01481371789854791, -14.25334919248795096 ) ) ;
#4614=CARTESIAN_POINT ( 'NONE',  ( -12.46528703574805697, 68.19768628210144357, -2.660918448318280838 ) ) ;
#4616=CARTESIAN_POINT ( 'NONE',  ( 8.927990412390657937, 15.87268628210144605, -13.04141134922759804 ) ) ;
#4617=MECHANICAL_DESIGN_GEOMETRIC_PRESENTATION_REPRESENTATION('',(#24602),#31250);
#4621=CARTESIAN_POINT ( 'NONE',  ( -15.46528703574804986, 22.19768628210144001, -3.257655550457287497 ) ) ;
#4626=CARTESIAN_POINT ( 'NONE',  ( -10.49813415415989581, 4.372686282101440725, -7.228626920339068285 ) ) ;
#4628=CARTESIAN_POINT ( 'NONE',  ( 8.152565276336593669, 103.9523137178985763, 5.233372021372610483 ) ) ;
#4633=CARTESIAN_POINT ( 'NONE',  ( -5.558451987054219501, 142.8813032066705944, 11.24274018108063267 ) ) ;
#4639=CARTESIAN_POINT ( 'NONE',  ( -12.53471296425194659, 40.02268628210143930, 2.311890736173176641 ) ) ;
#4646=CARTESIAN_POINT ( 'NONE',  ( 4.944772684328679446, 79.98518628210145209, -11.48171059495397373 ) ) ;
#4647=CARTESIAN_POINT ( 'NONE',  ( -8.927990412390661490, 140.0726862821014151, 13.04141134922759804 ) ) ;
#4651=DIRECTION ( 'NONE',  ( 0.000000000000000000, 0.000000000000000000, 1.000000000000000000 ) ) ;
#4653=CARTESIAN_POINT ( 'NONE',  ( -12.53471296425189152, 117.1773137178985564, -2.311890736173453753 ) ) ;
#4658=CARTESIAN_POINT ( 'NONE',  ( 14.38691631536194393, 103.6648137178985678, 5.770363421894124656 ) ) ;
#4663=CARTESIAN_POINT ( 'NONE',  ( -7.228626920339069173, 130.8726862821014834, 10.49813415415989581 ) ) ;
#4664=CARTESIAN_POINT ( 'NONE',  ( -8.927990412390661490, 75.67268628210143788, 13.04141134922759804 ) ) ;
#4667=CARTESIAN_POINT ( 'NONE',  ( -13.23911966647218463, 76.24768628210145494, 8.632099005475506459 ) ) ;
#4670=CARTESIAN_POINT ( 'NONE',  ( -7.954856959092191815, 31.97268628210143149, -5.529263428287477744 ) ) ;
#4675=CARTESIAN_POINT ( 'NONE',  ( -8.962234695871760692, 66.76018628210145778, 8.715434833791933400 ) ) ;
#4678=CARTESIAN_POINT ( 'NONE',  ( -8.710071997420127943, 50.08518628210143930, -3.796722387233380402 ) ) ;
#4688=CARTESIAN_POINT ( 'NONE',  ( -4.944772684328424539, 91.01481371789856212, -11.48171059495408031 ) ) ;
#4689=CARTESIAN_POINT ( 'NONE',  ( 12.53471296425194659, 90.62268628210145494, -2.311890736173178418 ) ) ;
#4695=CARTESIAN_POINT ( 'NONE',  ( -10.83675517735179028, 60.53981371789856070, 11.08355503943118947 ) ) ;
#4702=CARTESIAN_POINT ( 'NONE',  ( 9.500000000000005329, 38.68981371789855217, -0.1745138560723090149 ) ) ;
#4704=CARTESIAN_POINT ( 'NONE',  ( 6.594114490232462877, 92.73981371789854222, -6.840914352311949109 ) ) ;
#4706=CARTESIAN_POINT ( 'NONE',  ( -6.932735513424201912, 14.25231371789853441, 10.69584247140429412 ) ) ;
#4707=CARTESIAN_POINT ( 'NONE',  ( 4.622313124798573369, 74.23518628210145209, 11.61527771782819940 ) ) ;
#4716=CARTESIAN_POINT ( 'NONE',  ( 1.715153634034233487, 102.1226862821014549, 9.534712964251941258 ) ) ;
#4719=CARTESIAN_POINT ( 'NONE',  ( 12.46528703574805874, 109.5976862821014493, 2.660918448318279950 ) ) ;
#4733=CARTESIAN_POINT ( 'NONE',  ( -6.840914352311947333, 7.639813717898540801, -6.594114490232462877 ) ) ;
#4738=CARTESIAN_POINT ( 'NONE',  ( 8.715434833792128799, 9.939813717898537959, -8.962234695871567070 ) ) ;
#4740=CARTESIAN_POINT ( 'NONE',  ( 2.908627838312458636, 110.2773137178985650, -15.53471296425188442 ) ) ;
#4749=CARTESIAN_POINT ( 'NONE',  ( 10.69584247140445221, 108.4476862821014578, -6.932735513423970097 ) ) ;
#4760=CARTESIAN_POINT ( 'NONE',  ( -5.770363421893818234, 124.8351862821014748, -14.38691631536207005 ) ) ;
#4763=CARTESIAN_POINT ( 'NONE',  ( -2.311890736173176641, 5.522686282101451738, -12.53471296425194836 ) ) ;
#4768=CARTESIAN_POINT ( 'NONE',  ( -9.465287035748065847, 77.39768628210144641, -2.064181346179273735 ) ) ;
#4770=CARTESIAN_POINT ( 'NONE',  ( 3.796722387233182339, 123.2148137178985792, 8.710071997420207879 ) ) ;
#4776=CARTESIAN_POINT ( 'NONE',  ( 7.954856959092311719, 56.22731371789854649, -5.529263428287300108 ) ) ;
#4780=CARTESIAN_POINT ( 'NONE',  ( 8.715434833792128799, 55.93981371789855217, -8.962234695871567070 ) ) ;
#4784=CARTESIAN_POINT ( 'NONE',  ( -8.715434833792127023, 32.93981371789854506, 8.962234695871568846 ) ) ;
#4788=CARTESIAN_POINT ( 'NONE',  ( -8.962234695871760692, 11.56018628210145316, 8.715434833791933400 ) ) ;
#4792=CARTESIAN_POINT ( 'NONE',  ( 11.48171059495408208, 65.71481371789855075, -4.944772684328420986 ) ) ;
#4797=CARTESIAN_POINT ( 'NONE',  ( -15.50000000000000533, 34.08981371789853654, 0.1745138560722471477 ) ) ;
#4799=CARTESIAN_POINT ( 'NONE',  ( -12.53471296425194836, 30.82268628210144001, 2.311890736173176641 ) ) ;
#4801=CARTESIAN_POINT ( 'NONE',  ( -4.944772684328673229, 66.18518628210144072, 11.48171059495397728 ) ) ;
#4802=CARTESIAN_POINT ( 'NONE',  ( 3.257655550457285720, 6.097686282101443922, -15.46528703574804986 ) ) ;
#4806=CARTESIAN_POINT ( 'NONE',  ( 6.092822981423978490, 33.98518628210143788, -14.25334919248782306 ) ) ;
#4812=CARTESIAN_POINT ( 'NONE',  ( -7.228626920339069173, 11.27268628210143042, 10.49813415415989581 ) ) ;
#4814=CARTESIAN_POINT ( 'NONE',  ( -1.715153634034442431, 105.6773137178985706, 9.534712964251900402 ) ) ;
#4818=CARTESIAN_POINT ( 'NONE',  ( 6.932735513424201024, 120.0523137178985706, -10.69584247140429412 ) ) ;
#4824=CARTESIAN_POINT ( 'NONE',  ( 8.715434833791931624, 27.66018628210144215, 8.962234695871760692 ) ) ;
#4832=CARTESIAN_POINT ( 'NONE',  ( 11.61527771782819940, 81.13518628210145778, -4.622313124798573369 ) ) ;
#4834=CARTESIAN_POINT ( 'NONE',  ( -6.092822981423666739, 8.214813717898532985, -14.25334919248795096 ) ) ;
#4841=CARTESIAN_POINT ( 'NONE',  ( 7.228626920338837358, 122.9273137178985422, 10.49813415416005036 ) ) ;
#4847=CARTESIAN_POINT ( 'NONE',  ( 13.04141134922778988, 93.02731371789853654, -8.927990412390371944 ) ) ;
#4851=CARTESIAN_POINT ( 'NONE',  ( 8.962234695871762469, 126.5601862821014691, -8.715434833791931624 ) ) ;
#4852=CARTESIAN_POINT ( 'NONE',  ( 14.38691631536207538, 71.93518628210142651, -5.770363421893813793 ) ) ;
#4856=CARTESIAN_POINT ( 'NONE',  ( 13.23911966647218996, 90.04768628210145209, -8.632099005475504683 ) ) ;
#4859=CARTESIAN_POINT ( 'NONE',  ( 8.843639120294328748, 44.33518628210144641, -3.474262827703334722 ) ) ;
#4863=CARTESIAN_POINT ( 'NONE',  ( 12.46528703574805874, 54.39768628210146062, 2.660918448318279950 ) ) ;
#4866=CARTESIAN_POINT ( 'NONE',  ( 8.152565276336714462, 25.64768628210144286, -5.233372021372432847 ) ) ;
#4877=CARTESIAN_POINT ( 'NONE',  ( 2.311890736173452865, 82.67731371789855643, -12.53471296425189152 ) ) ;
#4878=CARTESIAN_POINT ( 'NONE',  ( 12.50000000000000355, 90.91018628210146346, 0.1745138560725507937 ) ) ;
#4883=CARTESIAN_POINT ( 'NONE',  ( 15.53471296425188797, 57.37731371789855928, 2.908627838312457747 ) ) ;
#4888=CARTESIAN_POINT ( 'NONE',  ( -2.064181346179062349, 36.10231371789854649, -9.465287035748106703 ) ) ;
#4890=CARTESIAN_POINT ( 'NONE',  ( 8.710071997420211432, 102.5148137178985621, -3.796722387233181895 ) ) ;
#4892=CARTESIAN_POINT ( 'NONE',  ( -10.69584247140429412, 16.55231371789855999, -6.932735513424201024 ) ) ;
#4893=CARTESIAN_POINT ( 'NONE',  ( -2.660918448318275509, 65.89768628210146062, 12.46528703574805874 ) ) ;
#4895=FACE_OUTER_BOUND ( 'NONE', #21258, .T. ) ;
#4900=CARTESIAN_POINT ( 'NONE',  ( 6.594114490232313663, 101.2601862821014436, 6.840914352312096547 ) ) ;
#4902=CARTESIAN_POINT ( 'NONE',  ( 11.48171059495397728, 119.0851862821014606, 4.944772684328674117 ) ) ;
#4903=CARTESIAN_POINT ( 'NONE',  ( -9.195083260712237916, 143.0000000000000000, 6.638546685473677655 ) ) ;
#4915=CARTESIAN_POINT ( 'NONE',  ( 8.715434833792128799, 138.7398137178985564, -8.962234695871567070 ) ) ;
#4916=CARTESIAN_POINT ( 'NONE',  ( -7.228626920339070061, 140.0726862821014436, 10.49813415415989404 ) ) ;
#4920=CARTESIAN_POINT ( 'NONE',  ( 10.49813415416005213, 10.22731371789853405, -7.228626920338837358 ) ) ;
#4922=CARTESIAN_POINT ( 'NONE',  ( 8.632099005475788900, 120.0523137178985280, -13.23911966647199812 ) ) ;
#4928=CARTESIAN_POINT ( 'NONE',  ( -12.46528703574805697, 114.1976862821014720, -2.660918448318280838 ) ) ;
#4934=CARTESIAN_POINT ( 'NONE',  ( 10.49813415415989581, 119.3726862821014549, 7.228626920339068285 ) ) ;
#4938=CARTESIAN_POINT ( 'NONE',  ( 11.08355503943142750, 117.3601862821014663, -10.83675517735155225 ) ) ;
#4941=CARTESIAN_POINT ( 'NONE',  ( 4.622313124798573369, 19.03518628210144925, 11.61527771782819940 ) ) ;
#4946=CARTESIAN_POINT ( 'NONE',  ( 8.152565276336714462, 80.84768628210143504, -5.233372021372432847 ) ) ;
#4948=CARTESIAN_POINT ( 'NONE',  ( -2.064181346179062349, 128.1023137178985678, -9.465287035748106703 ) ) ;
#4955=CARTESIAN_POINT ( 'NONE',  ( 6.594114490232462877, 65.13981371789854791, -6.840914352311949109 ) ) ;
#4960=CARTESIAN_POINT ( 'NONE',  ( -12.50000000000000355, 70.88981371789856212, 0.1745138560722786503 ) ) ;
#4964=CARTESIAN_POINT ( 'NONE',  ( 10.69584247140429589, 30.35231371789855359, 6.932735513424201024 ) ) ;
#4975=CARTESIAN_POINT ( 'NONE',  ( 2.660918448318002838, 59.10231371789854649, 12.46528703574811558 ) ) ;
#4980=CARTESIAN_POINT ( 'NONE',  ( 2.908627838312458636, 45.87731371789854506, -15.53471296425188442 ) ) ;
#4982=CARTESIAN_POINT ( 'NONE',  ( 11.61527771782819940, 35.13518628210143646, -4.622313124798573369 ) ) ;
#4983=CARTESIAN_POINT ( 'NONE',  ( 4.944772684328679446, 70.78518628210144925, -11.48171059495397373 ) ) ;
#4984=CARTESIAN_POINT ( 'NONE',  ( 13.04141134922759804, 18.17268628210144499, 8.927990412390657937 ) ) ;
#4988=CARTESIAN_POINT ( 'NONE',  ( 15.50000000000000533, 26.51018628210144001, 0.1745138560725827404 ) ) ;
#4998=CARTESIAN_POINT ( 'NONE',  ( -3.796722387233185003, 109.4148137178985536, -8.710071997420207879 ) ) ;
#5004=CARTESIAN_POINT ( 'NONE',  ( 12.53471296425189330, 121.7773137178985792, 2.311890736173451533 ) ) ;
#5012=CARTESIAN_POINT ( 'NONE',  ( 8.715434833791931624, 36.86018628210144499, 8.962234695871760692 ) ) ;
#5021=CARTESIAN_POINT ( 'NONE',  ( 0.1745138560725515708, 61.01018628210145067, -12.50000000000000355 ) ) ;
#5027=CARTESIAN_POINT ( 'NONE',  ( 11.61527771782809637, 122.0648137178985735, 4.622313124798827388 ) ) ;
#5033=CARTESIAN_POINT ( 'NONE',  ( -13.23911966647199812, 90.15231371789855075, -8.632099005475788900 ) ) ;
#5037=CARTESIAN_POINT ( 'NONE',  ( 12.53471296425194836, 127.4226862821014663, -2.311890736173178418 ) ) ;
#5038=CARTESIAN_POINT ( 'NONE',  ( -15.46528703574804986, 68.19768628210142936, -3.257655550457287497 ) ) ;
#5041=CARTESIAN_POINT ( 'NONE',  ( 3.257655550457285720, 88.89768628210146062, -15.46528703574804986 ) ) ;
#5045=CARTESIAN_POINT ( 'NONE',  ( -9.500000000000005329, 12.71018628210143753, -0.1745138560725176813 ) ) ;
#5048=CARTESIAN_POINT ( 'NONE',  ( 10.49813415415989581, 64.17268628210143788, 7.228626920339068285 ) ) ;
#5051=CARTESIAN_POINT ( 'NONE',  ( -6.594114490232312775, 32.26018628210145067, -6.840914352312096547 ) ) ;
#5056=COLOUR_RGB ( '',0.8941176470588234615, 0.8941176470588234615, 0.8941176470588234615 ) ;
#5064=CARTESIAN_POINT ( 'NONE',  ( 12.50000000000000355, 81.71018628210144641, 0.1745138560725507937 ) ) ;
#5069=CARTESIAN_POINT ( 'NONE',  ( 6.092822981423662299, 49.61481371789856354, 14.25334919248795096 ) ) ;
#5075=CARTESIAN_POINT ( 'NONE',  ( -3.796722387233185003, 45.01481371789854791, -8.710071997420207879 ) ) ;
#5077=CARTESIAN_POINT ( 'NONE',  ( 5.233372021372610483, 101.6523137178985792, -8.152565276336593669 ) ) ;
#5080=CARTESIAN_POINT ( 'NONE',  ( 10.49813415416005213, 10.22731371789853227, -7.228626920338837358 ) ) ;
#5083=CARTESIAN_POINT ( 'NONE',  ( -2.311890736173176641, 69.92268628210146630, -12.53471296425194836 ) ) ;
#5090=CARTESIAN_POINT ( 'NONE',  ( 6.840914352312096547, 71.36018628210143788, -6.594114490232313663 ) ) ;
#5093=CARTESIAN_POINT ( 'NONE',  ( 12.53471296425194836, 118.2226862821014635, -2.311890736173178418 ) ) ;
#5105=CARTESIAN_POINT ( 'NONE',  ( -4.622313124798826500, 133.5648137178985735, 11.61527771782809637 ) ) ;
#5111=CARTESIAN_POINT ( 'NONE',  ( -8.962234695871565293, 7.639813717898541690, -8.715434833792128799 ) ) ;
#5113=CARTESIAN_POINT ( 'NONE',  ( 14.38691631536194393, 112.8648137178985564, 5.770363421894124656 ) ) ;
#5118=CARTESIAN_POINT ( 'NONE',  ( 8.962234695871762469, 117.3601862821014521, -8.715434833791931624 ) ) ;
#5124=CARTESIAN_POINT ( 'NONE',  ( 12.46528703574805874, 118.7976862821014663, 2.660918448318279950 ) ) ;
#5129=CARTESIAN_POINT ( 'NONE',  ( -11.08355503943142573, 112.7601862821014720, 10.83675517735155402 ) ) ;
#5131=CARTESIAN_POINT ( 'NONE',  ( -4.944772684328673229, 10.98518628210143433, 11.48171059495397728 ) ) ;
#5136=CARTESIAN_POINT ( 'NONE',  ( -3.796722387233375073, 75.38518628210142936, 8.710071997420127943 ) ) ;
#5143=CARTESIAN_POINT ( 'NONE',  ( 0.1745138560723095977, 50.18981371789855217, 9.500000000000005329 ) ) ;
#5147=CARTESIAN_POINT ( 'NONE',  ( 2.660918448318003282, 59.10231371789854649, 12.46528703574811558 ) ) ;
#5150=CARTESIAN_POINT ( 'NONE',  ( -7.228626920338836470, 26.32731371789854791, -10.49813415416005213 ) ) ;
#5167=CARTESIAN_POINT ( 'NONE',  ( 13.23911966647199812, 39.55231371789854933, 8.632099005475788900 ) ) ;
#5169=CARTESIAN_POINT ( 'NONE',  ( -11.48171059495397373, 4.085186282101443744, -4.944772684328680334 ) ) ;
#5170=CARTESIAN_POINT ( 'NONE',  ( 12.53471296425194836, 72.22268628210143504, -2.311890736173178418 ) ) ;
#5171=CARTESIAN_POINT ( 'NONE',  ( -10.83675517735155047, 13.86018628210145032, -11.08355503943142750 ) ) ;
#5176=CARTESIAN_POINT ( 'NONE',  ( -10.83675517735155047, 23.06018628210144783, -11.08355503943142750 ) ) ;
#5187=CARTESIAN_POINT ( 'NONE',  ( -8.710071997420207879, 107.1148137178985564, 3.796722387233182339 ) ) ;
#5193=CARTESIAN_POINT ( 'NONE',  ( 12.50000000000000355, 121.4898137178985564, -0.1745138560722771515 ) ) ;
#5206=CARTESIAN_POINT ( 'NONE',  ( 4.622313124798573369, 65.03518628210144925, 11.61527771782819940 ) ) ;
#5212=CARTESIAN_POINT ( 'NONE',  ( -8.962234695871565293, 127.2398137178985564, -8.715434833792128799 ) ) ;
#5219=CARTESIAN_POINT ( 'NONE',  ( -10.83675517735179028, 97.33981371789856496, 11.08355503943118947 ) ) ;
#5224=CARTESIAN_POINT ( 'NONE',  ( -6.932735513423968321, 124.5476862821014663, -10.69584247140445221 ) ) ;
#5225=CARTESIAN_POINT ( 'NONE',  ( -11.08355503943142573, 57.56018628210145494, 10.83675517735155402 ) ) ;
#5228=CARTESIAN_POINT ( 'NONE',  ( 2.908627838312118019, 83.72268628210143504, 15.53471296425195369 ) ) ;
#5233=CARTESIAN_POINT ( 'NONE',  ( 3.474262827703335166, 19.03518628210144570, 8.843639120294326972 ) ) ;
#5236=CARTESIAN_POINT ( 'NONE',  ( -4.944772684328673229, 56.98518628210144499, 11.48171059495397728 ) ) ;
#5239=CARTESIAN_POINT ( 'NONE',  ( -1.715153634034234598, 33.12268628210143362, -9.534712964251941258 ) ) ;
#5242=VERTEX_POINT ( 'NONE', #10496 ) ;
#5251=CARTESIAN_POINT ( 'NONE',  ( -7.228626920339070061, 84.87268628210145494, 10.49813415415989404 ) ) ;
#5256=CARTESIAN_POINT ( 'NONE',  ( 11.08355503943118769, 30.63981371789855146, 10.83675517735179028 ) ) ;
#5264=CARTESIAN_POINT ( 'NONE',  ( 2.064181346179061460, 31.50231371789854862, 9.465287035748106703 ) ) ;
#5266=CARTESIAN_POINT ( 'NONE',  ( 6.840914352311949109, 95.03981371789855359, 6.594114490232462877 ) ) ;
#5268=CARTESIAN_POINT ( 'NONE',  ( -5.770363421894122880, 142.7648137178985621, 14.38691631536194393 ) ) ;
#5269=CARTESIAN_POINT ( 'NONE',  ( 2.660918448318279950, 70.49768628210145494, -12.46528703574805697 ) ) ;
#5277=CARTESIAN_POINT ( 'NONE',  ( 6.840914352312096547, 80.56018628210146915, -6.594114490232313663 ) ) ;
#5279=CARTESIAN_POINT ( 'NONE',  ( -10.69584247140444866, 113.0476862821014663, 6.932735513423972762 ) ) ;
#5290=CARTESIAN_POINT ( 'NONE',  ( -10.69584247140429412, 117.7523137178986019, -6.932735513424201024 ) ) ;
#5291=CARTESIAN_POINT ( 'NONE',  ( 12.53471296425194659, 136.6226862821014834, -2.311890736173178418 ) ) ;
#5297=CARTESIAN_POINT ( 'NONE',  ( -15.53471296425188442, 107.9773137178985394, -2.908627838312459080 ) ) ;
#5305=CARTESIAN_POINT ( 'NONE',  ( -12.46528703574805697, 104.9976862821014691, -2.660918448318280838 ) ) ;
#5311=CARTESIAN_POINT ( 'NONE',  ( 10.69584247140445221, 117.6476862821014464, -6.932735513423970097 ) ) ;
#5317=CARTESIAN_POINT ( 'NONE',  ( 15.50000000000000533, 109.3101862821014549, 0.1745138560725827404 ) ) ;
#5318=CARTESIAN_POINT ( 'NONE',  ( 7.228626920339069173, 15.87268628210144961, -10.49813415415989404 ) ) ;
#5320=CARTESIAN_POINT ( 'NONE',  ( 9.500000000000005329, 136.9101862821014777, 0.1745138560725188748 ) ) ;
#5325=CARTESIAN_POINT ( 'NONE',  ( -5.529263428287477744, 66.47268628210146346, 7.954856959092191815 ) ) ;
#5331=CARTESIAN_POINT ( 'NONE',  ( 3.474262827703532341, 55.36481371789856354, -8.843639120294245259 ) ) ;
#5336=CARTESIAN_POINT ( 'NONE',  ( -12.50000000000000355, 61.68981371789855928, 0.1745138560722786503 ) ) ;
#5339=CARTESIAN_POINT ( 'NONE',  ( -12.53471296425189152, 34.37731371789855217, -2.311890736173453753 ) ) ;
#5343=CARTESIAN_POINT ( 'NONE',  ( -2.311890736173176641, 5.522686282101451738, -12.53471296425194836 ) ) ;
#5354=CARTESIAN_POINT ( 'NONE',  ( 15.53471296425188797, 20.57731371789854435, 2.908627838312457747 ) ) ;
#5356=CARTESIAN_POINT ( 'NONE',  ( 11.48171059495397728, 17.88518628210143646, 4.944772684328674117 ) ) ;
#5357=CARTESIAN_POINT ( 'NONE',  ( 12.46528703574805874, 45.19768628210143646, 2.660918448318279950 ) ) ;
#5361=CARTESIAN_POINT ( 'NONE',  ( 15.46528703574804986, 8.397686282101439303, 3.257655550457285720 ) ) ;
#5368=CARTESIAN_POINT ( 'NONE',  ( -0.1745138560723084320, 109.9898137178985706, -9.500000000000005329 ) ) ;
#5374=CARTESIAN_POINT ( 'NONE',  ( -8.715434833792127023, 124.9398137178985593, 8.962234695871568846 ) ) ;
#5386=CARTESIAN_POINT ( 'NONE',  ( -10.49813415415989581, 50.37268628210145494, -7.228626920339068285 ) ) ;
#5392=CARTESIAN_POINT ( 'NONE',  ( -7.228626920338836470, 99.92731371789855643, -10.49813415416005213 ) ) ;
#5397=CARTESIAN_POINT ( 'NONE',  ( -0.1745138560722442889, 91.58981371789856496, -15.50000000000000533 ) ) ;
#5401=CARTESIAN_POINT ( 'NONE',  ( 2.311890736173175753, 111.3226862821014720, 12.53471296425194836 ) ) ;
#5402=CARTESIAN_POINT ( 'NONE',  ( -5.770363421893818234, 69.63518628210144357, -14.38691631536207005 ) ) ;
#5406=CARTESIAN_POINT ( 'NONE',  ( -6.092822981423970496, 75.38518628210142936, 14.25334919248782661 ) ) ;
#5408=CARTESIAN_POINT ( 'NONE',  ( 8.152565276336714462, 25.64768628210144286, -5.233372021372432847 ) ) ;
#5412=CARTESIAN_POINT ( 'NONE',  ( 2.660918448318279950, 52.09768628210144215, -12.46528703574805697 ) ) ;
#5415=CARTESIAN_POINT ( 'NONE',  ( -8.152565276336710909, 30.24768628210144783, 5.233372021372435512 ) ) ;
#5427=CARTESIAN_POINT ( 'NONE',  ( -7.228626920339070061, 75.67268628210145209, 10.49813415415989404 ) ) ;
#5432=CARTESIAN_POINT ( 'NONE',  ( 13.04141134922778988, 37.82731371789854080, -8.927990412390371944 ) ) ;
#5439=CARTESIAN_POINT ( 'NONE',  ( 6.594114490232462877, 37.53981371789855359, -6.840914352311949109 ) ) ;
#5444=CARTESIAN_POINT ( 'NONE',  ( 12.53471296425189330, 20.57731371789854435, 2.311890736173451977 ) ) ;
#5447=CARTESIAN_POINT ( 'NONE',  ( 12.50000000000000355, 63.31018628210144072, 0.1745138560725507937 ) ) ;
#5455=CARTESIAN_POINT ( 'NONE',  ( -6.594114490232312775, 78.26018628210144357, -6.840914352312096547 ) ) ;
#5457=CARTESIAN_POINT ( 'NONE',  ( 2.311890736173175753, 120.5226862821014606, 12.53471296425194836 ) ) ;
#5470=CARTESIAN_POINT ( 'NONE',  ( -11.61527771782809282, 117.4648137178985650, -4.622313124798832717 ) ) ;
#5471=CARTESIAN_POINT ( 'NONE',  ( 4.944772684328679446, 125.9851862821014521, -11.48171059495397373 ) ) ;
#5477=CARTESIAN_POINT ( 'NONE',  ( -2.908627838312453306, 96.47731371789852517, 15.53471296425188797 ) ) ;
#5478=CARTESIAN_POINT ( 'NONE',  ( -0.1745138560725500443, 93.21018628210146062, 12.50000000000000355 ) ) ;
#5481=CARTESIAN_POINT ( 'NONE',  ( 10.69584247140445221, 117.6476862821014464, -6.932735513423970097 ) ) ;
#5486=CARTESIAN_POINT ( 'NONE',  ( -8.715434833791929847, 124.2601862821014578, -8.962234695871762469 ) ) ;
#5493=CARTESIAN_POINT ( 'NONE',  ( -5.770363421893818234, 97.23518628210146630, -14.38691631536207005 ) ) ;
#5494=CARTESIAN_POINT ( 'NONE',  ( 4.944772684328679446, 24.78518628210143859, -11.48171059495397373 ) ) ;
#5497=CARTESIAN_POINT ( 'NONE',  ( -1.715153634034234598, 125.1226862821014691, -9.534712964251941258 ) ) ;
#5502=CARTESIAN_POINT ( 'NONE',  ( 5.233372021372432847, 55.54768628210144499, 8.152565276336710909 ) ) ;
#5510=CARTESIAN_POINT ( 'NONE',  ( -5.233372021372612259, 41.85231371789854649, 8.152565276336593669 ) ) ;
#5514=CARTESIAN_POINT ( 'NONE',  ( 0.1745138560722779009, 68.58981371789856496, 12.50000000000000355 ) ) ;
#5517=CARTESIAN_POINT ( 'NONE',  ( -14.25334919248795096, 143.9148137178985678, 6.092822981423662299 ) ) ;
#5532=CARTESIAN_POINT ( 'NONE',  ( 11.08355503943118769, 12.23981371789853512, 10.83675517735179028 ) ) ;
#5534=CARTESIAN_POINT ( 'NONE',  ( -0.1745138560725500443, 10.41018628210144215, 12.50000000000000355 ) ) ;
#5537=CARTESIAN_POINT ( 'NONE',  ( 10.69584247140445221, 44.04768628210144499, -6.932735513423970097 ) ) ;
#5540=CARTESIAN_POINT ( 'NONE',  ( -14.25334919248782306, 13.28518628210143149, -6.092822981423979378 ) ) ;
#5550=CARTESIAN_POINT ( 'NONE',  ( 0.1745138560723095977, 96.18981371789855928, 9.500000000000005329 ) ) ;
#5557=CARTESIAN_POINT ( 'NONE',  ( 8.715434833792128799, 111.1398137178985621, -8.962234695871567070 ) ) ;
#5561=CARTESIAN_POINT ( 'NONE',  ( -12.53471296425189152, 80.37731371789854506, -2.311890736173453753 ) ) ;
#5570=CARTESIAN_POINT ( 'NONE',  ( 12.50000000000000355, 54.11018628210144499, 0.1745138560725507937 ) ) ;
#5576=CARTESIAN_POINT ( 'NONE',  ( -11.61527771782809282, 108.2648137178985621, -4.622313124798832717 ) ) ;
#5581=CARTESIAN_POINT ( 'NONE',  ( 13.04141134922778988, 83.82731371789856212, -8.927990412390371944 ) ) ;
#5585=CARTESIAN_POINT ( 'NONE',  ( -11.61527771782819940, 94.93518628210145494, 4.622313124798574258 ) ) ;
#5586=CARTESIAN_POINT ( 'NONE',  ( 13.04141134922759804, 64.17268628210143788, 8.927990412390657937 ) ) ;
#5589=CARTESIAN_POINT ( 'NONE',  ( -14.25334919248782306, 59.28518628210144925, -6.092822981423979378 ) ) ;
#5595=CARTESIAN_POINT ( 'NONE',  ( -7.228626920339069173, 38.87268628210144072, 10.49813415415989581 ) ) ;
#5598=CARTESIAN_POINT ( 'NONE',  ( -8.843639120294326972, 21.33518628210144641, 3.474262827703335166 ) ) ;
#5610=CARTESIAN_POINT ( 'NONE',  ( -4.622313124798576922, 60.43518628210145494, -11.61527771782819762 ) ) ;
#5617=CARTESIAN_POINT ( 'NONE',  ( -10.83675517735179028, 42.13981371789854791, 11.08355503943118947 ) ) ;
#5623=CARTESIAN_POINT ( 'NONE',  ( 2.064181346179061460, 13.10231371789855181, 9.465287035748106703 ) ) ;
#5630=CARTESIAN_POINT ( 'NONE',  ( -13.04141134922778456, 134.4273137178984996, 8.927990412390377273 ) ) ;
#5633=CARTESIAN_POINT ( 'NONE',  ( -12.46528703574805697, 58.99768628210144783, -2.660918448318280838 ) ) ;
#5641=CARTESIAN_POINT ( 'NONE',  ( 8.843639120294328748, 81.13518628210145778, -3.474262827703334722 ) ) ;
#5644=CARTESIAN_POINT ( 'NONE',  ( 8.962234695871762469, 89.76018628210144357, -8.715434833791931624 ) ) ;
#5657=CARTESIAN_POINT ( 'NONE',  ( 4.944772684328420986, 114.0148137178985621, 11.48171059495408208 ) ) ;
#5659=CARTESIAN_POINT ( 'NONE',  ( 12.53471296425194659, 127.4226862821014663, -2.311890736173178418 ) ) ;
#5665=CARTESIAN_POINT ( 'NONE',  ( -8.632099005475794229, 97.05231371789855643, 13.23911966647199812 ) ) ;
#5669=CARTESIAN_POINT ( 'NONE',  ( -0.1745138560723084320, 73.18981371789854506, -9.500000000000005329 ) ) ;
#5673=CARTESIAN_POINT ( 'NONE',  ( 10.69584247140429589, 57.95231371789854791, 6.932735513424201024 ) ) ;
#5675=CARTESIAN_POINT ( 'NONE',  ( -4.944772684328673229, 121.3851862821014578, 11.48171059495397728 ) ) ;
#5680=CARTESIAN_POINT ( 'NONE',  ( 15.53471296425195369, 99.82268628210142936, -2.908627838312120684 ) ) ;
#5681=CARTESIAN_POINT ( 'NONE',  ( -8.715434833791929847, 13.86018628210145032, -8.962234695871762469 ) ) ;
#5684=CARTESIAN_POINT ( 'NONE',  ( 7.954856959092191815, 137.7726862821014606, 5.529263428287477744 ) ) ;
#5689=CARTESIAN_POINT ( 'NONE',  ( -8.843639120294326972, 67.33518628210143220, 3.474262827703335166 ) ) ;
#5690=CARTESIAN_POINT ( 'NONE',  ( 10.69584247140445221, 16.44768628210144357, -6.932735513423970097 ) ) ;
#5698=CARTESIAN_POINT ( 'NONE',  ( 9.534712964251900402, 38.97731371789853938, 1.715153634034445540 ) ) ;
#5703=CARTESIAN_POINT ( 'NONE',  ( -2.311890736173447980, 41.27731371789855785, 12.53471296425189330 ) ) ;
#5706=CARTESIAN_POINT ( 'NONE',  ( 2.311890736173452865, 18.27731371789853299, -12.53471296425189152 ) ) ;
#5722=CARTESIAN_POINT ( 'NONE',  ( 5.770363421894130873, 27.76481371789854791, -14.38691631536193860 ) ) ;
#5724=CARTESIAN_POINT ( 'NONE',  ( 12.50000000000000355, 8.110186282101444988, 0.1745138560725507937 ) ) ;
#5725=CARTESIAN_POINT ( 'NONE',  ( -0.1745138560725500443, 47.21018628210143930, 12.50000000000000355 ) ) ;
#5738=CARTESIAN_POINT ( 'NONE',  ( -6.840914352311947333, 90.43981371789854506, -6.594114490232462877 ) ) ;
#5745=CARTESIAN_POINT ( 'NONE',  ( -12.50000000000000355, 98.48981371789855643, 0.1745138560722786503 ) ) ;
#5750=CARTESIAN_POINT ( 'NONE',  ( -4.622313124798826500, 69.16481371789855359, 11.61527771782809637 ) ) ;
#5760=CARTESIAN_POINT ( 'NONE',  ( -12.53471296425194836, 67.62268628210145494, 2.311890736173176641 ) ) ;
#5766=CARTESIAN_POINT ( 'NONE',  ( 10.49813415416005213, 111.4273137178985564, -7.228626920338837358 ) ) ;
#5772=CARTESIAN_POINT ( 'NONE',  ( 8.632099005475788900, 83.25231371789854506, -13.23911966647199812 ) ) ;
#5774=CIRCLE ( 'NONE', #3370, 1.499999999999990452 ) ;
#5777=CARTESIAN_POINT ( 'NONE',  ( 6.932735513423970097, 110.7476862821014549, 10.69584247140445044 ) ) ;
#5778=CARTESIAN_POINT ( 'NONE',  ( -8.632099005475501130, 50.94768628210145067, -13.23911966647218996 ) ) ;
#5782=CARTESIAN_POINT ( 'NONE',  ( 15.46528703574804986, 72.79768628210145209, 3.257655550457285720 ) ) ;
#5787=CARTESIAN_POINT ( 'NONE',  ( 8.715434833791931624, 46.06018628210144072, 8.962234695871760692 ) ) ;
#5790=CARTESIAN_POINT ( 'NONE',  ( 3.796722387233379514, 6.385186282101440902, -8.710071997420127943 ) ) ;
#5800=CARTESIAN_POINT ( 'NONE',  ( -10.49813415415989404, 59.57268628210145778, -7.228626920339069173 ) ) ;
#5808=CARTESIAN_POINT ( 'NONE',  ( -5.770363421894122880, 41.56481371789855217, 14.38691631536194393 ) ) ;
#5815=CARTESIAN_POINT ( 'NONE',  ( -1.715153634034442431, 22.87731371789854151, 9.534712964251900402 ) ) ;
#5821=CARTESIAN_POINT ( 'NONE',  ( 3.257655550456945548, 123.5023137178985451, 15.46528703574811736 ) ) ;
#5824=CARTESIAN_POINT ( 'NONE',  ( 10.69584247140445221, 44.04768628210144499, -6.932735513423970097 ) ) ;
#5833=CARTESIAN_POINT ( 'NONE',  ( 2.064181346179272847, 70.49768628210145494, -9.465287035748065847 ) ) ;
#5836=CARTESIAN_POINT ( 'NONE',  ( 12.46528703574805874, 91.19768628210145778, 2.660918448318279950 ) ) ;
#5848=CARTESIAN_POINT ( 'NONE',  ( -4.944772684328424539, 118.6148137178985564, -11.48171059495408031 ) ) ;
#5849=CARTESIAN_POINT ( 'NONE',  ( 2.311890736173175753, 129.7226862821014493, 12.53471296425194659 ) ) ;
#5855=CARTESIAN_POINT ( 'NONE',  ( -14.38691631536193860, 89.86481371789855643, -5.770363421894132649 ) ) ;
#5859=CARTESIAN_POINT ( 'NONE',  ( -5.529263428287297444, 81.52731371789856496, -7.954856959092311719 ) ) ;
#5862=CARTESIAN_POINT ( 'NONE',  ( 12.50000000000000355, 47.88981371789854791, -0.1745138560722771515 ) ) ;
#5864=CARTESIAN_POINT ( 'NONE',  ( 0.1745138560725515708, 107.0101862821014578, -12.50000000000000355 ) ) ;
#5869=CARTESIAN_POINT ( 'NONE',  ( -6.092822981423970496, 102.9851862821014805, 14.25334919248782661 ) ) ;
#5871=CARTESIAN_POINT ( 'NONE',  ( 12.53471296425194659, 7.822686282101448896, -2.311890736173178418 ) ) ;
#5874=CARTESIAN_POINT ( 'NONE',  ( -8.152565276336710909, 131.4476862821014436, 5.233372021372435512 ) ) ;
#5879=CARTESIAN_POINT ( 'NONE',  ( 9.465287035748067623, 63.59768628210142793, 2.064181346179272847 ) ) ;
#5887=CARTESIAN_POINT ( 'NONE',  ( 8.152565276336593669, 39.55231371789854933, 5.233372021372610483 ) ) ;
#5893=CARTESIAN_POINT ( 'NONE',  ( 12.46528703574811558, 47.60231371789855359, -2.660918448318005947 ) ) ;
#5896=CARTESIAN_POINT ( 'NONE',  ( 4.622313124798831829, 9.364813717898545775, -11.61527771782809282 ) ) ;
#5911=CARTESIAN_POINT ( 'NONE',  ( -10.83675517735179028, 23.73981371789854222, 11.08355503943118947 ) ) ;
#5913=CARTESIAN_POINT ( 'NONE',  ( -6.932735513423968321, 4.947686282101432909, -10.69584247140445221 ) ) ;
#5914=CARTESIAN_POINT ( 'NONE',  ( 12.50000000000000355, 54.11018628210144499, 0.1745138560725507937 ) ) ;
#5925=CARTESIAN_POINT ( 'NONE',  ( -6.594114490232462877, 97.33981371789856496, 6.840914352311949109 ) ) ;
#5933=CARTESIAN_POINT ( 'NONE',  ( 11.48171059495408208, 102.5148137178985621, -4.944772684328420986 ) ) ;
#5938=CARTESIAN_POINT ( 'NONE',  ( -12.50000000000000355, 61.68981371789855928, 0.1745138560722786503 ) ) ;
#5946=CARTESIAN_POINT ( 'NONE',  ( -12.50000000000000355, 40.31018628210144783, -0.1745138560725492671 ) ) ;
#5953=CARTESIAN_POINT ( 'NONE',  ( 4.944772684328420986, 95.61481371789857064, 11.48171059495408208 ) ) ;
#5959=CARTESIAN_POINT ( 'NONE',  ( -13.23911966647199812, 80.95231371789854791, -8.632099005475788900 ) ) ;
#5963=CARTESIAN_POINT ( 'NONE',  ( -12.50000000000000355, 104.7101862821014606, -0.1745138560725492671 ) ) ;
#5964=CARTESIAN_POINT ( 'NONE',  ( 5.770363421893814682, 37.43518628210144072, 14.38691631536207183 ) ) ;
#5967=CARTESIAN_POINT ( 'NONE',  ( -8.927990412390661490, 75.67268628210143788, 13.04141134922759804 ) ) ;
#5973=CARTESIAN_POINT ( 'NONE',  ( -10.49813415415989581, 31.97268628210143859, -7.228626920339068285 ) ) ;
#5976=CARTESIAN_POINT ( 'NONE',  ( -5.233372021372430183, 14.14768628210144286, -8.152565276336710909 ) ) ;
#5988=CARTESIAN_POINT ( 'NONE',  ( 11.61527771782819940, 62.73518628210145209, -4.622313124798573369 ) ) ;
#5995=CARTESIAN_POINT ( 'NONE',  ( -0.1745138560722442889, 36.38981371789855501, -15.50000000000000533 ) ) ;
#6002=CARTESIAN_POINT ( 'NONE',  ( -8.843639120294245259, 25.46481371789855075, -3.474262827703533230 ) ) ;
#6007=CARTESIAN_POINT ( 'NONE',  ( 14.25334919248795451, 130.1148137178985564, -6.092822981423661410 ) ) ;
#6009=CARTESIAN_POINT ( 'NONE',  ( 11.61527771782819940, 53.53518628210144925, -4.622313124798573369 ) ) ;
#6016=CARTESIAN_POINT ( 'NONE',  ( -9.534712964251941258, 58.42268628210145209, 1.715153634034234154 ) ) ;
#6019=CARTESIAN_POINT ( 'NONE',  ( 10.69584247140445221, 90.04768628210145209, -6.932735513423970097 ) ) ;
#6031=CARTESIAN_POINT ( 'NONE',  ( -12.46528703574811558, 125.8023137178985706, 2.660918448318003726 ) ) ;
#6032=CARTESIAN_POINT ( 'NONE',  ( 8.962234695871762469, 117.3601862821014521, -8.715434833791931624 ) ) ;
#6037=CARTESIAN_POINT ( 'NONE',  ( -10.83675517735179028, 88.13981371789856212, 11.08355503943118947 ) ) ;
#6042=CARTESIAN_POINT ( 'NONE',  ( -9.500000000000005329, 70.88981371789854791, 0.1745138560723101806 ) ) ;
#6045=CARTESIAN_POINT ( 'NONE',  ( 2.660918448318002838, 40.70231371789854791, 12.46528703574811558 ) ) ;
#6047=CARTESIAN_POINT ( 'NONE',  ( -10.69584247140444866, 94.64768628210146062, 6.932735513423972762 ) ) ;
#6052=CARTESIAN_POINT ( 'NONE',  ( -3.257655550457281723, 93.49768628210142651, 15.46528703574804986 ) ) ;
#6053=CARTESIAN_POINT ( 'NONE',  ( 6.932735513423970097, 18.74768628210144072, 10.69584247140445044 ) ) ;
#6056=CARTESIAN_POINT ( 'NONE',  ( 3.474262827703335166, 120.2351862821014521, 8.843639120294326972 ) ) ;
#6062=CARTESIAN_POINT ( 'NONE',  ( -8.152565276336710909, 67.04768628210143788, 5.233372021372435512 ) ) ;
#6069=CARTESIAN_POINT ( 'NONE',  ( 9.500000000000005329, 38.68981371789855217, -0.1745138560723090149 ) ) ;
#6075=CARTESIAN_POINT ( 'NONE',  ( -6.932735513424201912, 41.85231371789854649, 10.69584247140429412 ) ) ;
#6078=CARTESIAN_POINT ( 'NONE',  ( 10.49813415416005213, 19.42731371789854933, -7.228626920338837358 ) ) ;
#6095=CARTESIAN_POINT ( 'NONE',  ( 15.46528703574811736, 20.00231371789855217, -3.257655550456947768 ) ) ;
#6097=CARTESIAN_POINT ( 'NONE',  ( -6.594114490232312775, 133.4601862821014606, -6.840914352312096547 ) ) ;
#6098=CARTESIAN_POINT ( 'NONE',  ( 4.944772684328679446, 52.38518628210145067, -11.48171059495397373 ) ) ;
#6104=CARTESIAN_POINT ( 'NONE',  ( 9.534712964251941258, 17.02268628210144996, -1.715153634034235708 ) ) ;
#6112=CARTESIAN_POINT ( 'NONE',  ( -6.840914352311947333, 99.63981371789857633, -6.594114490232462877 ) ) ;
#6120=CARTESIAN_POINT ( 'NONE',  ( 12.53471296425189330, 94.17731371789855643, 2.311890736173451533 ) ) ;
#6124=CARTESIAN_POINT ( 'NONE',  ( 11.61527771782809637, 66.86481371789855643, 4.622313124798827388 ) ) ;
#6132=CARTESIAN_POINT ( 'NONE',  ( -10.49813415415989581, 31.97268628210143859, -7.228626920339068285 ) ) ;
#6139=CARTESIAN_POINT ( 'NONE',  ( -12.53471296425189152, 107.9773137178985536, -2.311890736173453753 ) ) ;
#6144=CARTESIAN_POINT ( 'NONE',  ( 5.770363421894130873, 73.76481371789856212, -14.38691631536193860 ) ) ;
#6150=CARTESIAN_POINT ( 'NONE',  ( 12.50000000000000355, 100.1101862821014521, 0.1745138560725507937 ) ) ;
#6151=CARTESIAN_POINT ( 'NONE',  ( 0.1745138560725837118, 51.81018628210144783, -15.50000000000000533 ) ) ;
#6155=CARTESIAN_POINT ( 'NONE',  ( 5.770363421893814682, 65.03518628210144925, 14.38691631536207183 ) ) ;
#6163=CARTESIAN_POINT ( 'NONE',  ( 0.1745138560725515708, 42.61018628210144499, -12.50000000000000355 ) ) ;
#6166=CARTESIAN_POINT ( 'NONE',  ( -9.500000000000005329, 12.71018628210143753, -0.1745138560725176813 ) ) ;
#6178=CARTESIAN_POINT ( 'NONE',  ( -10.69584247140444866, 76.24768628210144072, 6.932735513423972762 ) ) ;
#6185=CARTESIAN_POINT ( 'NONE',  ( -12.46528703574805697, 86.59768628210144925, -2.660918448318280838 ) ) ;
#6186=CARTESIAN_POINT ( 'NONE',  ( -15.50000000000000533, 24.88981371789854080, 0.1745138560722471477 ) ) ;
#6193=CARTESIAN_POINT ( 'NONE',  ( -5.529263428287297444, 17.12731371789855217, -7.954856959092311719 ) ) ;
#6198=CARTESIAN_POINT ( 'NONE',  ( -14.25334919248795096, 125.5148137178985763, 6.092822981423662299 ) ) ;
#6202=CARTESIAN_POINT ( 'NONE',  ( -11.48171059495397373, 50.08518628210144641, -4.944772684328680334 ) ) ;
#6210=CARTESIAN_POINT ( 'NONE',  ( -3.796722387233375073, 56.98518628210145209, 8.710071997420127943 ) ) ;
#6213=CARTESIAN_POINT ( 'NONE',  ( -8.715434833791929847, 96.66018628210146346, -8.962234695871762469 ) ) ;
#6225=CARTESIAN_POINT ( 'NONE',  ( -11.61527771782809282, 108.2648137178985621, -4.622313124798832717 ) ) ;
#6226=CARTESIAN_POINT ( 'NONE',  ( 4.622313124798573369, 129.4351862821014549, 11.61527771782819940 ) ) ;
#6231=CARTESIAN_POINT ( 'NONE',  ( 14.38691631536194393, 85.26481371789857633, 5.770363421894124656 ) ) ;
#6232=CIRCLE ( 'NONE', #2328, 1.499999999999990452 ) ;
#6235=CARTESIAN_POINT ( 'NONE',  ( 1.715153634034233487, 102.1226862821014549, 9.534712964251941258 ) ) ;
#6238=CARTESIAN_POINT ( 'NONE',  ( 8.843639120294245259, 66.86481371789854222, 3.474262827703527901 ) ) ;
#6242=CARTESIAN_POINT ( 'NONE',  ( 12.46528703574811558, 47.60231371789855359, -2.660918448318005503 ) ) ;
#6245=CARTESIAN_POINT ( 'NONE',  ( 6.932735513423970097, 101.5476862821014379, 10.69584247140445044 ) ) ;
#6249=CARTESIAN_POINT ( 'NONE',  ( 12.50000000000000355, 136.9101862821014777, 0.1745138560725507937 ) ) ;
#6251=CARTESIAN_POINT ( 'NONE',  ( 15.50000000000000533, 81.71018628210144641, 0.1745138560725827404 ) ) ;
#6256=CARTESIAN_POINT ( 'NONE',  ( 8.843639120294328748, 108.7351862821014663, -3.474262827703334722 ) ) ;
#6258=CARTESIAN_POINT ( 'NONE',  ( -13.04141134922759804, 13.57268628210145422, -8.927990412390657937 ) ) ;
#6269=CARTESIAN_POINT ( 'NONE',  ( -8.843639120294245259, 43.86481371789854933, -3.474262827703533230 ) ) ;
#6273=CARTESIAN_POINT ( 'NONE',  ( -10.69584247140429412, 44.15231371789854364, -6.932735513424201024 ) ) ;
#6275=CARTESIAN_POINT ( 'NONE',  ( -0.1745138560722763466, 8.789813717898553591, -12.50000000000000355 ) ) ;
#6291=CARTESIAN_POINT ( 'NONE',  ( 14.25334919248782661, 137.4851862821014379, 6.092822981423971385 ) ) ;
#6295=CARTESIAN_POINT ( 'NONE',  ( -8.843639120294326972, 122.5351862821014493, 3.474262827703335166 ) ) ;
#6297=CARTESIAN_POINT ( 'NONE',  ( -2.311890736173176641, 33.12268628210144072, -12.53471296425194836 ) ) ;
#6303=CARTESIAN_POINT ( 'NONE',  ( 15.50000000000000533, 127.7101862821014606, 0.1745138560725827404 ) ) ;
#6305=CARTESIAN_POINT ( 'NONE',  ( -3.474262827703337830, 23.63518628210144357, -8.843639120294326972 ) ) ;
#6311=CARTESIAN_POINT ( 'NONE',  ( 7.954856959092311719, 102.2273137178985678, -5.529263428287300108 ) ) ;
#6316=CARTESIAN_POINT ( 'NONE',  ( 6.932735513424201024, 92.45231371789854791, -10.69584247140429412 ) ) ;
#6320=CARTESIAN_POINT ( 'NONE',  ( -11.48171059495408208, 61.11481371789854933, 4.944772684328421875 ) ) ;
#6329=CARTESIAN_POINT ( 'NONE',  ( 4.622313124798573369, 37.43518628210144783, 11.61527771782819940 ) ) ;
#6334=CARTESIAN_POINT ( 'NONE',  ( -8.715434833792127023, 88.13981371789856212, 8.962234695871568846 ) ) ;
#6340=CARTESIAN_POINT ( 'NONE',  ( -10.83675517735179028, 69.73981371789855643, 11.08355503943118947 ) ) ;
#6344=CARTESIAN_POINT ( 'NONE',  ( -8.715434833791929847, 87.46018628210144641, -8.962234695871762469 ) ) ;
#6345=CARTESIAN_POINT ( 'NONE',  ( 14.25334919248782661, 45.48518628210144499, 6.092822981423971385 ) ) ;
#6349=CARTESIAN_POINT ( 'NONE',  ( -5.770363421893818234, 51.23518628210143788, -14.38691631536207005 ) ) ;
#6355=CARTESIAN_POINT ( 'NONE',  ( 0.1745138560725515708, 33.41018628210144925, -12.50000000000000355 ) ) ;
#6357=CARTESIAN_POINT ( 'NONE',  ( -9.465287035748065847, 3.797686282101448096, -2.064181346179273735 ) ) ;
#6367=CARTESIAN_POINT ( 'NONE',  ( -11.48171059495397373, 50.08518628210144641, -4.944772684328680334 ) ) ;
#6373=CARTESIAN_POINT ( 'NONE',  ( -8.715434833791929847, 96.66018628210146346, -8.962234695871762469 ) ) ;
#6374=CARTESIAN_POINT ( 'NONE',  ( 15.50000000000000533, 20.28981371789855004, -0.1745138560722452326 ) ) ;
#6380=CARTESIAN_POINT ( 'NONE',  ( 8.152565276336593669, 11.95231371789853902, 5.233372021372610483 ) ) ;
#6387=CARTESIAN_POINT ( 'NONE',  ( -13.23911966647199812, 136.1523137178985507, -8.632099005475788900 ) ) ;
#6392=CARTESIAN_POINT ( 'NONE',  ( -8.715434833791929847, 41.46018628210144641, -8.962234695871762469 ) ) ;
#6399=CARTESIAN_POINT ( 'NONE',  ( 9.500000000000005329, 54.11018628210144499, 0.1745138560725188748 ) ) ;
#6402=CARTESIAN_POINT ( 'NONE',  ( 2.660918448318279950, 88.89768628210146062, -12.46528703574805697 ) ) ;
#6416=CARTESIAN_POINT ( 'NONE',  ( -6.932735513424201912, 97.05231371789857064, 10.69584247140429412 ) ) ;
#6417=CARTESIAN_POINT ( 'NONE',  ( -8.715434833791929847, 96.66018628210146346, -8.962234695871762469 ) ) ;
#6422=CARTESIAN_POINT ( 'NONE',  ( -14.38691631536193860, 71.46481371789856496, -5.770363421894132649 ) ) ;
#6425=CARTESIAN_POINT ( 'NONE',  ( -9.465287035748065847, 95.79768628210145209, -2.064181346179273735 ) ) ;
#6428=CARTESIAN_POINT ( 'NONE',  ( 9.500000000000005329, 84.68981371789855928, -0.1745138560723090149 ) ) ;
#6431=CARTESIAN_POINT ( 'NONE',  ( -10.69584247140429412, 53.35231371789855359, -6.932735513424201024 ) ) ;
#6433=CARTESIAN_POINT ( 'NONE',  ( -2.660918448318275509, 102.6976862821014720, 12.46528703574805874 ) ) ;
#6437=CARTESIAN_POINT ( 'NONE',  ( 10.49813415415989581, 137.7726862821014606, 7.228626920339068285 ) ) ;
#6439=CARTESIAN_POINT ( 'NONE',  ( 2.908627838312118019, 74.52268628210144641, 15.53471296425195369 ) ) ;
#6441=CARTESIAN_POINT ( 'NONE',  ( -2.311890736173176641, 5.522686282101451738, -12.53471296425194659 ) ) ;
#6444=CARTESIAN_POINT ( 'NONE',  ( -1.715153634034234598, 115.9226862821014521, -9.534712964251941258 ) ) ;
#6446=CARTESIAN_POINT ( 'NONE',  ( 8.927990412390657937, 6.672686282101436106, -13.04141134922759804 ) ) ;
#6461=CARTESIAN_POINT ( 'NONE',  ( 8.843639120294245259, 20.86481371789854578, 3.474262827703527901 ) ) ;
#6465=CARTESIAN_POINT ( 'NONE',  ( -10.49813415416004858, 42.42731371789855643, 7.228626920338840023 ) ) ;
#6468=CARTESIAN_POINT ( 'NONE',  ( -10.83675517735179028, 134.1398137178985621, 11.08355503943118947 ) ) ;
#6485=CARTESIAN_POINT ( 'NONE',  ( 13.23911966647218996, 136.0476862821014379, -8.632099005475504683 ) ) ;
#6487=CARTESIAN_POINT ( 'NONE',  ( 0.1745138560725194299, 134.6101862821014947, -9.500000000000005329 ) ) ;
#6489=CARTESIAN_POINT ( 'NONE',  ( -6.932735513423968321, 23.34768628210144570, -10.69584247140445221 ) ) ;
#6493=CARTESIAN_POINT ( 'NONE',  ( 2.908627838312118019, 129.7226862821014208, 15.53471296425195369 ) ) ;
#6495=CARTESIAN_POINT ( 'NONE',  ( 6.594114490232313663, 9.260186282101427580, 6.840914352312096547 ) ) ;
#6501=CARTESIAN_POINT ( 'NONE',  ( -6.594114490232462877, 78.93981371789855928, 6.840914352311949109 ) ) ;
#6505=CARTESIAN_POINT ( 'NONE',  ( -12.53471296425189152, 107.9773137178985678, -2.311890736173453309 ) ) ;
#6509=CARTESIAN_POINT ( 'NONE',  ( 2.660918448318002838, 59.10231371789854649, 12.46528703574811558 ) ) ;
#6517=CARTESIAN_POINT ( 'NONE',  ( -2.311890736173176641, 33.12268628210144072, -12.53471296425194836 ) ) ;
#6524=CARTESIAN_POINT ( 'NONE',  ( 2.660918448318002838, 86.70231371789854791, 12.46528703574811558 ) ) ;
#6529=CARTESIAN_POINT ( 'NONE',  ( 15.53471296425188797, 57.37731371789855928, 2.908627838312457747 ) ) ;
#6532=CARTESIAN_POINT ( 'NONE',  ( 4.622313124798573369, 83.43518628210145494, 11.61527771782819940 ) ) ;
#6533=CARTESIAN_POINT ( 'NONE',  ( -2.908627838312119351, 33.12268628210143362, -15.53471296425195369 ) ) ;
#6537=CARTESIAN_POINT ( 'NONE',  ( 8.632099005475504683, 46.34768628210144925, 13.23911966647218996 ) ) ;
#6543=CARTESIAN_POINT ( 'NONE',  ( 4.944772684328679446, 15.58518628210145351, -11.48171059495397373 ) ) ;
#6545=CARTESIAN_POINT ( 'NONE',  ( 0.1745138560723095977, 123.7898137178985678, 9.500000000000005329 ) ) ;
#6555=CARTESIAN_POINT ( 'NONE',  ( 8.962234695871762469, 52.96018628210144641, -8.715434833791931624 ) ) ;
#6562=CARTESIAN_POINT ( 'NONE',  ( 8.962234695871762469, 89.76018628210144357, -8.715434833791931624 ) ) ;
#6563=CARTESIAN_POINT ( 'NONE',  ( -14.38691631536193860, 25.46481371789855075, -5.770363421894132649 ) ) ;
#6570=CARTESIAN_POINT ( 'NONE',  ( 7.228626920338837358, 141.3273137178985337, 10.49813415416005036 ) ) ;
#6575=CARTESIAN_POINT ( 'NONE',  ( 5.770363421894130873, 119.7648137178985905, -14.38691631536193860 ) ) ;
#6578=CARTESIAN_POINT ( 'NONE',  ( 4.622313124798573369, 28.23518628210144854, 11.61527771782819940 ) ) ;
#6580=EDGE_CURVE ( 'NONE', #21580, #5242, #5774, .T. ) ;
#6583=CARTESIAN_POINT ( 'NONE',  ( -6.092822981423970496, 112.1851862821014691, 14.25334919248782661 ) ) ;
#6586=CARTESIAN_POINT ( 'NONE',  ( 2.064181346179272847, 61.29768628210142367, -9.465287035748065847 ) ) ;
#6590=CARTESIAN_POINT ( 'NONE',  ( -11.61527771782819940, 76.53518628210146346, 4.622313124798574258 ) ) ;
#6603=CARTESIAN_POINT ( 'NONE',  ( 12.53471296425189330, 103.3773137178985735, 2.311890736173451977 ) ) ;
#6604=CARTESIAN_POINT ( 'NONE',  ( 12.50000000000000355, 100.1101862821014521, 0.1745138560725507937 ) ) ;
#6609=CARTESIAN_POINT ( 'NONE',  ( -13.23911966647199812, 80.95231371789854791, -8.632099005475788900 ) ) ;
#6612=CARTESIAN_POINT ( 'NONE',  ( -2.064181346179269738, 102.6976862821014294, 9.465287035748067623 ) ) ;
#6614=CARTESIAN_POINT ( 'NONE',  ( 7.954856959092311719, 56.22731371789854649, -5.529263428287300108 ) ) ;
#6617=CARTESIAN_POINT ( 'NONE',  ( 2.064181346179061460, 105.1023137178985678, 9.465287035748106703 ) ) ;
#6619=CARTESIAN_POINT ( 'NONE',  ( -0.1745138560722763466, 45.58981371789855075, -12.50000000000000355 ) ) ;
#6621=CARTESIAN_POINT ( 'NONE',  ( -2.311890736173176641, 97.52268628210144641, -12.53471296425194836 ) ) ;
#6624=CARTESIAN_POINT ( 'NONE',  ( -12.46528703574805697, 132.5976862821014777, -2.660918448318280838 ) ) ;
#6626=CARTESIAN_POINT ( 'NONE',  ( 13.04141134922759804, 91.77268628210144641, 8.927990412390657937 ) ) ;
#6631=CARTESIAN_POINT ( 'NONE',  ( -5.529263428287477744, 112.4726862821014635, 7.954856959092191815 ) ) ;
#6634=CARTESIAN_POINT ( 'NONE',  ( -13.04141134922759804, 4.372686282101438948, -8.927990412390657937 ) ) ;
#6645=CARTESIAN_POINT ( 'NONE',  ( 3.474262827703532341, 27.76481371789854791, -8.843639120294245259 ) ) ;
#6650=CARTESIAN_POINT ( 'NONE',  ( 4.622313124798831829, 18.56481371789855928, -11.61527771782809282 ) ) ;
#6652=CARTESIAN_POINT ( 'NONE',  ( 11.08355503943118769, 131.8398137178985792, 10.83675517735179028 ) ) ;
#6670=CARTESIAN_POINT ( 'NONE',  ( 5.770363421893814682, 138.6351862821014720, 14.38691631536207183 ) ) ;
#6673=CARTESIAN_POINT ( 'NONE',  ( 9.500000000000005329, 136.9101862821014777, 0.1745138560725188748 ) ) ;
#6676=CARTESIAN_POINT ( 'NONE',  ( -10.49813415415989581, 22.77268628210143575, -7.228626920339068285 ) ) ;
#6681=CARTESIAN_POINT ( 'NONE',  ( -2.908627838312119351, 125.1226862821014691, -15.53471296425195369 ) ) ;
#6683=CARTESIAN_POINT ( 'NONE',  ( -6.840914352312096547, 11.56018628210145316, 6.594114490232313663 ) ) ;
#6690=CARTESIAN_POINT ( 'NONE',  ( 9.534712964251900402, 66.57731371789853370, 1.715153634034445540 ) ) ;
#6694=CARTESIAN_POINT ( 'NONE',  ( -12.46528703574811558, 89.00231371789855928, 2.660918448318004170 ) ) ;
#6698=CARTESIAN_POINT ( 'NONE',  ( 8.715434833792128799, 46.73981371789854933, -8.962234695871567070 ) ) ;
#6704=CARTESIAN_POINT ( 'NONE',  ( 4.622313124798573369, 28.23518628210144854, 11.61527771782819940 ) ) ;
#6710=CARTESIAN_POINT ( 'NONE',  ( -10.69584247140429412, 90.15231371789856496, -6.932735513424201024 ) ) ;
#6716=CARTESIAN_POINT ( 'NONE',  ( -14.38691631536193860, 53.06481371789855928, -5.770363421894132649 ) ) ;
#6719=CARTESIAN_POINT ( 'NONE',  ( -10.49813415415989581, 87.17268628210143788, -7.228626920339068285 ) ) ;
#6721=CARTESIAN_POINT ( 'NONE',  ( 0.1745138560725837118, 33.41018628210144925, -15.50000000000000533 ) ) ;
#6725=CARTESIAN_POINT ( 'NONE',  ( 13.23911966647218996, 53.24768628210144783, -8.632099005475504683 ) ) ;
#6731=CARTESIAN_POINT ( 'NONE',  ( -12.50000000000000355, 12.71018628210143753, -0.1745138560725492671 ) ) ;
#6733=CARTESIAN_POINT ( 'NONE',  ( 9.465287035748106703, 130.4023137178985792, -2.064181346179063237 ) ) ;
#6742=CARTESIAN_POINT ( 'NONE',  ( 12.46528703574805874, 45.19768628210144357, 2.660918448318279950 ) ) ;
#6750=CARTESIAN_POINT ( 'NONE',  ( -4.622313124798576922, 88.03518628210144925, -11.61527771782819762 ) ) ;
#6751=CARTESIAN_POINT ( 'NONE',  ( -0.1745138560722442889, 27.18981371789855572, -15.50000000000000533 ) ) ;
#6757=CARTESIAN_POINT ( 'NONE',  ( 2.660918448318002838, 141.9023137178985792, 12.46528703574811558 ) ) ;
#6762=CARTESIAN_POINT ( 'NONE',  ( -11.08355503943118592, 118.0398137178985536, -10.83675517735179383 ) ) ;
#6765=CARTESIAN_POINT ( 'NONE',  ( -12.46528703574805697, 31.39768628210144641, -2.660918448318280838 ) ) ;
#6769=CARTESIAN_POINT ( 'NONE',  ( -2.908627838312119351, 97.52268628210144641, -15.53471296425195369 ) ) ;
#6772=CARTESIAN_POINT ( 'NONE',  ( 5.233372021372432847, 55.54768628210144499, 8.152565276336710909 ) ) ;
#6776=CARTESIAN_POINT ( 'NONE',  ( -11.48171059495397373, 77.68518628210145494, -4.944772684328680334 ) ) ;
#6779=CARTESIAN_POINT ( 'NONE',  ( 7.954856959092191815, 45.77268628210144641, 5.529263428287477744 ) ) ;
#6789=CARTESIAN_POINT ( 'NONE',  ( 11.48171059495408208, 111.7148137178985650, -4.944772684328420986 ) ) ;
#6790=CARTESIAN_POINT ( 'NONE',  ( -0.1745138560725500443, 102.4101862821014493, 12.50000000000000355 ) ) ;
#6795=CARTESIAN_POINT ( 'NONE',  ( 6.092822981423662299, 77.21481371789855075, 14.25334919248795096 ) ) ;
#6799=CARTESIAN_POINT ( 'NONE',  ( -9.534712964251941258, 104.4226862821014521, 1.715153634034234154 ) ) ;
#6801=CARTESIAN_POINT ( 'NONE',  ( -6.840914352311947333, 53.63981371789855501, -6.594114490232462877 ) ) ;
#6803=CARTESIAN_POINT ( 'NONE',  ( 5.233372021372610483, 120.0523137178985280, -8.152565276336593669 ) ) ;
#6805=CARTESIAN_POINT ( 'NONE',  ( -11.61527771782809282, 25.46481371789855075, -4.622313124798832717 ) ) ;
#6807=CARTESIAN_POINT ( 'NONE',  ( 10.69584247140445221, 80.84768628210144925, -6.932735513423970097 ) ) ;
#6812=CARTESIAN_POINT ( 'NONE',  ( -11.08355503943142573, 85.16018628210146346, 10.83675517735155402 ) ) ;
#6816=CARTESIAN_POINT ( 'NONE',  ( 6.840914352312096547, 117.3601862821014663, -6.594114490232313663 ) ) ;
#6819=CARTESIAN_POINT ( 'NONE',  ( -11.61527771782819940, 131.7351862821014663, 4.622313124798574258 ) ) ;
#6831=CARTESIAN_POINT ( 'NONE',  ( -2.064181346179062349, 17.70231371789854435, -9.465287035748106703 ) ) ;
#6836=CARTESIAN_POINT ( 'NONE',  ( -2.660918448318005058, 17.70231371789854435, -12.46528703574811558 ) ) ;
#6838=CARTESIAN_POINT ( 'NONE',  ( -8.632099005475794229, 124.6523137178985650, 13.23911966647199812 ) ) ;
#6848=CARTESIAN_POINT ( 'NONE',  ( 10.49813415415989581, 128.5726862821014720, 7.228626920339068285 ) ) ;
#6853=( LENGTH_UNIT ( ) NAMED_UNIT ( * ) SI_UNIT ( .MILLI., .METRE. ) );
#6862=CARTESIAN_POINT ( 'NONE',  ( -0.1745138560725817967, 130.0101862821014436, 15.50000000000000533 ) ) ;
#6865=CARTESIAN_POINT ( 'NONE',  ( 1.715153634034233487, 120.5226862821014322, 9.534712964251941258 ) ) ;
#6867=CARTESIAN_POINT ( 'NONE',  ( -10.69584247140444866, 39.44768628210145067, 6.932735513423972762 ) ) ;
#6871=CARTESIAN_POINT ( 'NONE',  ( 6.092822981423978490, 116.7851862821014635, -14.25334919248782306 ) ) ;
#6874=CARTESIAN_POINT ( 'NONE',  ( -3.796722387233185003, 137.0148137178985621, -8.710071997420207879 ) ) ;
#6881=CARTESIAN_POINT ( 'NONE',  ( -9.465287035748106703, 79.80231371789852801, 2.064181346179061460 ) ) ;
#6885=CARTESIAN_POINT ( 'NONE',  ( -10.49813415416004858, 88.42731371789858485, 7.228626920338840023 ) ) ;
#6887=CARTESIAN_POINT ( 'NONE',  ( -7.856644100452656154, 143.0000000000000568, 10.55002382876331524 ) ) ;
#6889=CARTESIAN_POINT ( 'NONE',  ( -11.61527771782809282, 43.86481371789854933, -4.622313124798832717 ) ) ;
#6895=CARTESIAN_POINT ( 'NONE',  ( 11.61527771782819940, 16.73518628210143788, -4.622313124798573369 ) ) ;
#6904=CARTESIAN_POINT ( 'NONE',  ( 2.311890736173452865, 82.67731371789855643, -12.53471296425189152 ) ) ;
#6910=CARTESIAN_POINT ( 'NONE',  ( -15.46528703574811736, 52.20231371789854080, 3.257655550456946436 ) ) ;
#6914=CARTESIAN_POINT ( 'NONE',  ( -8.962234695871760692, 94.36018628210145209, 8.715434833791933400 ) ) ;
#6915=CARTESIAN_POINT ( 'NONE',  ( -3.257655550457281723, 29.09768628210144925, 15.46528703574804986 ) ) ;
#6919=CARTESIAN_POINT ( 'NONE',  ( 0.1745138560725837118, 42.61018628210144499, -15.50000000000000533 ) ) ;
#6925=CARTESIAN_POINT ( 'NONE',  ( 12.46528703574805874, 26.79768628210144144, 2.660918448318279950 ) ) ;
#6927=CARTESIAN_POINT ( 'NONE',  ( -0.1745138560723084320, 137.5898137178985792, -9.500000000000005329 ) ) ;
#6932=CARTESIAN_POINT ( 'NONE',  ( -11.08355503943142573, 94.36018628210146630, 10.83675517735155402 ) ) ;
#6934=CARTESIAN_POINT ( 'NONE',  ( 12.53471296425189330, 130.9773137178985678, 2.311890736173451533 ) ) ;
#6942=CARTESIAN_POINT ( 'NONE',  ( 10.69584247140445221, 53.24768628210144072, -6.932735513423970097 ) ) ;
#6950=CARTESIAN_POINT ( 'NONE',  ( 7.228626920339068285, 80.27268628210146062, -10.49813415415989581 ) ) ;
#6951=CARTESIAN_POINT ( 'NONE',  ( -15.50000000000000533, 15.68981371789854329, 0.1745138560722471477 ) ) ;
#6959=CARTESIAN_POINT ( 'NONE',  ( 10.69584247140429589, 140.7523137178985735, 6.932735513424201024 ) ) ;
#6965=CARTESIAN_POINT ( 'NONE',  ( 14.25334919248795451, 111.7148137178985792, -6.092822981423661410 ) ) ;
#6968=CARTESIAN_POINT ( 'NONE',  ( 11.48171059495397728, 36.28518628210144925, 4.944772684328674117 ) ) ;
#6972=CARTESIAN_POINT ( 'NONE',  ( 13.23911966647218996, 108.4476862821014294, -8.632099005475504683 ) ) ;
#6975=CARTESIAN_POINT ( 'NONE',  ( -3.796722387233375073, 47.78518628210144215, 8.710071997420127943 ) ) ;
#6980=CARTESIAN_POINT ( 'NONE',  ( -4.944772684328673229, 84.58518628210146062, 11.48171059495397728 ) ) ;
#6983=CARTESIAN_POINT ( 'NONE',  ( 9.500000000000005329, 44.91018628210144215, 0.1745138560725188748 ) ) ;
#6993=CARTESIAN_POINT ( 'NONE',  ( 10.69584247140429589, 94.75231371789854506, 6.932735513424201024 ) ) ;
#6994=CARTESIAN_POINT ( 'NONE',  ( 11.61527771782819940, 99.53518628210144925, -4.622313124798573369 ) ) ;
#6999=CARTESIAN_POINT ( 'NONE',  ( 3.257655550456945548, 68.30231371789852801, 15.46528703574811736 ) ) ;
#7003=CARTESIAN_POINT ( 'NONE',  ( 8.843639120294328748, 108.7351862821014663, -3.474262827703334722 ) ) ;
#7005=CARTESIAN_POINT ( 'NONE',  ( 2.064181346179061460, 59.10231371789854649, 9.465287035748106703 ) ) ;
#7008=CARTESIAN_POINT ( 'NONE',  ( 9.534712964251900402, 112.5773137178985479, 1.715153634034445540 ) ) ;
#7010=CARTESIAN_POINT ( 'NONE',  ( 10.69584247140429589, 21.15231371789855430, 6.932735513424201024 ) ) ;
#7011=CARTESIAN_POINT ( 'NONE',  ( -4.622313124798576922, 88.03518628210144925, -11.61527771782819762 ) ) ;
#7020=CARTESIAN_POINT ( 'NONE',  ( -6.840914352312096547, 103.5601862821014407, 6.594114490232313663 ) ) ;
#7022=VECTOR ( 'NONE', #9594, 1000.000000000000000 ) ;
#7023=CARTESIAN_POINT ( 'NONE',  ( -12.46528703574805697, 123.3976862821014606, -2.660918448318280838 ) ) ;
#7036=CARTESIAN_POINT ( 'NONE',  ( -3.474262827703527901, 13.96481371789853831, 8.843639120294245259 ) ) ;
#7039=ORIENTED_EDGE ( 'NONE', *, *, #9923, .F. ) ;
#7041=CARTESIAN_POINT ( 'NONE',  ( -7.228626920338836470, 17.12731371789855217, -10.49813415416005213 ) ) ;
#7043=CARTESIAN_POINT ( 'NONE',  ( 13.04141134922778988, 129.8273137178985905, -8.927990412390371944 ) ) ;
#7050=CARTESIAN_POINT ( 'NONE',  ( -0.1745138560725500443, 139.2101862821014606, 12.50000000000000355 ) ) ;
#7060=CARTESIAN_POINT ( 'NONE',  ( -0.1745138560725817967, 139.2101862821014890, 15.50000000000000533 ) ) ;
#7063=CARTESIAN_POINT ( 'NONE',  ( -9.465287035748065847, 114.1976862821014578, -2.064181346179273735 ) ) ;
#7065=CARTESIAN_POINT ( 'NONE',  ( 6.932735513423970097, 37.14768628210143930, 10.69584247140445044 ) ) ;
#7071=CARTESIAN_POINT ( 'NONE',  ( -13.04141134922759804, 114.7726862821014322, -8.927990412390657937 ) ) ;
#7073=CARTESIAN_POINT ( 'NONE',  ( 9.465287035748067623, 8.397686282101439303, 2.064181346179272847 ) ) ;
#7080=CARTESIAN_POINT ( 'NONE',  ( -3.796722387233185003, 72.61481371789855643, -8.710071997420207879 ) ) ;
#7083=CARTESIAN_POINT ( 'NONE',  ( 4.622313124798831829, 82.96481371789856496, -11.61527771782809282 ) ) ;
#7085=CARTESIAN_POINT ( 'NONE',  ( -6.422845572874366304, 142.9999999999996305, 10.72508787064079172 ) ) ;
#7087=CARTESIAN_POINT ( 'NONE',  ( 2.660918448318002838, 49.90231371789855075, 12.46528703574811558 ) ) ;
#7092=CARTESIAN_POINT ( 'NONE',  ( -12.50000000000000355, 12.71018628210143753, -0.1745138560725492671 ) ) ;
#7097=CARTESIAN_POINT ( 'NONE',  ( 2.311890736173452865, 91.87731371789855928, -12.53471296425189152 ) ) ;
#7102=CARTESIAN_POINT ( 'NONE',  ( 8.927990412390371944, 49.32731371789854791, 13.04141134922778811 ) ) ;
#7105=CARTESIAN_POINT ( 'NONE',  ( 7.228626920339068285, 80.27268628210146062, -10.49813415415989581 ) ) ;
#7106=CARTESIAN_POINT ( 'NONE',  ( -10.83675517735155047, 23.06018628210144783, -11.08355503943142750 ) ) ;
#7109=CARTESIAN_POINT ( 'NONE',  ( -15.46528703574804986, 40.59768628210144215, -3.257655550457287497 ) ) ;
#7116=CARTESIAN_POINT ( 'NONE',  ( -2.311890736173176641, 23.92268628210143788, -12.53471296425194836 ) ) ;
#7118=CARTESIAN_POINT ( 'NONE',  ( 5.529263428287300108, 132.1273137178985735, 7.954856959092309943 ) ) ;
#7122=CARTESIAN_POINT ( 'NONE',  ( 2.311890736173452421, 128.6773137178985564, -12.53471296425189152 ) ) ;
#7128=CARTESIAN_POINT ( 'NONE',  ( 8.715434833791931624, 55.26018628210144357, 8.962234695871760692 ) ) ;
#7137=CARTESIAN_POINT ( 'NONE',  ( -8.715434833791929847, 69.06018628210145494, -8.962234695871762469 ) ) ;
#7138=CARTESIAN_POINT ( 'NONE',  ( 15.46528703574804986, 137.1976862821014436, 3.257655550457285720 ) ) ;
#7143=CARTESIAN_POINT ( 'NONE',  ( -6.932735513424201912, 133.8523137178985678, 10.69584247140429412 ) ) ;
#7150=CARTESIAN_POINT ( 'NONE',  ( 13.23911966647199812, 113.1523137178985650, 8.632099005475788900 ) ) ;
#7156=CARTESIAN_POINT ( 'NONE',  ( 11.08355503943142750, 98.96018628210144641, -10.83675517735155225 ) ) ;
#7160=CARTESIAN_POINT ( 'NONE',  ( -0.1745138560725182642, 47.21018628210144641, 9.500000000000005329 ) ) ;
#7165=CARTESIAN_POINT ( 'NONE',  ( -0.1745138560725500443, 84.01018628210145778, 12.50000000000000355 ) ) ;
#7168=CARTESIAN_POINT ( 'NONE',  ( 3.796722387233379514, 43.18518628210144072, -8.710071997420127943 ) ) ;
#7178=CARTESIAN_POINT ( 'NONE',  ( 8.715434833792128799, 92.73981371789855643, -8.962234695871567070 ) ) ;
#7180=CARTESIAN_POINT ( 'NONE',  ( 10.69584247140445221, 99.24768628210145494, -6.932735513423970097 ) ) ;
#7186=CARTESIAN_POINT ( 'NONE',  ( 15.50000000000000533, 75.48981371789854222, -0.1745138560722452326 ) ) ;
#7192=CARTESIAN_POINT ( 'NONE',  ( 8.152565276336593669, 48.75231371789854506, 5.233372021372610483 ) ) ;
#7195=CARTESIAN_POINT ( 'NONE',  ( -5.529263428287297444, 109.1273137178985451, -7.954856959092311719 ) ) ;
#7197=CARTESIAN_POINT ( 'NONE',  ( -10.49813415416004858, 33.22731371789855359, 7.228626920338839135 ) ) ;
#7198=CARTESIAN_POINT ( 'NONE',  ( -2.311890736173176641, 79.12268628210145494, -12.53471296425194836 ) ) ;
#7207=CARTESIAN_POINT ( 'NONE',  ( -5.529263428287477744, 103.2726862821014322, 7.954856959092191815 ) ) ;
#7209=CARTESIAN_POINT ( 'NONE',  ( -8.962234695871760692, 131.1601862821014777, 8.715434833791933400 ) ) ;
#7220=CARTESIAN_POINT ( 'NONE',  ( -3.796722387233185003, 8.214813717898532985, -8.710071997420207879 ) ) ;
#7225=CARTESIAN_POINT ( 'NONE',  ( 8.962234695871567070, 30.63981371789854791, 8.715434833792127023 ) ) ;
#7227=CARTESIAN_POINT ( 'NONE',  ( 15.53471296425188797, 140.1773137178985564, 2.908627838312457747 ) ) ;
#7233=CARTESIAN_POINT ( 'NONE',  ( 12.46528703574805874, 127.9976862821014407, 2.660918448318279950 ) ) ;
#7243=CARTESIAN_POINT ( 'NONE',  ( -11.08355503943142573, 121.9601862821014606, 10.83675517735155402 ) ) ;
#7245=CARTESIAN_POINT ( 'NONE',  ( 9.534712964251941258, 118.2226862821014493, -1.715153634034235708 ) ) ;
#7247=CARTESIAN_POINT ( 'NONE',  ( 8.962234695871762469, 6.960186282101432198, -8.715434833791931624 ) ) ;
#7251=CARTESIAN_POINT ( 'NONE',  ( 9.534712964251941258, 72.22268628210143504, -1.715153634034235708 ) ) ;
#7253=CARTESIAN_POINT ( 'NONE',  ( 8.843639120294245259, 131.2648137178985621, 3.474262827703527901 ) ) ;
#7259=CARTESIAN_POINT ( 'NONE',  ( -9.500000000000005329, 80.08981371789856496, 0.1745138560723101806 ) ) ;
#7262=CARTESIAN_POINT ( 'NONE',  ( -11.48171059495408208, 79.51481371789856212, 4.944772684328421875 ) ) ;
#7266=CARTESIAN_POINT ( 'NONE',  ( -2.660918448318004614, 45.30231371789855643, -12.46528703574811558 ) ) ;
#7270=CARTESIAN_POINT ( 'NONE',  ( -11.48171059495397373, 22.48518628210144499, -4.944772684328680334 ) ) ;
#7276=CARTESIAN_POINT ( 'NONE',  ( -8.962234695871565293, 62.83981371789855785, -8.715434833792128799 ) ) ;
#7281=CARTESIAN_POINT ( 'NONE',  ( -10.83675517735179028, 60.53981371789856070, 11.08355503943118947 ) ) ;
#7284=CARTESIAN_POINT ( 'NONE',  ( -6.932735513423968321, 69.34768628210143504, -10.69584247140445221 ) ) ;
#7285=CARTESIAN_POINT ( 'NONE',  ( -15.53471296425195369, 30.82268628210143291, 2.908627838312118019 ) ) ;
#7290=CARTESIAN_POINT ( 'NONE',  ( -13.04141134922759804, 31.97268628210143149, -8.927990412390657937 ) ) ;
#7296=CARTESIAN_POINT ( 'NONE',  ( -2.660918448318275509, 29.09768628210144925, 12.46528703574805874 ) ) ;
#7298=CARTESIAN_POINT ( 'NONE',  ( 6.594114490232462877, 138.7398137178985564, -6.840914352311949109 ) ) ;
#7304=CARTESIAN_POINT ( 'NONE',  ( -4.622313124798826500, 142.7648137178985621, 11.61527771782809637 ) ) ;
#7310=CARTESIAN_POINT ( 'NONE',  ( 4.622313124798573369, 37.43518628210144783, 11.61527771782819940 ) ) ;
#7318=CARTESIAN_POINT ( 'NONE',  ( 4.622313124798573369, 83.43518628210145494, 11.61527771782819940 ) ) ;
#7319=CARTESIAN_POINT ( 'NONE',  ( -8.632099005475501130, 133.7476862821013981, -13.23911966647218996 ) ) ;
#7325=CARTESIAN_POINT ( 'NONE',  ( 7.954856959092311719, 10.22731371789853405, -5.529263428287300108 ) ) ;
#7333=CARTESIAN_POINT ( 'NONE',  ( -5.770363421894122880, 115.1648137178985678, 14.38691631536194393 ) ) ;
#7338=CARTESIAN_POINT ( 'NONE',  ( 4.944772684328679446, 135.1851862821014549, -11.48171059495397373 ) ) ;
#7341=CARTESIAN_POINT ( 'NONE',  ( -15.50000000000000533, 95.51018628210147199, -0.1745138560725808530 ) ) ;
#7345=CARTESIAN_POINT ( 'NONE',  ( 5.233372021372432847, 37.14768628210143220, 8.152565276336710909 ) ) ;
#7349=CARTESIAN_POINT ( 'NONE',  ( -10.49813415415989581, 68.77268628210146062, -7.228626920339068285 ) ) ;
#7352=CARTESIAN_POINT ( 'NONE',  ( -2.064181346179269738, 38.29768628210144499, 9.465287035748067623 ) ) ;
#7361=CARTESIAN_POINT ( 'NONE',  ( 8.962234695871567070, 76.63981371789856212, 8.715434833792127023 ) ) ;
#7362=CARTESIAN_POINT ( 'NONE',  ( 10.69584247140445221, 90.04768628210145209, -6.932735513423970097 ) ) ;
#7368=CARTESIAN_POINT ( 'NONE',  ( -3.257655550456946880, 54.50231371789855928, -15.46528703574811736 ) ) ;
#7374=CARTESIAN_POINT ( 'NONE',  ( -9.500000000000005329, 61.68981371789855928, 0.1745138560723101806 ) ) ;
#7376=CARTESIAN_POINT ( 'NONE',  ( 1.715153634034445762, 110.2773137178985650, -9.534712964251895073 ) ) ;
#7378=CARTESIAN_POINT ( 'NONE',  ( -2.660918448318004614, 26.90231371789854364, -12.46528703574811558 ) ) ;
#7380=CARTESIAN_POINT ( 'NONE',  ( -4.944772684328673229, 84.58518628210146062, 11.48171059495397728 ) ) ;
#7386=CARTESIAN_POINT ( 'NONE',  ( 7.954856959092191815, 91.77268628210144641, 5.529263428287477744 ) ) ;
#7388=CARTESIAN_POINT ( 'NONE',  ( 8.962234695871762469, 126.5601862821014691, -8.715434833791931624 ) ) ;
#7395=( BOUNDED_CURVE ( )  B_SPLINE_CURVE ( 2, ( #8153, #33547, #19727, #2261, #16310, #4916, #11171, #22555, #18972, #30527, #19535, #27856, #1889, #16497, #13652, #31265, #4549, #5291, #2447, #10798, #33919, #7962, #16686, #28232, #13840, #28408, #25387, #36937, #10983, #14022, #25571, #37124, #12095, #31448, #35031, #23669, #14765, #19907, #28592, #32192, #28966, #5849, #6226, #3006, #34655, #11359, #8337, #11540, #23112, #5659, #9076, #14389, #8518, #528, #5471, #17427, #8700, #14206, #2818, #14575, #29148, #26127, #32002, #20274, #37489, #17054, #2629, #20085, #31813, #25757, #159, #37309, #31629, #11726, #22930, #23298, #34845, #25946, #34475, #17800, #8883, #17239, #28780, #20461, #6032, #17618, #3189, #26310, #347, #20645, #11912, #23478, #29342, #3381, #14949, #26497, #29533, #27073, #3574, #18564, #18365, #35592, #9637, #29719, #21400, #15134, #13048, #30293, #29913, #26686, #4136, #3943, #35779, #23861, #35970, #24422, #35400, #24047, #716, #30105, #21214, #12666, #3753, #15708, #35214, #9822, #27259, #15897, #10007, #1282, #21027, #910, #32753, #21589, #32562, #9263, #6790, #4318, #24234, #33136, #32940, #15519, #1098, #12479, #6604, #1474, #6994, #7180, #9450, #12854, #18751, #18179, #20835, #27443, #32378, #12289, #6417, #17990, #15327, #26879, #28369, #19682, #19496, #22515, #13613, #24787, #16827, #2405, #21959, #34062, #27820, #24966, #1849, #10383, #18934, #8110, #4878, #4689, #30673, #7362, #13237, #10756, #19315, #16271, #33504, #33880, #10568, #19122, #36525, #2217, #7549, #31221, #22145, #33693, #7732, #30487, #36716, #5251, #13418, #31043, #24604, #30853, #16458, #2034, #36153, #25161, #22328, #10197, #5064, #7922, #16645, #28187, #28002, #13799, #21773, #25348, #36894, #10942, #33323, #4508, #16084, #27634, #1663, #36337, #34249, #2958, #29102, #6178, #3145, #5427, #14714, #34797, #17008, #17195, #17750, #17567, #29292, #13978, #14527, #14161, #37268, #37447, #8654, #28734, #22882, #25529, #26083, #23431, #25715, #17382, #2773, #11314, #37082, #26263, #23252, #19864, #34612, #112, #31407, #20413, #11129, #9026, #8841, #11862, #11678, #34433, #22707, #20224, #25899, #11496, #8292, #31956, #28548, #34983, #5988, #8470, #297, #20598, #32138, #2590, #20042, #31586, #5610, #23065, #14346, #5800, #31768, #28923, #3520, #32701, #24182, #9958, #29859, #12801, #35727, #27020, #32890, #9773, #859, #12429, #7128, #15086, #29671, #20784, #21350, #15275, #32510, #6942, #6555, #9213, #23620, #3895, #18511, #33085, #30050, #32328, #4084, #15656, #6367, #18129, #18700, #3705, #35915, #15466, #27206, #1045, #26828, #23998, #35544, #9588, #12237, #3330, #12617, #24371, #26636, #6742, #21162, #666, #14901, #1230, #21539, #17938, #18317, #35165, #26450, #482, #29482, #12049, #23808, #35350, #9402, #20977, #30993, #4639, #21904, #7494, #12998, #7682, #15842, #22279, #24920, #1611, #7310, #19443, #5012, #19070, #36286, #24554, #27582, #30622, #19262, #1798, #36104, #36473, #18883, #27768, #30801, #7869, #30241, #4453, #33832, #27390, #30434, #10514, #10147, #33453, #16218, #13181, #1420, #10702, #10333, #16033, #33643, #13365, #22093, #24735, #4824, #16405, #27951, #1982, #13553, #4268, #25107, #36664, #21720, #33271, #5494, #36965, #25596, #34679, #32022, #2653, #14229, #34316, #25967, #19752, #14412, #28615, #25780, #34498, #17076, #14600, #23318, #8540, #16894, #37151, #22582, #6053, #14046, #184, #37330, #22953, #28433, #11380, #34127, #5690, #20106, #5318, #34867, #8724, #11750, #2473, #17640, #31654, #5681, #17263, #8177, #23137, #11009, #8909, #28803, #11192, #26151, #20484, #2288, #22767, #13864, #2840, #31470, #31290, #19932, #11564, #8361, #20296, #31838, #5871, #17449, #25412, #28987, #3028, #1122, #32401, #29558, #6441, #14974, #23505, #27098, #9475, #9288, #35238, #11934 ),
 .UNSPECIFIED., .F., .F. ) 
 B_SPLINE_CURVE_WITH_KNOTS ( ( 3, 2, 2, 2, 2, 2, 2, 2, 2, 2, 2, 2, 2, 2, 2, 2, 2, 2, 2, 2, 2, 2, 2, 2, 2, 2, 2, 2, 2, 2, 2, 2, 2, 2, 2, 2, 2, 2, 2, 2, 2, 2, 2, 2, 2, 2, 2, 2, 2, 2, 2, 2, 2, 2, 2, 2, 2, 2, 2, 2, 2, 2, 2, 2, 2, 2, 2, 2, 2, 2, 2, 2, 2, 2, 2, 2, 2, 2, 2, 2, 2, 2, 2, 2, 2, 2, 2, 2, 2, 2, 2, 2, 2, 2, 2, 2, 2, 2, 2, 2, 2, 2, 2, 2, 2, 2, 2, 2, 2, 2, 2, 2, 2, 2, 2, 2, 2, 2, 2, 2, 2, 2, 2, 2, 2, 2, 2, 2, 2, 2, 2, 2, 2, 2, 2, 2, 2, 2, 2, 2, 2, 2, 2, 2, 2, 2, 2, 2, 2, 2, 2, 2, 2, 2, 2, 2, 2, 2, 2, 2, 2, 2, 2, 2, 2, 2, 2, 2, 2, 2, 2, 2, 2, 2, 2, 2, 2, 2, 2, 2, 2, 2, 2, 2, 2, 2, 2, 2, 2, 2, 2, 2, 2, 2, 2, 2, 2, 2, 2, 2, 2, 2, 2, 2, 2, 2, 2, 2, 2, 2, 2, 2, 2, 2, 2, 2, 2, 2, 2, 2, 2, 2, 2, 2, 2, 2, 2, 2, 2, 2, 2, 2, 2, 2, 2, 2, 2, 2, 2, 2, 3 ),
 ( 0.000000000000000000, 0.004166666666666666609, 0.008333333333333333218, 0.01250000000000000069, 0.01666666666666666644, 0.02083333333333333218, 0.02500000000000000139, 0.02916666666666666713, 0.03333333333333333287, 0.03749999999999999861, 0.04166666666666666435, 0.04583333333333333010, 0.05000000000000000278, 0.05416666666666666852, 0.05833333333333333426, 0.06250000000000000000, 0.06666666666666666574, 0.07083333333333333148, 0.07499999999999999722, 0.07916666666666666297, 0.08333333333333332871, 0.08749999999999999445, 0.09166666666666666019, 0.09583333333333333981, 0.1000000000000000056, 0.1041666666666666713, 0.1083333333333333370, 0.1125000000000000028, 0.1166666666666666685, 0.1208333333333333343, 0.1250000000000000000, 0.1291666666666666796, 0.1333333333333333315, 0.1375000000000000111, 0.1416666666666666630, 0.1458333333333333426, 0.1499999999999999944, 0.1541666666666666741, 0.1583333333333333259, 0.1625000000000000056, 0.1666666666666666574, 0.1708333333333333370, 0.1749999999999999889, 0.1791666666666666685, 0.1833333333333333204, 0.1875000000000000000, 0.1916666666666666796, 0.1958333333333333315, 0.2000000000000000111, 0.2041666666666666630, 0.2083333333333333426, 0.2124999999999999944, 0.2166666666666666741, 0.2208333333333333259, 0.2250000000000000056, 0.2291666666666666574, 0.2333333333333333370, 0.2374999999999999889, 0.2416666666666666685, 0.2458333333333333204, 0.2500000000000000000, 0.2541666666666666519, 0.2583333333333333592, 0.2625000000000000111, 0.2666666666666666630, 0.2708333333333333148, 0.2750000000000000222, 0.2791666666666666741, 0.2833333333333333259, 0.2874999999999999778, 0.2916666666666666852, 0.2958333333333333370, 0.2999999999999999889, 0.3041666666666666408, 0.3083333333333333481, 0.3125000000000000000, 0.3166666666666666519, 0.3208333333333333592, 0.3250000000000000111, 0.3291666666666666630, 0.3333333333333333148, 0.3375000000000000222, 0.3416666666666666741, 0.3458333333333333259, 0.3499999999999999778, 0.3541666666666666852, 0.3583333333333333370, 0.3624999999999999889, 0.3666666666666666408, 0.3708333333333333481, 0.3750000000000000000, 0.3791666666666666519, 0.3833333333333333592, 0.3875000000000000111, 0.3916666666666666630, 0.3958333333333333148, 0.4000000000000000222, 0.4041666666666666741, 0.4083333333333333259, 0.4124999999999999778, 0.4166666666666666852, 0.4208333333333333370, 0.4249999999999999889, 0.4291666666666666408, 0.4333333333333333481, 0.4375000000000000000, 0.4416666666666666519, 0.4458333333333333592, 0.4500000000000000111, 0.4541666666666666630, 0.4583333333333333148, 0.4625000000000000222, 0.4666666666666666741, 0.4708333333333333259, 0.4749999999999999778, 0.4791666666666666852, 0.4833333333333333370, 0.4874999999999999889, 0.4916666666666666408, 0.4958333333333333481, 0.5000000000000000000, 0.5041666666666666519, 0.5083333333333333037, 0.5124999999999999556, 0.5166666666666667185, 0.5208333333333333703, 0.5250000000000000222, 0.5291666666666666741, 0.5333333333333333259, 0.5374999999999999778, 0.5416666666666666297, 0.5458333333333332815, 0.5500000000000000444, 0.5541666666666666963, 0.5583333333333333481, 0.5625000000000000000, 0.5666666666666666519, 0.5708333333333333037, 0.5749999999999999556, 0.5791666666666667185, 0.5833333333333333703, 0.5875000000000000222, 0.5916666666666666741, 0.5958333333333333259, 0.5999999999999999778, 0.6041666666666666297, 0.6083333333333332815, 0.6125000000000000444, 0.6166666666666666963, 0.6208333333333333481, 0.6250000000000000000, 0.6291666666666666519, 0.6333333333333333037, 0.6374999999999999556, 0.6416666666666667185, 0.6458333333333333703, 0.6500000000000000222, 0.6541666666666666741, 0.6583333333333333259, 0.6624999999999999778, 0.6666666666666666297, 0.6708333333333332815, 0.6750000000000000444, 0.6791666666666666963, 0.6833333333333333481, 0.6875000000000000000, 0.6916666666666666519, 0.6958333333333333037, 0.6999999999999999556, 0.7041666666666667185, 0.7083333333333333703, 0.7125000000000000222, 0.7166666666666666741, 0.7208333333333333259, 0.7249999999999999778, 0.7291666666666666297, 0.7333333333333332815, 0.7375000000000000444, 0.7416666666666666963, 0.7458333333333333481, 0.7500000000000000000, 0.7541666666666666519, 0.7583333333333333037, 0.7624999999999999556, 0.7666666666666667185, 0.7708333333333333703, 0.7750000000000000222, 0.7791666666666666741, 0.7833333333333333259, 0.7874999999999999778, 0.7916666666666666297, 0.7958333333333332815, 0.8000000000000000444, 0.8041666666666666963, 0.8083333333333333481, 0.8125000000000000000, 0.8166666666666666519, 0.8208333333333333037, 0.8249999999999999556, 0.8291666666666667185, 0.8333333333333333703, 0.8375000000000000222, 0.8416666666666666741, 0.8458333333333333259, 0.8499999999999999778, 0.8541666666666666297, 0.8583333333333332815, 0.8625000000000000444, 0.8666666666666666963, 0.8708333333333333481, 0.8750000000000000000, 0.8791666666666666519, 0.8833333333333333037, 0.8874999999999999556, 0.8916666666666667185, 0.8958333333333333703, 0.9000000000000000222, 0.9041666666666666741, 0.9083333333333333259, 0.9124999999999999778, 0.9166666666666666297, 0.9208333333333332815, 0.9250000000000000444, 0.9291666666666666963, 0.9333333333333333481, 0.9375000000000000000, 0.9416666666666666519, 0.9458333333333333037, 0.9499999999999999556, 0.9541666666666667185, 0.9583333333333333703, 0.9625000000000000222, 0.9666666666666666741, 0.9708333333333333259, 0.9749999999999999778, 0.9791666666666666297, 0.9833333333333332815, 0.9875000000000000444, 0.9916666666666666963, 0.9958333333333333481, 1.000000000000000000 ),
 .UNSPECIFIED. ) 
 CURVE ( )  GEOMETRIC_REPRESENTATION_ITEM ( )  RATIONAL_B_SPLINE_CURVE ( ( 1.000000000000000000, 0.9807852804032304306, 1.000000000000000000, 0.9807852804032304306, 1.000000000000000000, 0.9807852804032304306, 1.000000000000000000, 0.9807852804032304306, 1.000000000000000000, 0.9807852804032304306, 1.000000000000000000, 0.9807852804032304306, 1.000000000000000000, 0.9807852804032304306, 1.000000000000000000, 0.9807852804032304306, 1.000000000000000000, 0.9807852804032304306, 1.000000000000000000, 0.9807852804032304306, 1.000000000000000000, 0.9807852804032304306, 1.000000000000000000, 0.9807852804032304306, 1.000000000000000000, 0.9807852804032304306, 1.000000000000000000, 0.9807852804032304306, 1.000000000000000000, 0.9807852804032304306, 1.000000000000000000, 0.9807852804032304306, 1.000000000000000000, 0.9807852804032304306, 1.000000000000000000, 0.9807852804032304306, 1.000000000000000000, 0.9807852804032304306, 1.000000000000000000, 0.9807852804032304306, 1.000000000000000000, 0.9807852804032304306, 1.000000000000000000, 0.9807852804032304306, 1.000000000000000000, 0.9807852804032304306, 1.000000000000000000, 0.9807852804032304306, 1.000000000000000000, 0.9807852804032304306, 1.000000000000000000, 0.9807852804032304306, 1.000000000000000000, 0.9807852804032304306, 1.000000000000000000, 0.9807852804032304306, 1.000000000000000000, 0.9807852804032304306, 1.000000000000000000, 0.9807852804032304306, 1.000000000000000000, 0.9807852804032304306, 1.000000000000000000, 0.9807852804032304306, 1.000000000000000000, 0.9807852804032304306, 1.000000000000000000, 0.9807852804032304306, 1.000000000000000000, 0.9807852804032304306, 1.000000000000000000, 0.9807852804032304306, 1.000000000000000000, 0.9807852804032304306, 1.000000000000000000, 0.9807852804032304306, 1.000000000000000000, 0.9807852804032304306, 1.000000000000000000, 0.9807852804032304306, 1.000000000000000000, 0.9807852804032304306, 1.000000000000000000, 0.9807852804032304306, 1.000000000000000000, 0.9807852804032304306, 1.000000000000000000, 0.9807852804032304306, 1.000000000000000000, 0.9807852804032304306, 1.000000000000000000, 0.9807852804032304306, 1.000000000000000000, 0.9807852804032304306, 1.000000000000000000, 0.9807852804032304306, 1.000000000000000000, 0.9807852804032304306, 1.000000000000000000, 0.9807852804032304306, 1.000000000000000000, 0.9807852804032304306, 1.000000000000000000, 0.9807852804032304306, 1.000000000000000000, 0.9807852804032304306, 1.000000000000000000, 0.9807852804032304306, 1.000000000000000000, 0.9807852804032304306, 1.000000000000000000, 0.9807852804032304306, 1.000000000000000000, 0.9807852804032304306, 1.000000000000000000, 0.9807852804032304306, 1.000000000000000000, 0.9807852804032304306, 1.000000000000000000, 0.9807852804032304306, 1.000000000000000000, 0.9807852804032304306, 1.000000000000000000, 0.9807852804032304306, 1.000000000000000000, 0.9807852804032304306, 1.000000000000000000, 0.9807852804032304306, 1.000000000000000000, 0.9807852804032304306, 1.000000000000000000, 0.9807852804032304306, 1.000000000000000000, 0.9807852804032304306, 1.000000000000000000, 0.9807852804032304306, 1.000000000000000000, 0.9807852804032304306, 1.000000000000000000, 0.9807852804032304306, 1.000000000000000000, 0.9807852804032304306, 1.000000000000000000, 0.9807852804032304306, 1.000000000000000000, 0.9807852804032304306, 1.000000000000000000, 0.9807852804032304306, 1.000000000000000000, 0.9807852804032304306, 1.000000000000000000, 0.9807852804032304306, 1.000000000000000000, 0.9807852804032304306, 1.000000000000000000, 0.9807852804032304306, 1.000000000000000000, 0.9807852804032304306, 1.000000000000000000, 0.9807852804032304306, 1.000000000000000000, 0.9807852804032304306, 1.000000000000000000, 0.9807852804032304306, 1.000000000000000000, 0.9807852804032304306, 1.000000000000000000, 0.9807852804032304306, 1.000000000000000000, 0.9807852804032304306, 1.000000000000000000, 0.9807852804032304306, 1.000000000000000000, 0.9807852804032304306, 1.000000000000000000, 0.9807852804032304306, 1.000000000000000000, 0.9807852804032304306, 1.000000000000000000, 0.9807852804032304306, 1.000000000000000000, 0.9807852804032304306, 1.000000000000000000, 0.9807852804032304306, 1.000000000000000000, 0.9807852804032304306, 1.000000000000000000, 0.9807852804032304306, 1.000000000000000000, 0.9807852804032304306, 1.000000000000000000, 0.9807852804032304306, 1.000000000000000000, 0.9807852804032304306, 1.000000000000000000, 0.9807852804032304306, 1.000000000000000000, 0.9807852804032304306, 1.000000000000000000, 0.9807852804032304306, 1.000000000000000000, 0.9807852804032304306, 1.000000000000000000, 0.9807852804032304306, 1.000000000000000000, 0.9807852804032304306, 1.000000000000000000, 0.9807852804032304306, 1.000000000000000000, 0.9807852804032304306, 1.000000000000000000, 0.9807852804032304306, 1.000000000000000000, 0.9807852804032304306, 1.000000000000000000, 0.9807852804032304306, 1.000000000000000000, 0.9807852804032304306, 1.000000000000000000, 0.9807852804032304306, 1.000000000000000000, 0.9807852804032304306, 1.000000000000000000, 0.9807852804032304306, 1.000000000000000000, 0.9807852804032304306, 1.000000000000000000, 0.9807852804032304306, 1.000000000000000000, 0.9807852804032304306, 1.000000000000000000, 0.9807852804032304306, 1.000000000000000000, 0.9807852804032304306, 1.000000000000000000, 0.9807852804032304306, 1.000000000000000000, 0.9807852804032304306, 1.000000000000000000, 0.9807852804032304306, 1.000000000000000000, 0.9807852804032304306, 1.000000000000000000, 0.9807852804032304306, 1.000000000000000000, 0.9807852804032304306, 1.000000000000000000, 0.9807852804032304306, 1.000000000000000000, 0.9807852804032304306, 1.000000000000000000, 0.9807852804032304306, 1.000000000000000000, 0.9807852804032304306, 1.000000000000000000, 0.9807852804032304306, 1.000000000000000000, 0.9807852804032304306, 1.000000000000000000, 0.9807852804032304306, 1.000000000000000000, 0.9807852804032304306, 1.000000000000000000, 0.9807852804032304306, 1.000000000000000000, 0.9807852804032304306, 1.000000000000000000, 0.9807852804032304306, 1.000000000000000000, 0.9807852804032304306, 1.000000000000000000, 0.9807852804032304306, 1.000000000000000000, 0.9807852804032304306, 1.000000000000000000, 0.9807852804032304306, 1.000000000000000000, 0.9807852804032304306, 1.000000000000000000, 0.9807852804032304306, 1.000000000000000000, 0.9807852804032304306, 1.000000000000000000, 0.9807852804032304306, 1.000000000000000000, 0.9807852804032304306, 1.000000000000000000, 0.9807852804032304306, 1.000000000000000000, 0.9807852804032304306, 1.000000000000000000, 0.9807852804032304306, 1.000000000000000000, 0.9807852804032304306, 1.000000000000000000, 0.9807852804032304306, 1.000000000000000000, 0.9807852804032304306, 1.000000000000000000, 0.9807852804032304306, 1.000000000000000000, 0.9807852804032304306, 1.000000000000000000, 0.9807852804032304306, 1.000000000000000000, 0.9807852804032304306, 1.000000000000000000, 0.9807852804032304306, 1.000000000000000000, 0.9807852804032304306, 1.000000000000000000, 0.9807852804032304306, 1.000000000000000000, 0.9807852804032304306, 1.000000000000000000, 0.9807852804032304306, 1.000000000000000000, 0.9807852804032304306, 1.000000000000000000, 0.9807852804032304306, 1.000000000000000000, 0.9807852804032304306, 1.000000000000000000, 0.9807852804032304306, 1.000000000000000000, 0.9807852804032304306, 1.000000000000000000, 0.9807852804032304306, 1.000000000000000000, 0.9807852804032304306, 1.000000000000000000, 0.9807852804032304306, 1.000000000000000000, 0.9807852804032304306, 1.000000000000000000, 0.9807852804032304306, 1.000000000000000000, 0.9807852804032304306, 1.000000000000000000, 0.9807852804032304306, 1.000000000000000000, 0.9807852804032304306, 1.000000000000000000, 0.9807852804032304306, 1.000000000000000000, 0.9807852804032304306, 1.000000000000000000, 0.9807852804032304306, 1.000000000000000000, 0.9807852804032304306, 1.000000000000000000, 0.9807852804032304306, 1.000000000000000000, 0.9807852804032304306, 1.000000000000000000, 0.9807852804032304306, 1.000000000000000000, 0.9807852804032304306, 1.000000000000000000, 0.9807852804032304306, 1.000000000000000000, 0.9807852804032304306, 1.000000000000000000, 0.9807852804032304306, 1.000000000000000000, 0.9807852804032304306, 1.000000000000000000, 0.9807852804032304306, 1.000000000000000000, 0.9807852804032304306, 1.000000000000000000, 0.9807852804032304306, 1.000000000000000000, 0.9807852804032304306, 1.000000000000000000, 0.9807852804032304306, 1.000000000000000000, 0.9807852804032304306, 1.000000000000000000, 0.9807852804032304306, 1.000000000000000000, 0.9807852804032304306, 1.000000000000000000, 0.9807852804032304306, 1.000000000000000000, 0.9807852804032304306, 1.000000000000000000, 0.9807852804032304306, 1.000000000000000000, 0.9807852804032304306, 1.000000000000000000, 0.9807852804032304306, 1.000000000000000000, 0.9807852804032304306, 1.000000000000000000, 0.9807852804032304306, 1.000000000000000000, 0.9807852804032304306, 1.000000000000000000, 0.9807852804032304306, 1.000000000000000000, 0.9807852804032304306, 1.000000000000000000, 0.9807852804032304306, 1.000000000000000000, 0.9807852804032304306, 1.000000000000000000, 0.9807852804032304306, 1.000000000000000000, 0.9807852804032304306, 1.000000000000000000, 0.9807852804032304306, 1.000000000000000000, 0.9807852804032304306, 1.000000000000000000, 0.9807852804032304306, 1.000000000000000000, 0.9807852804032304306, 1.000000000000000000, 0.9807852804032304306, 1.000000000000000000, 0.9807852804032304306, 1.000000000000000000, 0.9807852804032304306, 1.000000000000000000, 0.9807852804032304306, 1.000000000000000000, 0.9807852804032304306, 1.000000000000000000, 0.9807852804032304306, 1.000000000000000000, 0.9807852804032304306, 1.000000000000000000, 0.9807852804032304306, 1.000000000000000000, 0.9807852804032304306, 1.000000000000000000, 0.9807852804032304306, 1.000000000000000000, 0.9807852804032304306, 1.000000000000000000, 0.9807852804032304306, 1.000000000000000000, 0.9807852804032304306, 1.000000000000000000, 0.9807852804032304306, 1.000000000000000000, 0.9807852804032304306, 1.000000000000000000, 0.9807852804032304306, 1.000000000000000000, 0.9807852804032304306, 1.000000000000000000, 0.9807852804032304306, 1.000000000000000000, 0.9807852804032304306, 1.000000000000000000, 0.9807852804032304306, 1.000000000000000000, 0.9807852804032304306, 1.000000000000000000, 0.9807852804032304306, 1.000000000000000000, 0.9807852804032304306, 1.000000000000000000, 0.9807852804032304306, 1.000000000000000000, 0.9807852804032304306, 1.000000000000000000, 0.9807852804032304306, 1.000000000000000000, 0.9807852804032304306, 1.000000000000000000, 0.9807852804032304306, 1.000000000000000000, 0.9807852804032304306, 1.000000000000000000, 0.9807852804032304306, 1.000000000000000000, 0.9807852804032304306, 1.000000000000000000 ) ) 
 REPRESENTATION_ITEM ( '' )  );
#7399=CARTESIAN_POINT ( 'NONE',  ( 11.48171059495408208, 139.3148137178985451, -4.944772684328420986 ) ) ;
#7405=CARTESIAN_POINT ( 'NONE',  ( 7.228626920338837358, 21.72731371789854293, 10.49813415416005036 ) ) ;
#7407=CARTESIAN_POINT ( 'NONE',  ( 6.092822981423662299, 104.8148137178985593, 14.25334919248795096 ) ) ;
#7416=CARTESIAN_POINT ( 'NONE',  ( 0.1745138560725515708, 125.4101862821014635, -12.50000000000000355 ) ) ;
#7426=CARTESIAN_POINT ( 'NONE',  ( 4.944772684328679446, 135.1851862821014549, -11.48171059495397373 ) ) ;
#7430=CARTESIAN_POINT ( 'NONE',  ( -8.927990412390661490, 112.4726862821014635, 13.04141134922759804 ) ) ;
#7431=CARTESIAN_POINT ( 'NONE',  ( 6.594114490232313663, 119.6601862821014635, 6.840914352312096547 ) ) ;
#7433=CARTESIAN_POINT ( 'NONE',  ( 2.660918448318279950, 6.097686282101443922, -12.46528703574805697 ) ) ;
#7437=CARTESIAN_POINT ( 'NONE',  ( -6.840914352312096547, 85.16018628210146346, 6.594114490232313663 ) ) ;
#7438=CARTESIAN_POINT ( 'NONE',  ( 6.840914352311949109, 131.8398137178985792, 6.594114490232462877 ) ) ;
#7444=CARTESIAN_POINT ( 'NONE',  ( -9.465287035748106703, 61.40231371789855785, 2.064181346179061460 ) ) ;
#7447=CARTESIAN_POINT ( 'NONE',  ( -6.932735513424201912, 78.65231371789856496, 10.69584247140429412 ) ) ;
#7449=CARTESIAN_POINT ( 'NONE',  ( -14.00000000000001599, 143.0000000000000000, 1.203016833088524695 ) ) ;
#7451=CARTESIAN_POINT ( 'NONE',  ( 4.944772684328420986, 40.41481371789855359, 11.48171059495408208 ) ) ;
#7455=CARTESIAN_POINT ( 'NONE',  ( 6.932735513423970097, 27.94768628210143646, 10.69584247140445044 ) ) ;
#7459=CARTESIAN_POINT ( 'NONE',  ( -11.48171059495408208, 61.11481371789854933, 4.944772684328421875 ) ) ;
#7465=CARTESIAN_POINT ( 'NONE',  ( 14.25334919248795451, 38.11481371789853512, -6.092822981423661410 ) ) ;
#7469=CARTESIAN_POINT ( 'NONE',  ( -8.962234695871760692, 66.76018628210145778, 8.715434833791933400 ) ) ;
#7470=CARTESIAN_POINT ( 'NONE',  ( -15.53471296425195369, 12.42268628210144144, 2.908627838312118019 ) ) ;
#7474=CARTESIAN_POINT ( 'NONE',  ( -14.25334919248782306, 22.48518628210144499, -6.092822981423979378 ) ) ;
#7482=CARTESIAN_POINT ( 'NONE',  ( 0.1745138560723095977, 114.5898137178985650, 9.500000000000005329 ) ) ;
#7488=CARTESIAN_POINT ( 'NONE',  ( 2.660918448318003282, 141.9023137178985792, 12.46528703574811558 ) ) ;
#7494=CARTESIAN_POINT ( 'NONE',  ( -10.69584247140444866, 39.44768628210145067, 6.932735513423972762 ) ) ;
#7503=CARTESIAN_POINT ( 'NONE',  ( 2.311890736173175753, 83.72268628210143504, 12.53471296425194836 ) ) ;
#7504=CARTESIAN_POINT ( 'NONE',  ( -13.23911966647199812, 7.352313717898546486, -8.632099005475788900 ) ) ;
#7511=CARTESIAN_POINT ( 'NONE',  ( -10.69584247140429412, 117.7523137178986019, -6.932735513424201024 ) ) ;
#7518=CARTESIAN_POINT ( 'NONE',  ( 13.23911966647199812, 94.75231371789854506, 8.632099005475788900 ) ) ;
#7522=CARTESIAN_POINT ( 'NONE',  ( -8.962234695871760692, 121.9601862821014464, 8.715434833791933400 ) ) ;
#7523=CARTESIAN_POINT ( 'NONE',  ( -13.23911966647218463, 76.24768628210145494, 8.632099005475506459 ) ) ;
#7527=CARTESIAN_POINT ( 'NONE',  ( 15.50000000000000533, 81.71018628210144641, 0.1745138560725827404 ) ) ;
#7531=CARTESIAN_POINT ( 'NONE',  ( -8.152565276336710909, 39.44768628210144357, 5.233372021372435512 ) ) ;
#7536=CARTESIAN_POINT ( 'NONE',  ( 4.622313124798573369, 65.03518628210144925, 11.61527771782819940 ) ) ;
#7539=CARTESIAN_POINT ( 'NONE',  ( -9.534712964251941258, 49.22268628210144215, 1.715153634034234154 ) ) ;
#7548=CARTESIAN_POINT ( 'NONE',  ( 12.46528703574811558, 93.60231371789855359, -2.660918448318005503 ) ) ;
#7549=CARTESIAN_POINT ( 'NONE',  ( -11.48171059495397373, 86.88518628210145778, -4.944772684328680334 ) ) ;
#7554=CARTESIAN_POINT ( 'NONE',  ( -0.1745138560722442889, 63.98981371789855643, -15.50000000000000533 ) ) ;
#7560=CARTESIAN_POINT ( 'NONE',  ( 8.152565276336593669, 39.55231371789854933, 5.233372021372610483 ) ) ;
#7562=CARTESIAN_POINT ( 'NONE',  ( 9.465287035748106703, 93.60231371789855359, -2.064181346179063237 ) ) ;
#7564=CARTESIAN_POINT ( 'NONE',  ( -6.932735513424201912, 23.45231371789854791, 10.69584247140429412 ) ) ;
#7565=CARTESIAN_POINT ( 'NONE',  ( 10.49813415415989581, 91.77268628210144641, 7.228626920339068285 ) ) ;
#7573=CARTESIAN_POINT ( 'NONE',  ( -6.594114490232312775, 87.46018628210146062, -6.840914352312096547 ) ) ;
#7575=CARTESIAN_POINT ( 'NONE',  ( -12.53471296425194836, 122.8226862821014720, 2.311890736173176641 ) ) ;
#7589=CARTESIAN_POINT ( 'NONE',  ( 3.474262827703532341, 9.364813717898543999, -8.843639120294245259 ) ) ;
#7596=CARTESIAN_POINT ( 'NONE',  ( 0.1745138560722461762, 105.3898137178985479, 15.50000000000000533 ) ) ;
#7602=CARTESIAN_POINT ( 'NONE',  ( 11.61527771782819940, 136.3351862821014606, -4.622313124798573369 ) ) ;
#7609=CARTESIAN_POINT ( 'NONE',  ( -2.660918448318275509, 130.2976862821014379, 12.46528703574805874 ) ) ;
#7615=CARTESIAN_POINT ( 'NONE',  ( -0.1745138560725817967, 120.8101862821014691, 15.50000000000000533 ) ) ;
#7618=CARTESIAN_POINT ( 'NONE',  ( 7.228626920339068285, 15.87268628210144961, -10.49813415415989581 ) ) ;
#7622=CARTESIAN_POINT ( 'NONE',  ( 8.843639120294328748, 90.33518628210144641, -3.474262827703334722 ) ) ;
#7624=CARTESIAN_POINT ( 'NONE',  ( -3.796722387233185003, 127.8148137178985735, -8.710071997420207879 ) ) ;
#7631=CARTESIAN_POINT ( 'NONE',  ( -8.843639120294245259, 53.06481371789855928, -3.474262827703533230 ) ) ;
#7635=CARTESIAN_POINT ( 'NONE',  ( -2.660918448318005058, 63.70231371789855501, -12.46528703574811558 ) ) ;
#7639=CARTESIAN_POINT ( 'NONE',  ( 0.1745138560722779009, 31.78981371789854649, 12.50000000000000355 ) ) ;
#7649=CARTESIAN_POINT ( 'NONE',  ( 6.932735513424201024, 64.85231371789855359, -10.69584247140429412 ) ) ;
#7654=CARTESIAN_POINT ( 'NONE',  ( 8.927990412390371944, 30.92731371789853867, 13.04141134922778811 ) ) ;
#7656=CARTESIAN_POINT ( 'NONE',  ( 4.944772684328679446, 33.98518628210143788, -11.48171059495397373 ) ) ;
#7658=CARTESIAN_POINT ( 'NONE',  ( -2.311890736173176641, 69.92268628210146630, -12.53471296425194836 ) ) ;
#7659=CARTESIAN_POINT ( 'NONE',  ( 5.770363421893814682, 9.835186282101449962, 14.38691631536207183 ) ) ;
#7664=CARTESIAN_POINT ( 'NONE',  ( -14.25334919248782306, 31.68518628210144428, -6.092822981423979378 ) ) ;
#7672=CARTESIAN_POINT ( 'NONE',  ( -8.843639120294245259, 108.2648137178985621, -3.474262827703533230 ) ) ;
#7676=CARTESIAN_POINT ( 'NONE',  ( -4.622313124798826500, 124.3648137178985706, 11.61527771782809637 ) ) ;
#7682=CARTESIAN_POINT ( 'NONE',  ( -7.228626920339070061, 38.87268628210144072, 10.49813415415989404 ) ) ;
#7689=CARTESIAN_POINT ( 'NONE',  ( -11.48171059495397373, 68.48518628210145209, -4.944772684328680334 ) ) ;
#7690=CARTESIAN_POINT ( 'NONE',  ( 11.08355503943142750, 135.7601862821014720, -10.83675517735155225 ) ) ;
#7697=CARTESIAN_POINT ( 'NONE',  ( -11.61527771782809282, 126.6648137178985678, -4.622313124798832717 ) ) ;
#7702=CARTESIAN_POINT ( 'NONE',  ( 8.632099005475788900, 101.6523137178985792, -13.23911966647199812 ) ) ;
#7707=CARTESIAN_POINT ( 'NONE',  ( 7.228626920339068285, 117.0726862821014720, -10.49813415415989581 ) ) ;
#7708=CARTESIAN_POINT ( 'NONE',  ( 6.092822981423978490, 61.58518628210146062, -14.25334919248782306 ) ) ;
#7711=CARTESIAN_POINT ( 'NONE',  ( -0.1745138560725817967, 93.21018628210146062, 15.50000000000000533 ) ) ;
#7714=CARTESIAN_POINT ( 'NONE',  ( -9.500000000000005329, 31.11018628210143433, -0.1745138560725176813 ) ) ;
#7718=CARTESIAN_POINT ( 'NONE',  ( 11.61527771782819940, 62.73518628210145209, -4.622313124798573369 ) ) ;
#7721=CARTESIAN_POINT ( 'NONE',  ( 0.1745138560725194299, 33.41018628210144925, -9.500000000000005329 ) ) ;
#7731=CARTESIAN_POINT ( 'NONE',  ( 8.715434833792128799, 83.53981371789856780, -8.962234695871567070 ) ) ;
#7732=CARTESIAN_POINT ( 'NONE',  ( -11.61527771782819940, 85.73518628210143788, 4.622313124798574258 ) ) ;
#7733=ORIENTED_EDGE ( 'NONE', *, *, #20597, .F. ) ;
#7737=CARTESIAN_POINT ( 'NONE',  ( 15.50000000000000533, 57.08981371789855075, -0.1745138560722452326 ) ) ;
#7742=CARTESIAN_POINT ( 'NONE',  ( 7.954856959092311719, 47.02731371789855075, -5.529263428287300108 ) ) ;
#7745=CARTESIAN_POINT ( 'NONE',  ( -6.840914352311947333, 99.63981371789857633, -6.594114490232462877 ) ) ;
#7747=CARTESIAN_POINT ( 'NONE',  ( -8.962234695871565293, 7.639813717898541690, -8.715434833792128799 ) ) ;
#7748=CARTESIAN_POINT ( 'NONE',  ( 11.61527771782819940, 62.73518628210145209, -4.622313124798573369 ) ) ;
#7751=CARTESIAN_POINT ( 'NONE',  ( 0.000000000000000000, 143.0000000000000000, 0.000000000000000000 ) ) ;
#7753=CARTESIAN_POINT ( 'NONE',  ( -12.50000000000000355, 141.5101862821014720, -0.1745138560725508214 ) ) ;
#7758=CARTESIAN_POINT ( 'NONE',  ( 0.1745138560725194299, 97.81018628210145494, -9.500000000000005329 ) ) ;
#7761=CARTESIAN_POINT ( 'NONE',  ( -2.660918448318275509, 111.8976862821014606, 12.46528703574805874 ) ) ;
#7762=CARTESIAN_POINT ( 'NONE',  ( -7.433878009488998906, 142.9999999999999716, 9.066021292333855897 ) ) ;
#7775=CARTESIAN_POINT ( 'NONE',  ( 10.49813415416005213, 139.0273137178985507, -7.228626920338837358 ) ) ;
#7780=CARTESIAN_POINT ( 'NONE',  ( -7.228626920338836470, 7.927313717898537782, -10.49813415416005213 ) ) ;
#7782=CARTESIAN_POINT ( 'NONE',  ( 8.927990412390371944, 113.7273137178985678, 13.04141134922778811 ) ) ;
#7789=CARTESIAN_POINT ( 'NONE',  ( -11.61527771782819940, 113.3351862821014606, 4.622313124798574258 ) ) ;
#7796=CARTESIAN_POINT ( 'NONE',  ( 8.962234695871762469, 117.3601862821014521, -8.715434833791931624 ) ) ;
#7803=CARTESIAN_POINT ( 'NONE',  ( 15.53471296425195369, 118.2226862821014493, -2.908627838312120684 ) ) ;
#7806=CARTESIAN_POINT ( 'NONE',  ( -9.500000000000005329, 141.5101862821014720, -0.1745138560725176813 ) ) ;
#7810=CARTESIAN_POINT ( 'NONE',  ( 6.840914352312096547, 89.76018628210145778, -6.594114490232313663 ) ) ;
#7812=CARTESIAN_POINT ( 'NONE',  ( 6.594114490232462877, 129.5398137178985678, -6.840914352311949109 ) ) ;
#7817=CARTESIAN_POINT ( 'NONE',  ( -9.534712964251895073, 52.77731371789855785, -1.715153634034446428 ) ) ;
#7821=CARTESIAN_POINT ( 'NONE',  ( -8.962234695871565293, 62.83981371789855785, -8.715434833792128799 ) ) ;
#7825=CARTESIAN_POINT ( 'NONE',  ( 12.50000000000000355, 38.68981371789855217, -0.1745138560722771515 ) ) ;
#7833=CARTESIAN_POINT ( 'NONE',  ( 0.1745138560722779009, 59.38981371789856212, 12.50000000000000355 ) ) ;
#7840=CARTESIAN_POINT ( 'NONE',  ( -13.04141134922778456, 42.42731371789855643, 8.927990412390377273 ) ) ;
#7842=CARTESIAN_POINT ( 'NONE',  ( 2.660918448318279950, 33.69768628210145067, -12.46528703574805697 ) ) ;
#7844=CARTESIAN_POINT ( 'NONE',  ( 11.48171059495397728, 73.08518628210144641, 4.944772684328674117 ) ) ;
#7845=CARTESIAN_POINT ( 'NONE',  ( -8.927990412390661490, 11.27268628210142865, 13.04141134922759804 ) ) ;
#7849=CARTESIAN_POINT ( 'NONE',  ( 10.83675517735155225, 27.66018628210143859, 11.08355503943142573 ) ) ;
#7855=CARTESIAN_POINT ( 'NONE',  ( -4.622313124798576922, 5.235186282101428112, -11.61527771782819762 ) ) ;
#7858=CARTESIAN_POINT ( 'NONE',  ( 9.465287035748106703, 112.0023137178985451, -2.064181346179063237 ) ) ;
#7863=CARTESIAN_POINT ( 'NONE',  ( 11.61527771782809637, 122.0648137178985735, 4.622313124798827388 ) ) ;
#7869=CARTESIAN_POINT ( 'NONE',  ( -2.311890736173176641, 33.12268628210144072, -12.53471296425194659 ) ) ;
#7877=CARTESIAN_POINT ( 'NONE',  ( 12.50000000000000355, 63.31018628210144072, 0.1745138560725507937 ) ) ;
#7884=CARTESIAN_POINT ( 'NONE',  ( -2.311890736173448424, 114.8773137178985735, 12.53471296425189330 ) ) ;
#7891=CARTESIAN_POINT ( 'NONE',  ( -2.908627838312453306, 96.47731371789852517, 15.53471296425188797 ) ) ;
#7895=CARTESIAN_POINT ( 'NONE',  ( -12.46528703574805697, 114.1976862821014720, -2.660918448318280838 ) ) ;
#7896=CARTESIAN_POINT ( 'NONE',  ( 0.1745138560725837118, 61.01018628210145067, -15.50000000000000533 ) ) ;
#7899=CARTESIAN_POINT ( 'NONE',  ( -11.08355503943142573, 94.36018628210146630, 10.83675517735155402 ) ) ;
#7903=CARTESIAN_POINT ( 'NONE',  ( 3.796722387233379514, 15.58518628210145351, -8.710071997420127943 ) ) ;
#7907=CARTESIAN_POINT ( 'NONE',  ( -12.53471296425194836, 58.42268628210145209, 2.311890736173176641 ) ) ;
#7910=CARTESIAN_POINT ( 'NONE',  ( 8.710071997420127943, 27.08518628210144996, 3.796722387233375073 ) ) ;
#7921=CARTESIAN_POINT ( 'NONE',  ( 12.50000000000000355, 93.88981371789856212, -0.1745138560722771515 ) ) ;
#7922=CARTESIAN_POINT ( 'NONE',  ( 12.53471296425194659, 81.42268628210145209, -2.311890736173178418 ) ) ;
#7927=CARTESIAN_POINT ( 'NONE',  ( 3.257655550456945548, 49.90231371789854364, 15.46528703574811736 ) ) ;
#7932=CARTESIAN_POINT ( 'NONE',  ( -1.715153634034442431, 41.27731371789855075, 9.534712964251900402 ) ) ;
#7934=CARTESIAN_POINT ( 'NONE',  ( 6.840914352311949109, 85.83981371789856496, 6.594114490232462877 ) ) ;
#7936=CARTESIAN_POINT ( 'NONE',  ( -8.962234695871565293, 16.83981371789855430, -8.715434833792128799 ) ) ;
#7937=CARTESIAN_POINT ( 'NONE',  ( -0.1745138560725500443, 56.41018628210145636, 12.50000000000000355 ) ) ;
#7945=CARTESIAN_POINT ( 'NONE',  ( 9.465287035748067623, 72.79768628210145209, 2.064181346179272847 ) ) ;
#7947=CARTESIAN_POINT ( 'NONE',  ( -7.228626920339069173, 121.6726862821014521, 10.49813415415989581 ) ) ;
#7961=CARTESIAN_POINT ( 'NONE',  ( -11.61527771782809282, 135.8648137178985849, -4.622313124798832717 ) ) ;
#7962=CARTESIAN_POINT ( 'NONE',  ( 7.228626920339069173, 135.4726862821014493, -10.49813415415989404 ) ) ;
#7968=CARTESIAN_POINT ( 'NONE',  ( -13.04141134922778456, 116.0273137178985792, 8.927990412390377273 ) ) ;
#7974=CARTESIAN_POINT ( 'NONE',  ( 0.1745138560725515708, 107.0101862821014578, -12.50000000000000355 ) ) ;
#7981=CARTESIAN_POINT ( 'NONE',  ( 12.46528703574805874, 127.9976862821014407, 2.660918448318279950 ) ) ;
#7986=CARTESIAN_POINT ( 'NONE',  ( -14.38691631536207183, 122.5351862821014493, 5.770363421893814682 ) ) ;
#7988=CARTESIAN_POINT ( 'NONE',  ( 2.311890736173175753, 10.12268628210144428, 12.53471296425194836 ) ) ;
#7993=CARTESIAN_POINT ( 'NONE',  ( -6.840914352312096547, 75.96018628210144641, 6.594114490232313663 ) ) ;
#8001=CARTESIAN_POINT ( 'NONE',  ( -3.474262827703527901, 50.76481371789856212, 8.843639120294245259 ) ) ;
#8005=CARTESIAN_POINT ( 'NONE',  ( -11.48171059495408208, 61.11481371789854933, 4.944772684328421875 ) ) ;
#8008=CARTESIAN_POINT ( 'NONE',  ( 10.49813415416005213, 28.62731371789854506, -7.228626920338837358 ) ) ;
#8018=CARTESIAN_POINT ( 'NONE',  ( 11.61527771782809637, 76.06481371789855928, 4.622313124798827388 ) ) ;
#8024=CARTESIAN_POINT ( 'NONE',  ( 11.08355503943118769, 39.83981371789855075, 10.83675517735179028 ) ) ;
#8027=CARTESIAN_POINT ( 'NONE',  ( 6.932735513423970097, 9.547686282101453870, 10.69584247140445044 ) ) ;
#8028=CARTESIAN_POINT ( 'NONE',  ( -12.50000000000000355, 58.71018628210145351, -0.1745138560725492671 ) ) ;
#8029=CARTESIAN_POINT ( 'NONE',  ( -15.50000000000000533, 3.510186282101451560, -0.1745138560725808530 ) ) ;
#8034=CARTESIAN_POINT ( 'NONE',  ( 6.092822981423978490, 24.78518628210144215, -14.25334919248782306 ) ) ;
#8040=CARTESIAN_POINT ( 'NONE',  ( 7.228626920339068285, 6.672686282101436106, -10.49813415415989581 ) ) ;
#8042=CARTESIAN_POINT ( 'NONE',  ( -8.152565276336593669, 108.5523137178985422, -5.233372021372610483 ) ) ;
#8049=CARTESIAN_POINT ( 'NONE',  ( -11.48171059495408208, 125.5148137178985763, 4.944772684328421875 ) ) ;
#8063=CARTESIAN_POINT ( 'NONE',  ( 2.311890736173175753, 56.12268628210144072, 12.53471296425194836 ) ) ;
#8071=CARTESIAN_POINT ( 'NONE',  ( -8.715434833792127023, 124.9398137178985593, 8.962234695871568846 ) ) ;
#8077=CARTESIAN_POINT ( 'NONE',  ( -8.927990412390371944, 90.72731371789855359, -13.04141134922778988 ) ) ;
#8081=CARTESIAN_POINT ( 'NONE',  ( 11.48171059495397728, 119.0851862821014606, 4.944772684328674117 ) ) ;
#8082=CARTESIAN_POINT ( 'NONE',  ( -13.23911966647218463, 57.84768628210144925, 8.632099005475506459 ) ) ;
#8086=CARTESIAN_POINT ( 'NONE',  ( 6.092822981423978490, 89.18518628210145494, -14.25334919248782306 ) ) ;
#8090=CARTESIAN_POINT ( 'NONE',  ( -6.840914352312096547, 20.76018628210144001, 6.594114490232313663 ) ) ;
#8095=CARTESIAN_POINT ( 'NONE',  ( -4.622313124798576922, 60.43518628210145494, -11.61527771782819762 ) ) ;
#8098=CARTESIAN_POINT ( 'NONE',  ( 2.064181346179272847, 33.69768628210143646, -9.465287035748065847 ) ) ;
#8110=CARTESIAN_POINT ( 'NONE',  ( 12.46528703574805874, 91.19768628210145778, 2.660918448318279950 ) ) ;
#8116=CARTESIAN_POINT ( 'NONE',  ( 15.53471296425188797, 66.57731371789853370, 2.908627838312457747 ) ) ;
#8119=APPLICATION_CONTEXT ( 'automotive_design' ) ;
#8123=CARTESIAN_POINT ( 'NONE',  ( -6.840914352311947333, 44.43981371789855928, -6.594114490232462877 ) ) ;
#8125=CARTESIAN_POINT ( 'NONE',  ( 8.152565276336593669, 85.55231371789855643, 5.233372021372610483 ) ) ;
#8127=CARTESIAN_POINT ( 'NONE',  ( -13.04141134922778456, 143.6273137178985451, 8.927990412390377273 ) ) ;
#8130=CARTESIAN_POINT ( 'NONE',  ( -10.49813415415989581, 68.77268628210146062, -7.228626920339068285 ) ) ;
#8138=CARTESIAN_POINT ( 'NONE',  ( -8.152565276336710909, 76.24768628210145494, 5.233372021372435512 ) ) ;
#8140=CARTESIAN_POINT ( 'NONE',  ( 12.46528703574805874, 118.7976862821014663, 2.660918448318279950 ) ) ;
#8152=CARTESIAN_POINT ( 'NONE',  ( 12.46528703574811558, 130.4023137178985792, -2.660918448318005503 ) ) ;
#8153=CARTESIAN_POINT ( 'NONE',  ( -12.50000000000000355, 141.5101862821014720, -0.1745138560725508214 ) ) ;
#8158=CARTESIAN_POINT ( 'NONE',  ( 10.69584247140429589, 11.95231371789853902, 6.932735513424201024 ) ) ;
#8160=CARTESIAN_POINT ( 'NONE',  ( 5.770363421894130873, 110.5648137178985593, -14.38691631536193860 ) ) ;
#8165=CARTESIAN_POINT ( 'NONE',  ( -11.48171059495397373, 105.2851862821014493, -4.944772684328680334 ) ) ;
#8171=CARTESIAN_POINT ( 'NONE',  ( -10.69584247140444866, 122.2476862821014549, 6.932735513423972762 ) ) ;
#8176=CARTESIAN_POINT ( 'NONE',  ( 0.1745138560725837118, 97.81018628210145494, -15.50000000000000533 ) ) ;
#8177=CARTESIAN_POINT ( 'NONE',  ( -11.48171059495397373, 13.28518628210142971, -4.944772684328680334 ) ) ;
#8179=CARTESIAN_POINT ( 'NONE',  ( -0.1745138560725182642, 130.0101862821014436, 9.500000000000005329 ) ) ;
#8182=ORIENTED_EDGE ( 'NONE', *, *, #23582, .F. ) ;
#8184=CARTESIAN_POINT ( 'NONE',  ( 8.843639120294328748, 62.73518628210145920, -3.474262827703334722 ) ) ;
#8191=CARTESIAN_POINT ( 'NONE',  ( -2.064181346179062349, 54.50231371789855928, -9.465287035748106703 ) ) ;
#8195=CARTESIAN_POINT ( 'NONE',  ( 11.61527771782809637, 66.86481371789855643, 4.622313124798827388 ) ) ;
#8198=CARTESIAN_POINT ( 'NONE',  ( -6.932735513424201912, 23.45231371789854791, 10.69584247140429412 ) ) ;
#8214=CARTESIAN_POINT ( 'NONE',  ( -15.53471296425188442, 34.37731371789854506, -2.908627838312459080 ) ) ;
#8216=CARTESIAN_POINT ( 'NONE',  ( -8.715434833791929847, 4.660186282101435928, -8.962234695871762469 ) ) ;
#8217=CARTESIAN_POINT ( 'NONE',  ( -11.48171059495397373, 50.08518628210144641, -4.944772684328680334 ) ) ;
#8218=CARTESIAN_POINT ( 'NONE',  ( -11.08355503943142573, 11.56018628210145316, 10.83675517735155402 ) ) ;
#8222=CARTESIAN_POINT ( 'NONE',  ( -13.23911966647218463, 11.84768628210144747, 8.632099005475506459 ) ) ;
#8231=CARTESIAN_POINT ( 'NONE',  ( 5.529263428287300108, 104.5273137178985650, 7.954856959092309943 ) ) ;
#8238=CARTESIAN_POINT ( 'NONE',  ( 2.660918448318003282, 123.5023137178985593, 12.46528703574811558 ) ) ;
#8251=CARTESIAN_POINT ( 'NONE',  ( 0.1745138560725515708, 51.81018628210144783, -12.50000000000000355 ) ) ;
#8257=CARTESIAN_POINT ( 'NONE',  ( -0.1745138560722763466, 128.3898137178985621, -12.50000000000000355 ) ) ;
#8263=CARTESIAN_POINT ( 'NONE',  ( 5.770363421894130873, 92.16481371789855359, -14.38691631536193860 ) ) ;
#8266=CARTESIAN_POINT ( 'NONE',  ( -4.622313124798576922, 115.6351862821014578, -11.61527771782819762 ) ) ;
#8267=CARTESIAN_POINT ( 'NONE',  ( 5.770363421893814682, 55.83518628210145351, 14.38691631536207183 ) ) ;
#8270=CARTESIAN_POINT ( 'NONE',  ( -15.46528703574804986, 77.39768628210144641, -3.257655550457287497 ) ) ;
#8273=CARTESIAN_POINT ( 'NONE',  ( -2.064181346179269738, 19.89768628210143930, 9.465287035748067623 ) ) ;
#8277=CARTESIAN_POINT ( 'NONE',  ( -10.69584247140444866, 57.84768628210144925, 6.932735513423972762 ) ) ;
#8280=CARTESIAN_POINT ( 'NONE',  ( -9.500000000000005329, 31.11018628210143433, -0.1745138560725176813 ) ) ;
#8292=CARTESIAN_POINT ( 'NONE',  ( 11.48171059495397728, 63.88518628210145067, 4.944772684328674117 ) ) ;
#8297=CARTESIAN_POINT ( 'NONE',  ( 10.83675517735179206, 46.73981371789855643, -11.08355503943118769 ) ) ;
#8305=CARTESIAN_POINT ( 'NONE',  ( 0.1745138560723095977, 31.78981371789855004, 9.500000000000005329 ) ) ;
#8308=CARTESIAN_POINT ( 'NONE',  ( -3.474262827703527901, 96.76481371789854791, 8.843639120294245259 ) ) ;
#8310=CARTESIAN_POINT ( 'NONE',  ( 2.660918448318002838, 13.10231371789855004, 12.46528703574811558 ) ) ;
#8312=CARTESIAN_POINT ( 'NONE',  ( 2.311890736173175753, 65.32268628210144357, 12.53471296425194836 ) ) ;
#8319=CARTESIAN_POINT ( 'NONE',  ( -1.715153634034234598, 79.12268628210145494, -9.534712964251941258 ) ) ;
#8323=CARTESIAN_POINT ( 'NONE',  ( -7.228626920339069173, 112.4726862821014493, 10.49813415415989581 ) ) ;
#8336=CARTESIAN_POINT ( 'NONE',  ( 12.50000000000000355, 121.4898137178985564, -0.1745138560722771515 ) ) ;
#8337=CARTESIAN_POINT ( 'NONE',  ( 11.48171059495397728, 128.2851862821014493, 4.944772684328674117 ) ) ;
#8342=CARTESIAN_POINT ( 'NONE',  ( 8.632099005475788900, 101.6523137178985792, -13.23911966647199812 ) ) ;
#8343=CARTESIAN_POINT ( 'NONE',  ( -2.311890736173176641, 97.52268628210144641, -12.53471296425194836 ) ) ;
#8347=CARTESIAN_POINT ( 'NONE',  ( 4.622313124798573369, 120.2351862821014663, 11.61527771782819940 ) ) ;
#8353=CARTESIAN_POINT ( 'NONE',  ( 2.660918448318279950, 116.4976862821014549, -12.46528703574805697 ) ) ;
#8360=CARTESIAN_POINT ( 'NONE',  ( 3.257655550457285720, 107.2976862821014521, -15.46528703574804986 ) ) ;
#8361=CARTESIAN_POINT ( 'NONE',  ( 11.48171059495397728, 8.685186282101437172, 4.944772684328674117 ) ) ;
#8363=CARTESIAN_POINT ( 'NONE',  ( -9.500000000000005329, 123.1101862821014663, -0.1745138560725176813 ) ) ;
#8368=CARTESIAN_POINT ( 'NONE',  ( -9.500000000000005329, 58.71018628210145351, -0.1745138560725176813 ) ) ;
#8374=CARTESIAN_POINT ( 'NONE',  ( 0.1745138560723095977, 31.78981371789855004, 9.500000000000005329 ) ) ;
#8379=CARTESIAN_POINT ( 'NONE',  ( 8.962234695871567070, 58.23981371789854933, 8.715434833792127023 ) ) ;
#8382=CARTESIAN_POINT ( 'NONE',  ( -12.50000000000000355, 6.489813717898557321, 0.1745138560722786503 ) ) ;
#8386=CARTESIAN_POINT ( 'NONE',  ( 2.660918448318279950, 6.097686282101443922, -12.46528703574805697 ) ) ;
#8399=CARTESIAN_POINT ( 'NONE',  ( -3.257655550456946880, 17.70231371789854435, -15.46528703574811736 ) ) ;
#8401=CARTESIAN_POINT ( 'NONE',  ( -2.311890736173176641, 5.522686282101451738, -12.53471296425194836 ) ) ;
#8402=CARTESIAN_POINT ( 'NONE',  ( -10.69584247140444866, 48.64768628210144641, 6.932735513423972762 ) ) ;
#8406=CARTESIAN_POINT ( 'NONE',  ( -11.08355503943142573, 20.76018628210144001, 10.83675517735155402 ) ) ;
#8413=CARTESIAN_POINT ( 'NONE',  ( -0.1745138560723084320, 100.7898137178985536, -9.500000000000005329 ) ) ;
#8419=CARTESIAN_POINT ( 'NONE',  ( 8.962234695871567070, 113.4398137178985593, 8.715434833792127023 ) ) ;
#8432=CARTESIAN_POINT ( 'NONE',  ( 8.962234695871762469, 52.96018628210144641, -8.715434833791931624 ) ) ;
#8437=CARTESIAN_POINT ( 'NONE',  ( -12.46528703574811558, 107.4023137178985650, 2.660918448318003726 ) ) ;
#8443=CARTESIAN_POINT ( 'NONE',  ( 3.257655550456945548, 68.30231371789852801, 15.46528703574811736 ) ) ;
#8447=CARTESIAN_POINT ( 'NONE',  ( 0.1745138560725515708, 97.81018628210144072, -12.50000000000000355 ) ) ;
#8448=CARTESIAN_POINT ( 'NONE',  ( 11.08355503943142750, 71.36018628210143788, -10.83675517735155225 ) ) ;
#8452=CARTESIAN_POINT ( 'NONE',  ( 3.257655550457285720, 61.29768628210142367, -15.46528703574804986 ) ) ;
#8457=CARTESIAN_POINT ( 'NONE',  ( 11.48171059495397728, 36.28518628210144925, 4.944772684328674117 ) ) ;
#8460=CARTESIAN_POINT ( 'NONE',  ( -8.710071997420127943, 31.68518628210144428, -3.796722387233380402 ) ) ;
#8470=CARTESIAN_POINT ( 'NONE',  ( 10.69584247140445221, 62.44768628210145778, -6.932735513423970097 ) ) ;
#8478=CARTESIAN_POINT ( 'NONE',  ( -15.50000000000000533, 43.28981371789856070, 0.1745138560722471477 ) ) ;
#8484=CARTESIAN_POINT ( 'NONE',  ( -1.715153634034442431, 13.67731371789853867, 9.534712964251900402 ) ) ;
#8491=CARTESIAN_POINT ( 'NONE',  ( 8.962234695871567070, 12.23981371789853512, 8.715434833792127023 ) ) ;
#8494=CARTESIAN_POINT ( 'NONE',  ( 7.228626920339068285, 71.07268628210144357, -10.49813415415989581 ) ) ;
#8503=CARTESIAN_POINT ( 'NONE',  ( -8.843639120294326972, 76.53518628210146346, 3.474262827703335166 ) ) ;
#8506=CARTESIAN_POINT ( 'NONE',  ( -0.1745138560725500443, 120.8101862821014691, 12.50000000000000355 ) ) ;
#8517=CARTESIAN_POINT ( 'NONE',  ( -11.48171059495408208, 116.3148137178985593, 4.944772684328421875 ) ) ;
#8518=CARTESIAN_POINT ( 'NONE',  ( 8.962234695871762469, 126.5601862821014691, -8.715434833791931624 ) ) ;
#8525=CARTESIAN_POINT ( 'NONE',  ( 6.092822981423662299, 95.61481371789857064, 14.25334919248795096 ) ) ;
#8526=CARTESIAN_POINT ( 'NONE',  ( 6.932735513423970097, 101.5476862821014379, 10.69584247140445044 ) ) ;
#8529=CARTESIAN_POINT ( 'NONE',  ( 9.534712964251900402, 75.77731371789855075, 1.715153634034445540 ) ) ;
#8533=CARTESIAN_POINT ( 'NONE',  ( 7.228626920339068285, 126.2726862821014606, -10.49813415415989581 ) ) ;
#8539=CARTESIAN_POINT ( 'NONE',  ( 2.908627838312118019, 102.1226862821014549, 15.53471296425195369 ) ) ;
#8540=CARTESIAN_POINT ( 'NONE',  ( -2.660918448318275509, 19.89768628210143575, 12.46528703574805874 ) ) ;
#8543=CARTESIAN_POINT ( 'NONE',  ( -1.715153634034234598, 134.3226862821014436, -9.534712964251941258 ) ) ;
#8547=CARTESIAN_POINT ( 'NONE',  ( 8.152565276336714462, 71.64768628210146062, -5.233372021372432847 ) ) ;
#8554=CARTESIAN_POINT ( 'NONE',  ( 8.843639120294245259, 30.06481371789855572, 3.474262827703527901 ) ) ;
#8560=CARTESIAN_POINT ( 'NONE',  ( 7.228626920338837358, 40.12731371789853796, 10.49813415416005036 ) ) ;
#8563=CARTESIAN_POINT ( 'NONE',  ( 6.092822981423662299, 141.6148137178985849, 14.25334919248795096 ) ) ;
#8578=CARTESIAN_POINT ( 'NONE',  ( 11.08355503943118769, 21.43981371789854506, 10.83675517735179028 ) ) ;
#8580=CARTESIAN_POINT ( 'NONE',  ( 12.53471296425194836, 17.02268628210144996, -2.311890736173178418 ) ) ;
#8581=CARTESIAN_POINT ( 'NONE',  ( -7.228626920339069173, 48.07268628210143646, 10.49813415415989581 ) ) ;
#8592=CARTESIAN_POINT ( 'NONE',  ( 5.233372021372610483, 101.6523137178985792, -8.152565276336593669 ) ) ;
#8599=CARTESIAN_POINT ( 'NONE',  ( -8.715434833792127023, 106.5398137178985536, 8.962234695871568846 ) ) ;
#8604=CARTESIAN_POINT ( 'NONE',  ( 11.48171059495408208, 65.71481371789855075, -4.944772684328420986 ) ) ;
#8613=CARTESIAN_POINT ( 'NONE',  ( 11.61527771782819940, 62.73518628210145209, -4.622313124798573369 ) ) ;
#8620=CARTESIAN_POINT ( 'NONE',  ( -0.1745138560722763466, 100.7898137178985536, -12.50000000000000355 ) ) ;
#8626=CARTESIAN_POINT ( 'NONE',  ( -6.092822981423666739, 81.81481371789855928, -14.25334919248795096 ) ) ;
#8630=CARTESIAN_POINT ( 'NONE',  ( 6.932735513423970097, 101.5476862821014379, 10.69584247140445044 ) ) ;
#8632=CARTESIAN_POINT ( 'NONE',  ( 13.23911966647218996, 44.04768628210143788, -8.632099005475504683 ) ) ;
#8635=CARTESIAN_POINT ( 'NONE',  ( 2.908627838312118019, 74.52268628210144641, 15.53471296425195369 ) ) ;
#8640=CARTESIAN_POINT ( 'NONE',  ( -6.932735513423968321, 41.74768628210144783, -10.69584247140445221 ) ) ;
#8643=CARTESIAN_POINT ( 'NONE',  ( -1.715153634034234598, 5.522686282101450850, -9.534712964251941258 ) ) ;
#8654=CARTESIAN_POINT ( 'NONE',  ( 11.61527771782819940, 71.93518628210145494, -4.622313124798573369 ) ) ;
#8661=CARTESIAN_POINT ( 'NONE',  ( 15.50000000000000533, 47.88981371789855501, -0.1745138560722452326 ) ) ;
#8668=CARTESIAN_POINT ( 'NONE',  ( 7.954856959092311719, 19.42731371789854933, -5.529263428287300108 ) ) ;
#8673=CARTESIAN_POINT ( 'NONE',  ( 13.04141134922778988, 139.0273137178985507, -8.927990412390371944 ) ) ;
#8676=CARTESIAN_POINT ( 'NONE',  ( -12.46528703574805697, 40.59768628210144215, -2.660918448318280838 ) ) ;
#8683=CARTESIAN_POINT ( 'NONE',  ( 9.534712964251941258, 72.22268628210143504, -1.715153634034235708 ) ) ;
#8686=CARTESIAN_POINT ( 'NONE',  ( 4.944772684328679446, 98.38518628210145778, -11.48171059495397373 ) ) ;
#8698=CARTESIAN_POINT ( 'NONE',  ( 7.228626920338837358, 122.9273137178985422, 10.49813415416005036 ) ) ;
#8700=CARTESIAN_POINT ( 'NONE',  ( 0.1745138560725515708, 125.4101862821014635, -12.50000000000000355 ) ) ;
#8707=CARTESIAN_POINT ( 'NONE',  ( 2.908627838312458636, 91.87731371789854506, -15.53471296425188442 ) ) ;
#8712=CARTESIAN_POINT ( 'NONE',  ( -9.465287035748106703, 79.80231371789852801, 2.064181346179061460 ) ) ;
#8716=CARTESIAN_POINT ( 'NONE',  ( 2.311890736173452865, 55.07731371789855501, -12.53471296425189152 ) ) ;
#8718=CARTESIAN_POINT ( 'NONE',  ( -12.50000000000000355, 95.51018628210144357, -0.1745138560725492671 ) ) ;
#8723=CARTESIAN_POINT ( 'NONE',  ( 10.83675517735155225, 110.4601862821014606, 11.08355503943142573 ) ) ;
#8724=CARTESIAN_POINT ( 'NONE',  ( 2.660918448318279950, 15.29768628210143078, -12.46528703574805874 ) ) ;
#8727=CARTESIAN_POINT ( 'NONE',  ( -8.843639120294326972, 131.7351862821014663, 3.474262827703335166 ) ) ;
#8733=CARTESIAN_POINT ( 'NONE',  ( 8.152565276336714462, 62.44768628210144357, -5.233372021372432847 ) ) ;
#8742=CARTESIAN_POINT ( 'NONE',  ( -6.840914352311947333, 44.43981371789855928, -6.594114490232462877 ) ) ;
#8747=CARTESIAN_POINT ( 'NONE',  ( 4.622313124798831829, 36.96481371789854364, -11.61527771782809282 ) ) ;
#8750=CARTESIAN_POINT ( 'NONE',  ( 11.61527771782809637, 11.66481371789854293, 4.622313124798827388 ) ) ;
#8757=( LENGTH_UNIT ( ) NAMED_UNIT ( * ) SI_UNIT ( .MILLI., .METRE. ) );
#8765=CARTESIAN_POINT ( 'NONE',  ( -15.46528703574811736, 24.60231371789854649, 3.257655550456946436 ) ) ;
#8767=CARTESIAN_POINT ( 'NONE',  ( -8.843639120294326972, 140.9351862821014549, 3.474262827703335166 ) ) ;
#8769=CARTESIAN_POINT ( 'NONE',  ( -6.932735513423968321, 50.94768628210144357, -10.69584247140445221 ) ) ;
#8782=CARTESIAN_POINT ( 'NONE',  ( -9.534712964251895073, 98.77731371789855075, -1.715153634034446428 ) ) ;
#8789=CARTESIAN_POINT ( 'NONE',  ( -12.53471296425189152, 98.77731371789855075, -2.311890736173453309 ) ) ;
#8793=CARTESIAN_POINT ( 'NONE',  ( 2.660918448318002838, 68.30231371789854222, 12.46528703574811558 ) ) ;
#8802=CARTESIAN_POINT ( 'NONE',  ( 12.46528703574805874, 45.19768628210143646, 2.660918448318279950 ) ) ;
#8808=CARTESIAN_POINT ( 'NONE',  ( 2.660918448318002838, 95.90231371789856496, 12.46528703574811558 ) ) ;
#8812=CARTESIAN_POINT ( 'NONE',  ( 15.50000000000000533, 84.68981371789855928, -0.1745138560722452326 ) ) ;
#8816=CARTESIAN_POINT ( 'NONE',  ( -10.69584247140444866, 113.0476862821014663, 6.932735513423972762 ) ) ;
#8817=CARTESIAN_POINT ( 'NONE',  ( 2.908627838312118019, 37.72268628210143504, 15.53471296425195369 ) ) ;
#8821=CARTESIAN_POINT ( 'NONE',  ( -15.46528703574804986, 68.19768628210142936, -3.257655550457287497 ) ) ;
#8828=CARTESIAN_POINT ( 'NONE',  ( -2.660918448318275509, 38.29768628210145920, 12.46528703574805874 ) ) ;
#8831=CARTESIAN_POINT ( 'NONE',  ( -6.594114490232312775, 13.86018628210145032, -6.840914352312096547 ) ) ;
#8841=CARTESIAN_POINT ( 'NONE',  ( -4.944772684328673229, 66.18518628210144072, 11.48171059495397728 ) ) ;
#8848=CARTESIAN_POINT ( 'NONE',  ( -6.092822981423666739, 45.01481371789854791, -14.25334919248795096 ) ) ;
#8854=CARTESIAN_POINT ( 'NONE',  ( 2.064181346179061460, 22.30231371789854933, 9.465287035748106703 ) ) ;
#8859=CARTESIAN_POINT ( 'NONE',  ( 5.770363421894130873, 138.1648137178985678, -14.38691631536193860 ) ) ;
#8861=CARTESIAN_POINT ( 'NONE',  ( -12.50000000000000355, 40.31018628210144783, -0.1745138560725492671 ) ) ;
#8868=CARTESIAN_POINT ( 'NONE',  ( -9.500000000000005329, 58.71018628210145351, -0.1745138560725176813 ) ) ;
#8871=CARTESIAN_POINT ( 'NONE',  ( 2.311890736173175753, 102.1226862821014691, 12.53471296425194836 ) ) ;
#8882=CARTESIAN_POINT ( 'NONE',  ( -6.932735513424201912, 115.4523137178985621, 10.69584247140429412 ) ) ;
#8883=CARTESIAN_POINT ( 'NONE',  ( 12.50000000000000355, 118.5101862821014578, 0.1745138560725507937 ) ) ;
#8889=CARTESIAN_POINT ( 'NONE',  ( -14.38691631536193860, 99.06481371789857349, -5.770363421894132649 ) ) ;
#8894=CARTESIAN_POINT ( 'NONE',  ( -3.474262827703527901, 69.16481371789853938, 8.843639120294245259 ) ) ;
#8898=CARTESIAN_POINT ( 'NONE',  ( -2.311890736173448424, 41.27731371789855075, 12.53471296425189330 ) ) ;
#8900=CARTESIAN_POINT ( 'NONE',  ( 10.69584247140445221, 108.4476862821014578, -6.932735513423970097 ) ) ;
#8904=CARTESIAN_POINT ( 'NONE',  ( 11.61527771782819940, 136.3351862821014606, -4.622313124798573369 ) ) ;
#8906=CARTESIAN_POINT ( 'NONE',  ( -14.25334919248782306, 96.08518628210146062, -6.092822981423979378 ) ) ;
#8909=CARTESIAN_POINT ( 'NONE',  ( -12.53471296425194659, 12.42268628210144144, 2.311890736173176641 ) ) ;
#8912=CARTESIAN_POINT ( 'NONE',  ( 2.064181346179272847, 125.6976862821014578, -9.465287035748065847 ) ) ;
#8918=CARTESIAN_POINT ( 'NONE',  ( 9.500000000000005329, 54.11018628210144499, 0.1745138560725188748 ) ) ;
#8925=CARTESIAN_POINT ( 'NONE',  ( 3.796722387233182339, 40.41481371789855359, 8.710071997420207879 ) ) ;
#8930=CARTESIAN_POINT ( 'NONE',  ( -8.715434833792127023, 42.13981371789854791, 8.962234695871568846 ) ) ;
#8933=CARTESIAN_POINT ( 'NONE',  ( -11.61527771782809282, 16.26481371789853370, -4.622313124798832717 ) ) ;
#8953=CARTESIAN_POINT ( 'NONE',  ( 8.927990412390371944, 21.72731371789853938, 13.04141134922778811 ) ) ;
#8956=CARTESIAN_POINT ( 'NONE',  ( 6.594114490232313663, 138.0601862821014549, 6.840914352312096547 ) ) ;
#8957=CARTESIAN_POINT ( 'NONE',  ( 8.962234695871762469, 43.76018628210144357, -8.715434833791931624 ) ) ;
#8961=CARTESIAN_POINT ( 'NONE',  ( 5.233372021372432847, 27.94768628210144001, 8.152565276336710909 ) ) ;
#8968=CARTESIAN_POINT ( 'NONE',  ( -9.534712964251895073, 89.57731371789856212, -1.715153634034446428 ) ) ;
#8974=CARTESIAN_POINT ( 'NONE',  ( 0.1745138560722779009, 105.3898137178985621, 12.50000000000000355 ) ) ;
#8978=CARTESIAN_POINT ( 'NONE',  ( 6.932735513424201024, 74.05231371789855643, -10.69584247140429412 ) ) ;
#8985=CARTESIAN_POINT ( 'NONE',  ( -11.61527771782819940, 39.73518628210144499, 4.622313124798574258 ) ) ;
#8993=CARTESIAN_POINT ( 'NONE',  ( 0.1745138560722779009, 105.3898137178985621, 12.50000000000000355 ) ) ;
#8998=CARTESIAN_POINT ( 'NONE',  ( -15.53471296425188442, 80.37731371789853085, -2.908627838312459080 ) ) ;
#9002=CARTESIAN_POINT ( 'NONE',  ( 4.622313124798573369, 101.8351862821014464, 11.61527771782819940 ) ) ;
#9003=CARTESIAN_POINT ( 'NONE',  ( -15.46528703574804986, 49.79768628210144499, -3.257655550457287497 ) ) ;
#9006=CARTESIAN_POINT ( 'NONE',  ( 2.908627838312118019, 65.32268628210144357, 15.53471296425195369 ) ) ;
#9012=CARTESIAN_POINT ( 'NONE',  ( -10.69584247140444866, 39.44768628210145067, 6.932735513423972762 ) ) ;
#9015=CARTESIAN_POINT ( 'NONE',  ( 6.840914352312096547, 6.960186282101432198, -6.594114490232313663 ) ) ;
#9026=CARTESIAN_POINT ( 'NONE',  ( -7.228626920339070061, 66.47268628210144925, 10.49813415415989404 ) ) ;
#9034=CARTESIAN_POINT ( 'NONE',  ( -15.46528703574811736, 24.60231371789854649, 3.257655550456946436 ) ) ;
#9041=CARTESIAN_POINT ( 'NONE',  ( 3.474262827703532341, 27.76481371789854791, -8.843639120294245259 ) ) ;
#9047=CARTESIAN_POINT ( 'NONE',  ( 13.23911966647199812, 131.5523137178985564, 8.632099005475788900 ) ) ;
#9051=CARTESIAN_POINT ( 'NONE',  ( -12.50000000000000355, 49.51018628210145067, -0.1745138560725492671 ) ) ;
#9059=CARTESIAN_POINT ( 'NONE',  ( -0.1745138560725182642, 65.61018628210146630, 9.500000000000005329 ) ) ;
#9062=CARTESIAN_POINT ( 'NONE',  ( 0.1745138560725515708, 88.61018628210146630, -12.50000000000000355 ) ) ;
#9075=CARTESIAN_POINT ( 'NONE',  ( -12.53471296425189152, 107.9773137178985536, -2.311890736173453753 ) ) ;
#9076=CARTESIAN_POINT ( 'NONE',  ( 11.61527771782819940, 127.1351862821014578, -4.622313124798573369 ) ) ;
#9081=CARTESIAN_POINT ( 'NONE',  ( 13.23911966647199812, 85.55231371789855643, 8.632099005475788900 ) ) ;
#9085=CARTESIAN_POINT ( 'NONE',  ( 3.474262827703335166, 101.8351862821014606, 8.843639120294326972 ) ) ;
#9087=CARTESIAN_POINT ( 'NONE',  ( -8.710071997420207879, 70.31481371789853085, 3.796722387233182339 ) ) ;
#9090=CARTESIAN_POINT ( 'NONE',  ( 12.50000000000000355, 57.08981371789855075, -0.1745138560722771515 ) ) ;
#9093=CARTESIAN_POINT ( 'NONE',  ( 4.622313124798573369, 101.8351862821014464, 11.61527771782819940 ) ) ;
#9096=CARTESIAN_POINT ( 'NONE',  ( -0.1745138560725500443, 139.2101862821014606, 12.50000000000000355 ) ) ;
#9098=CARTESIAN_POINT ( 'NONE',  ( -14.25334919248782306, 86.88518628210145778, -6.092822981423979378 ) ) ;
#9101=CARTESIAN_POINT ( 'NONE',  ( -3.474262827703337830, 115.6351862821014436, -8.843639120294326972 ) ) ;
#9104=CARTESIAN_POINT ( 'NONE',  ( -8.927990412390661490, 20.47268628210143859, 13.04141134922759804 ) ) ;
#9110=CARTESIAN_POINT ( 'NONE',  ( -6.840914352312096547, 48.36018628210145209, 6.594114490232313663 ) ) ;
#9114=DIRECTION ( 'NONE',  ( 1.047113545471812582E-14, 0.1163425707149433608, -0.9932091452657082487 ) ) ;
#9118=CARTESIAN_POINT ( 'NONE',  ( 5.529263428287300108, 40.12731371789853796, 7.954856959092309943 ) ) ;
#9122=CARTESIAN_POINT ( 'NONE',  ( 11.61527771782809637, 48.46481371789855785, 4.622313124798827388 ) ) ;
#9124=CARTESIAN_POINT ( 'NONE',  ( -4.622313124798826500, 13.96481371789853831, 11.61527771782809637 ) ) ;
#9142=CARTESIAN_POINT ( 'NONE',  ( -2.908627838312453306, 22.87731371789854151, 15.53471296425188797 ) ) ;
#9144=CARTESIAN_POINT ( 'NONE',  ( -7.954856959092191815, 123.9726862821014493, -5.529263428287477744 ) ) ;
#9145=CARTESIAN_POINT ( 'NONE',  ( 2.311890736173175753, 37.72268628210144215, 12.53471296425194836 ) ) ;
#9150=CARTESIAN_POINT ( 'NONE',  ( -3.796722387233375073, 29.38518628210144712, 8.710071997420127943 ) ) ;
#9157=CARTESIAN_POINT ( 'NONE',  ( 6.840914352311949109, 85.83981371789856496, 6.594114490232462877 ) ) ;
#9162=CARTESIAN_POINT ( 'NONE',  ( -6.932735513424201912, 97.05231371789855643, 10.69584247140429412 ) ) ;
#9167=CARTESIAN_POINT ( 'NONE',  ( -11.61527771782809282, 62.26481371789854791, -4.622313124798832717 ) ) ;
#9175=CARTESIAN_POINT ( 'NONE',  ( -10.69584247140444866, 39.44768628210145067, 6.932735513423972762 ) ) ;
#9180=CARTESIAN_POINT ( 'NONE',  ( 12.46528703574811558, 93.60231371789855359, -2.660918448318005503 ) ) ;
#9186=CARTESIAN_POINT ( 'NONE',  ( -14.25334919248795096, 70.31481371789853085, 6.092822981423662299 ) ) ;
#9191=CARTESIAN_POINT ( 'NONE',  ( -4.944772684328673229, 102.9851862821014663, 11.48171059495397728 ) ) ;
#9192=CARTESIAN_POINT ( 'NONE',  ( 13.04141134922759804, 45.77268628210144641, 8.927990412390657937 ) ) ;
#9195=CARTESIAN_POINT ( 'NONE',  ( 15.46528703574804986, 54.39768628210144641, 3.257655550457285720 ) ) ;
#9202=CARTESIAN_POINT ( 'NONE',  ( 2.311890736173175753, 46.92268628210145209, 12.53471296425194836 ) ) ;
#9203=CARTESIAN_POINT ( 'NONE',  ( -9.500000000000005329, 3.510186282101451560, -0.1745138560725176813 ) ) ;
#9213=CARTESIAN_POINT ( 'NONE',  ( 7.228626920339069173, 52.67268628210145209, -10.49813415415989404 ) ) ;
#9220=CARTESIAN_POINT ( 'NONE',  ( 12.50000000000000355, 90.91018628210146346, 0.1745138560725507937 ) ) ;
#9221=CARTESIAN_POINT ( 'NONE',  ( 5.770363421894130873, 27.76481371789854791, -14.38691631536193860 ) ) ;
#9226=CARTESIAN_POINT ( 'NONE',  ( -6.840914352311947333, 26.03981371789855714, -6.594114490232462877 ) ) ;
#9232=CARTESIAN_POINT ( 'NONE',  ( -8.632099005475794229, 124.6523137178985650, 13.23911966647199812 ) ) ;
#9237=CARTESIAN_POINT ( 'NONE',  ( 12.50000000000000355, 54.11018628210144499, 0.1745138560725507937 ) ) ;
#9245=CARTESIAN_POINT ( 'NONE',  ( -3.474262827703337830, 60.43518628210146204, -8.843639120294326972 ) ) ;
#9249=CARTESIAN_POINT ( 'NONE',  ( -4.944772684328673229, 102.9851862821014663, 11.48171059495397728 ) ) ;
#9262=CARTESIAN_POINT ( 'NONE',  ( -12.53471296425189152, 98.77731371789855075, -2.311890736173453753 ) ) ;
#9263=CARTESIAN_POINT ( 'NONE',  ( -2.660918448318275509, 102.6976862821014578, 12.46528703574805874 ) ) ;
#9268=CARTESIAN_POINT ( 'NONE',  ( -6.092822981423666739, 81.81481371789855928, -14.25334919248795096 ) ) ;
#9272=CARTESIAN_POINT ( 'NONE',  ( -9.465287035748065847, 104.9976862821014549, -2.064181346179273735 ) ) ;
#9273=PRODUCT_DEFINITION_SHAPE ( 'NONE', 'NONE',  #18775 ) ;
#9275=CARTESIAN_POINT ( 'NONE',  ( 9.500000000000005329, 75.48981371789854222, -0.1745138560723090149 ) ) ;
#9279=CARTESIAN_POINT ( 'NONE',  ( 10.49813415416005213, 56.22731371789854649, -7.228626920338837358 ) ) ;
#9281=CARTESIAN_POINT ( 'NONE',  ( -12.50000000000000355, 104.7101862821014606, -0.1745138560725492671 ) ) ;
#9284=CARTESIAN_POINT ( 'NONE',  ( -12.53471296425194836, 141.2226862821014493, 2.311890736173176641 ) ) ;
#9286=CARTESIAN_POINT ( 'NONE',  ( 8.632099005475504683, 83.14768628210143220, 13.23911966647218996 ) ) ;
#9288=CARTESIAN_POINT ( 'NONE',  ( -11.48171059495397373, 4.085186282101443744, -4.944772684328680334 ) ) ;
#9291=CARTESIAN_POINT ( 'NONE',  ( -6.594114490232312775, 105.8601862821014379, -6.840914352312096547 ) ) ;
#9294=CARTESIAN_POINT ( 'NONE',  ( 14.38691631536207538, 16.73518628210143788, -5.770363421893813793 ) ) ;
#9306=CARTESIAN_POINT ( 'NONE',  ( 6.840914352311949109, 12.23981371789853512, 6.594114490232462877 ) ) ;
#9311=CARTESIAN_POINT ( 'NONE',  ( -12.50000000000000355, 43.28981371789855359, 0.1745138560722786503 ) ) ;
#9313=CARTESIAN_POINT ( 'NONE',  ( 14.38691631536194393, 122.0648137178985877, 5.770363421894124656 ) ) ;
#9329=CARTESIAN_POINT ( 'NONE',  ( 14.38691631536207538, 136.3351862821014606, -5.770363421893813793 ) ) ;
#9333=CARTESIAN_POINT ( 'NONE',  ( 8.152565276336714462, 136.0476862821014379, -5.233372021372432847 ) ) ;
#9336=CARTESIAN_POINT ( 'NONE',  ( 4.622313124798573369, 28.23518628210144854, 11.61527771782819940 ) ) ;
#9340=CARTESIAN_POINT ( 'NONE',  ( -8.927990412390661490, 121.6726862821014521, 13.04141134922759804 ) ) ;
#9342=CARTESIAN_POINT ( 'NONE',  ( -0.1745138560725182642, 10.41018628210144037, 9.500000000000005329 ) ) ;
#9348=CARTESIAN_POINT ( 'NONE',  ( 7.954856959092311719, 83.82731371789856212, -5.529263428287300108 ) ) ;
#9352=CARTESIAN_POINT ( 'NONE',  ( -7.228626920338836470, 90.72731371789855359, -10.49813415416005213 ) ) ;
#9356=CARTESIAN_POINT ( 'NONE',  ( 8.962234695871567070, 67.43981371789855928, 8.715434833792127023 ) ) ;
#9363=CARTESIAN_POINT ( 'NONE',  ( 0.1745138560725515708, 33.41018628210144925, -12.50000000000000355 ) ) ;
#9369=CARTESIAN_POINT ( 'NONE',  ( 8.715434833792128799, 83.53981371789856780, -8.962234695871567070 ) ) ;
#9375=CARTESIAN_POINT ( 'NONE',  ( 8.632099005475788900, 64.85231371789855359, -13.23911966647199812 ) ) ;
#9378=CARTESIAN_POINT ( 'NONE',  ( -6.932735513423968321, 78.54768628210146630, -10.69584247140445221 ) ) ;
#9379=CARTESIAN_POINT ( 'NONE',  ( -15.46528703574804986, 40.59768628210144215, -3.257655550457287497 ) ) ;
#9382=CARTESIAN_POINT ( 'NONE',  ( -13.23911966647218463, 48.64768628210144641, 8.632099005475506459 ) ) ;
#9390=CARTESIAN_POINT ( 'NONE',  ( 7.228626920339068285, 15.87268628210144961, -10.49813415415989581 ) ) ;
#9392=CARTESIAN_POINT ( 'NONE',  ( 3.796722387233182339, 141.6148137178985849, 8.710071997420207879 ) ) ;
#9402=CARTESIAN_POINT ( 'NONE',  ( -11.48171059495397373, 40.88518628210144357, -4.944772684328680334 ) ) ;
#9409=CARTESIAN_POINT ( 'NONE',  ( 11.61527771782819940, 90.33518628210144641, -4.622313124798573369 ) ) ;
#9410=CARTESIAN_POINT ( 'NONE',  ( -3.257655550456946880, 17.70231371789854435, -15.46528703574811736 ) ) ;
#9416=CARTESIAN_POINT ( 'NONE',  ( 4.944772684328420986, 141.6148137178985849, 11.48171059495408208 ) ) ;
#9423=CARTESIAN_POINT ( 'NONE',  ( 15.50000000000000533, 139.8898137178985621, -0.1745138560722452326 ) ) ;
#9426=CARTESIAN_POINT ( 'NONE',  ( -11.61527771782819940, 39.73518628210144499, 4.622313124798574258 ) ) ;
#9429=CARTESIAN_POINT ( 'NONE',  ( 0.1745138560725837118, 97.81018628210145494, -15.50000000000000533 ) ) ;
#9432=CARTESIAN_POINT ( 'NONE',  ( 8.710071997420127943, 54.68518628210145494, 3.796722387233375073 ) ) ;
#9435=CARTESIAN_POINT ( 'NONE',  ( -7.228626920339069173, 94.07268628210145778, 10.49813415415989581 ) ) ;
#9449=CARTESIAN_POINT ( 'NONE',  ( -2.660918448318004614, 109.7023137178985621, -12.46528703574811558 ) ) ;
#9450=CARTESIAN_POINT ( 'NONE',  ( 8.962234695871762469, 98.96018628210146062, -8.715434833791931624 ) ) ;
#9454=CARTESIAN_POINT ( 'NONE',  ( -2.908627838312453306, 68.87731371789855928, 15.53471296425188797 ) ) ;
#9457=CARTESIAN_POINT ( 'NONE',  ( -8.843639120294326972, 94.93518628210146915, 3.474262827703335166 ) ) ;
#9461=CARTESIAN_POINT ( 'NONE',  ( 3.796722387233182339, 58.81481371789855217, 8.710071997420207879 ) ) ;
#9464=CARTESIAN_POINT ( 'NONE',  ( -3.796722387233185003, 118.6148137178985706, -8.710071997420207879 ) ) ;
#9466=CARTESIAN_POINT ( 'NONE',  ( 4.622313124798831829, 46.16481371789854649, -11.61527771782809282 ) ) ;
#9468=CARTESIAN_POINT ( 'NONE',  ( 4.944772684328679446, 98.38518628210145778, -11.48171059495397373 ) ) ;
#9471=CARTESIAN_POINT ( 'NONE',  ( -4.944772684328673229, 139.7851862821014493, 11.48171059495397728 ) ) ;
#9473=CARTESIAN_POINT ( 'NONE',  ( -13.04141134922759804, 87.17268628210142367, -8.927990412390657937 ) ) ;
#9475=CARTESIAN_POINT ( 'NONE',  ( -10.49813415415989404, 4.372686282101439836, -7.228626920339069173 ) ) ;
#9478=CARTESIAN_POINT ( 'NONE',  ( -6.840914352312096547, 121.9601862821014606, 6.594114490232313663 ) ) ;
#9480=CARTESIAN_POINT ( 'NONE',  ( -5.770363421893818234, 5.235186282101429001, -14.38691631536207005 ) ) ;
#9492=CARTESIAN_POINT ( 'NONE',  ( 9.500000000000005329, 20.28981371789855004, -0.1745138560723090149 ) ) ;
#9497=CARTESIAN_POINT ( 'NONE',  ( 10.49813415416005213, 19.42731371789854933, -7.228626920338837358 ) ) ;
#9499=CARTESIAN_POINT ( 'NONE',  ( -13.04141134922778456, 134.4273137178984996, 8.927990412390377273 ) ) ;
#9520=CARTESIAN_POINT ( 'NONE',  ( -15.53471296425188442, 6.777313717898553413, -2.908627838312459080 ) ) ;
#9522=CARTESIAN_POINT ( 'NONE',  ( 8.152565276336714462, 126.8476862821014635, -5.233372021372432847 ) ) ;
#9524=CARTESIAN_POINT ( 'NONE',  ( -11.48171059495397373, 31.68518628210144428, -4.944772684328680334 ) ) ;
#9527=CARTESIAN_POINT ( 'NONE',  ( 14.25334919248782661, 119.0851862821014606, 6.092822981423971385 ) ) ;
#9529=CARTESIAN_POINT ( 'NONE',  ( -3.474262827703527901, 142.7648137178985621, 8.843639120294245259 ) ) ;
#9535=CARTESIAN_POINT ( 'NONE',  ( 2.064181346179061460, 68.30231371789852801, 9.465287035748106703 ) ) ;
#9540=CARTESIAN_POINT ( 'NONE',  ( -2.660918448318005058, 72.90231371789855075, -12.46528703574811558 ) ) ;
#9542=CARTESIAN_POINT ( 'NONE',  ( -12.65935014772596823, 143.0000000000000284, 5.795439718954652264 ) ) ;
#9544=CARTESIAN_POINT ( 'NONE',  ( -7.228626920338836470, 53.92731371789854933, -10.49813415416005213 ) ) ;
#9550=CARTESIAN_POINT ( 'NONE',  ( -12.53471296425194836, 49.22268628210144215, 2.311890736173176641 ) ) ;
#9555=CARTESIAN_POINT ( 'NONE',  ( -8.962234695871565293, 81.23981371789855643, -8.715434833792128799 ) ) ;
#9560=CARTESIAN_POINT ( 'NONE',  ( -6.092822981423666739, 54.21481371789855785, -14.25334919248795096 ) ) ;
#9564=CARTESIAN_POINT ( 'NONE',  ( 6.932735513423970097, 92.34768628210144925, 10.69584247140445044 ) ) ;
#9565=CARTESIAN_POINT ( 'NONE',  ( 14.38691631536207538, 25.93518628210144072, -5.770363421893813793 ) ) ;
#9569=CARTESIAN_POINT ( 'NONE',  ( 3.257655550457285720, 52.09768628210144925, -15.46528703574804986 ) ) ;
#9576=CARTESIAN_POINT ( 'NONE',  ( -12.53471296425194836, 21.62268628210144072, 2.311890736173176641 ) ) ;
#9578=CARTESIAN_POINT ( 'NONE',  ( -6.840914352311947333, 136.4398137178985735, -6.594114490232462877 ) ) ;
#9588=CARTESIAN_POINT ( 'NONE',  ( 2.311890736173175753, 46.92268628210144499, 12.53471296425194659 ) ) ;
#9594=DIRECTION ( 'NONE',  ( 1.000000000000000000, -0.000000000000000000, 1.052579609121344151E-14 ) ) ;
#9597=CARTESIAN_POINT ( 'NONE',  ( 2.311890736173175753, 92.92268628210145209, 12.53471296425194836 ) ) ;
#9598=CARTESIAN_POINT ( 'NONE',  ( 3.257655550456945548, 22.30231371789854933, 15.46528703574811736 ) ) ;
#9604=CARTESIAN_POINT ( 'NONE',  ( 12.46528703574811558, 139.6023137178985394, -2.660918448318005503 ) ) ;
#9611=CARTESIAN_POINT ( 'NONE',  ( -8.927990412390371944, 109.1273137178985451, -13.04141134922778988 ) ) ;
#9614=CARTESIAN_POINT ( 'NONE',  ( 2.660918448318279950, 24.49768628210144783, -12.46528703574805697 ) ) ;
#9618=CARTESIAN_POINT ( 'NONE',  ( 8.632099005475504683, 110.7476862821014691, 13.23911966647218996 ) ) ;
#9620=CARTESIAN_POINT ( 'NONE',  ( 1.715153634034233487, 56.12268628210142651, 9.534712964251941258 ) ) ;
#9624=CARTESIAN_POINT ( 'NONE',  ( 12.46528703574805874, 81.99768628210146915, 2.660918448318279950 ) ) ;
#9636=CARTESIAN_POINT ( 'NONE',  ( 6.932735513424201024, 101.6523137178985650, -10.69584247140429412 ) ) ;
#9637=CARTESIAN_POINT ( 'NONE',  ( -4.944772684328673229, 112.1851862821014549, 11.48171059495397728 ) ) ;
#9643=CARTESIAN_POINT ( 'NONE',  ( -8.927990412390371944, 81.52731371789856496, -13.04141134922778988 ) ) ;
#9646=CARTESIAN_POINT ( 'NONE',  ( 3.796722387233379514, 107.5851862821014748, -8.710071997420127943 ) ) ;
#9649=CARTESIAN_POINT ( 'NONE',  ( -0.1745138560723084320, 54.78981371789855359, -9.500000000000005329 ) ) ;
#9651=CARTESIAN_POINT ( 'NONE',  ( 8.152565276336593669, 103.9523137178985763, 5.233372021372610483 ) ) ;
#9653=CARTESIAN_POINT ( 'NONE',  ( 12.46528703574811558, 38.40231371789855075, -2.660918448318005503 ) ) ;
#9655=CARTESIAN_POINT ( 'NONE',  ( 8.715434833791931624, 82.86018628210145209, 8.962234695871760692 ) ) ;
#9660=CARTESIAN_POINT ( 'NONE',  ( -10.83675517735155047, 78.26018628210144357, -11.08355503943142750 ) ) ;
#9665=CARTESIAN_POINT ( 'NONE',  ( 6.594114490232313663, 119.6601862821014635, 6.840914352312096547 ) ) ;
#9667=CARTESIAN_POINT ( 'NONE',  ( 12.46528703574805874, 127.9976862821014407, 2.660918448318279950 ) ) ;
#9679=CARTESIAN_POINT ( 'NONE',  ( 5.529263428287300108, 21.72731371789853938, 7.954856959092309943 ) ) ;
#9684=CARTESIAN_POINT ( 'NONE',  ( 12.50000000000000355, 20.28981371789855004, -0.1745138560722771515 ) ) ;
#9686=CARTESIAN_POINT ( 'NONE',  ( -15.50000000000000533, 135.2898137178985394, 0.1745138560722471477 ) ) ;
#9694=CARTESIAN_POINT ( 'NONE',  ( -7.228626920339069173, 130.8726862821014834, 10.49813415415989581 ) ) ;
#9706=CARTESIAN_POINT ( 'NONE',  ( -3.257655550457281723, 130.2976862821014379, 15.46528703574804986 ) ) ;
#9708=CARTESIAN_POINT ( 'NONE',  ( -2.064181346179269738, 121.0976862821014635, 9.465287035748067623 ) ) ;
#9712=CARTESIAN_POINT ( 'NONE',  ( -8.962234695871760692, 39.16018628210144215, 8.715434833791933400 ) ) ;
#9716=CARTESIAN_POINT ( 'NONE',  ( -0.1745138560725817967, 130.0101862821014436, 15.50000000000000533 ) ) ;
#9718=CARTESIAN_POINT ( 'NONE',  ( 3.474262827703532341, 138.1648137178985678, -8.843639120294245259 ) ) ;
#9728=CARTESIAN_POINT ( 'NONE',  ( 9.465287035748106703, 84.40231371789855075, -2.064181346179063237 ) ) ;
#9732=CARTESIAN_POINT ( 'NONE',  ( 8.962234695871567070, 76.63981371789856212, 8.715434833792127023 ) ) ;
#9736=CARTESIAN_POINT ( 'NONE',  ( 10.69584247140429589, 39.55231371789855643, 6.932735513424201024 ) ) ;
#9741=CARTESIAN_POINT ( 'NONE',  ( -10.69584247140444866, 30.24768628210144783, 6.932735513423972762 ) ) ;
#9745=CARTESIAN_POINT ( 'NONE',  ( 0.1745138560722779009, 86.98981371789855643, 12.50000000000000355 ) ) ;
#9750=CARTESIAN_POINT ( 'NONE',  ( 10.83675517735179206, 55.93981371789855217, -11.08355503943118769 ) ) ;
#9752=CARTESIAN_POINT ( 'NONE',  ( -0.1745138560725500443, 84.01018628210145778, 12.50000000000000355 ) ) ;
#9753=CARTESIAN_POINT ( 'NONE',  ( 15.50000000000000533, 35.71018628210144641, 0.1745138560725827404 ) ) ;
#9758=CARTESIAN_POINT ( 'NONE',  ( 8.927990412390657937, 43.47268628210144215, -13.04141134922759804 ) ) ;
#9763=CARTESIAN_POINT ( 'NONE',  ( -4.944772684328673229, 20.18518628210144783, 11.48171059495397728 ) ) ;
#9764=CARTESIAN_POINT ( 'NONE',  ( 8.152565276336593669, 122.3523137178985394, 5.233372021372610483 ) ) ;
#9768=CARTESIAN_POINT ( 'NONE',  ( -12.46528703574811558, 135.0023137178985451, 2.660918448318004170 ) ) ;
#9773=CARTESIAN_POINT ( 'NONE',  ( 2.311890736173175753, 56.12268628210144783, 12.53471296425194659 ) ) ;
#9782=CARTESIAN_POINT ( 'NONE',  ( -12.46528703574805697, 77.39768628210144641, -2.660918448318280838 ) ) ;
#9783=CARTESIAN_POINT ( 'NONE',  ( -2.908627838312453306, 22.87731371789854151, 15.53471296425188797 ) ) ;
#9789=CARTESIAN_POINT ( 'NONE',  ( 6.932735513424201024, 138.4523137178985621, -10.69584247140429412 ) ) ;
#9794=CARTESIAN_POINT ( 'NONE',  ( -14.38691631536193860, 117.4648137178985650, -5.770363421894132649 ) ) ;
#9797=CARTESIAN_POINT ( 'NONE',  ( 10.49813415415989581, 36.57268628210145067, 7.228626920339068285 ) ) ;
#9801=CARTESIAN_POINT ( 'NONE',  ( -11.08355503943142573, 103.5601862821014407, 10.83675517735155402 ) ) ;
#9805=CARTESIAN_POINT ( 'NONE',  ( 3.796722387233379514, 33.98518628210143788, -8.710071997420127943 ) ) ;
#9809=CARTESIAN_POINT ( 'NONE',  ( 2.311890736173175753, 83.72268628210143504, 12.53471296425194836 ) ) ;
#9812=CARTESIAN_POINT ( 'NONE',  ( 0.1745138560725194299, 42.61018628210144499, -9.500000000000005329 ) ) ;
#9821=CARTESIAN_POINT ( 'NONE',  ( 4.944772684328420986, 95.61481371789857064, 11.48171059495408208 ) ) ;
#9822=CARTESIAN_POINT ( 'NONE',  ( -10.49813415415989404, 105.5726862821014578, -7.228626920339069173 ) ) ;
#9827=CARTESIAN_POINT ( 'NONE',  ( -5.770363421894122880, 69.16481371789853938, 14.38691631536194393 ) ) ;
#9831=CARTESIAN_POINT ( 'NONE',  ( 2.064181346179272847, 107.2976862821014521, -9.465287035748065847 ) ) ;
#9833=CARTESIAN_POINT ( 'NONE',  ( 6.840914352311949109, 58.23981371789854222, 6.594114490232462877 ) ) ;
#9836=CARTESIAN_POINT ( 'NONE',  ( -9.500000000000005329, 116.8898137178985621, 0.1745138560723101806 ) ) ;
#9838=CARTESIAN_POINT ( 'NONE',  ( 10.49813415416005213, 28.62731371789854506, -7.228626920338837358 ) ) ;
#9840=CARTESIAN_POINT ( 'NONE',  ( 6.932735513423970097, 83.14768628210144641, 10.69584247140445044 ) ) ;
#9849=CARTESIAN_POINT ( 'NONE',  ( 9.500000000000005329, 118.5101862821014720, 0.1745138560725188748 ) ) ;
#9851=CARTESIAN_POINT ( 'NONE',  ( -4.622313124798576922, 124.8351862821014748, -11.61527771782819762 ) ) ;
#9862=CARTESIAN_POINT ( 'NONE',  ( -3.474262827703527901, 23.16481371789855359, 8.843639120294245259 ) ) ;
#9867=CARTESIAN_POINT ( 'NONE',  ( -8.962234695871565293, 26.03981371789855359, -8.715434833792128799 ) ) ;
#9869=CARTESIAN_POINT ( 'NONE',  ( 2.908627838312458636, 128.6773137178985280, -15.53471296425188442 ) ) ;
#9877=CARTESIAN_POINT ( 'NONE',  ( 4.622313124798573369, 129.4351862821014549, 11.61527771782819940 ) ) ;
#9888=CARTESIAN_POINT ( 'NONE',  ( -11.08355503943142573, 131.1601862821014777, 10.83675517735155402 ) ) ;
#9890=CARTESIAN_POINT ( 'NONE',  ( 9.465287035748067623, 109.5976862821014493, 2.064181346179272847 ) ) ;
#9892=CARTESIAN_POINT ( 'NONE',  ( 10.49813415415989581, 27.37268628210144783, 7.228626920339068285 ) ) ;
#9896=CARTESIAN_POINT ( 'NONE',  ( 15.46528703574804986, 127.9976862821014265, 3.257655550457285720 ) ) ;
#9898=CARTESIAN_POINT ( 'NONE',  ( -8.843639120294245259, 135.8648137178985849, -3.474262827703533230 ) ) ;
#9906=CARTESIAN_POINT ( 'NONE',  ( 7.954856959092311719, 74.62731371789853085, -5.529263428287300108 ) ) ;
#9909=CARTESIAN_POINT ( 'NONE',  ( 10.69584247140429589, 76.35231371789855359, 6.932735513424201024 ) ) ;
#9911=CARTESIAN_POINT ( 'NONE',  ( -7.578999853579856172, 143.0000000000000284, 10.66724312669795083 ) ) ;
#9913=CARTESIAN_POINT ( 'NONE',  ( 7.228626920338837358, 49.32731371789855501, 10.49813415416005036 ) ) ;
#9918=CARTESIAN_POINT ( 'NONE',  ( -8.962234695871760692, 29.96018628210143930, 8.715434833791933400 ) ) ;
#9922=CARTESIAN_POINT ( 'NONE',  ( -10.49813415416004858, 79.22731371789855359, 7.228626920338839135 ) ) ;
#9923=EDGE_CURVE ( 'NONE', #1210, #5242, #12143, .T. ) ;
#9930=CARTESIAN_POINT ( 'NONE',  ( -8.632099005475794229, 51.05231371789854222, 13.23911966647199812 ) ) ;
#9933=CARTESIAN_POINT ( 'NONE',  ( 8.962234695871762469, 80.56018628210145494, -8.715434833791931624 ) ) ;
#9934=CARTESIAN_POINT ( 'NONE',  ( 11.08355503943142750, 25.36018628210144854, -10.83675517735155225 ) ) ;
#9939=CARTESIAN_POINT ( 'NONE',  ( 5.770363421893814682, 46.63518628210144357, 14.38691631536207183 ) ) ;
#9945=CARTESIAN_POINT ( 'NONE',  ( 0.1745138560725515708, 24.21018628210144641, -12.50000000000000355 ) ) ;
#9947=CARTESIAN_POINT ( 'NONE',  ( -5.233372021372612259, 133.8523137178985394, 8.152565276336593669 ) ) ;
#9952=CARTESIAN_POINT ( 'NONE',  ( 4.622313124798831829, 128.9648137178985507, -11.61527771782809282 ) ) ;
#9958=CARTESIAN_POINT ( 'NONE',  ( -10.69584247140444866, 57.84768628210144925, 6.932735513423972762 ) ) ;
#9966=CARTESIAN_POINT ( 'NONE',  ( 10.69584247140445221, 71.64768628210146062, -6.932735513423970097 ) ) ;
#9967=CARTESIAN_POINT ( 'NONE',  ( -6.092822981423970496, 139.7851862821014493, 14.25334919248782661 ) ) ;
#9973=CARTESIAN_POINT ( 'NONE',  ( -6.840914352311947333, 7.639813717898540801, -6.594114490232462877 ) ) ;
#9979=CARTESIAN_POINT ( 'NONE',  ( 3.257655550456945548, 105.1023137178985678, 15.46528703574811736 ) ) ;
#9982=CARTESIAN_POINT ( 'NONE',  ( 8.715434833791931624, 27.66018628210144215, 8.962234695871760692 ) ) ;
#9986=CARTESIAN_POINT ( 'NONE',  ( -14.38691631536207183, 104.1351862821014720, 5.770363421893814682 ) ) ;
#9989=CARTESIAN_POINT ( 'NONE',  ( 5.529263428287477744, 43.47268628210144215, -7.954856959092191815 ) ) ;
#9993=CARTESIAN_POINT ( 'NONE',  ( 12.53471296425194836, 81.42268628210145209, -2.311890736173178418 ) ) ;
#9996=CARTESIAN_POINT ( 'NONE',  ( 9.465287035748067623, 45.19768628210142225, 2.064181346179272847 ) ) ;
#10006=CARTESIAN_POINT ( 'NONE',  ( -6.932735513424201912, 78.65231371789855075, 10.69584247140429412 ) ) ;
#10007=CARTESIAN_POINT ( 'NONE',  ( -12.50000000000000355, 104.7101862821014606, -0.1745138560725492671 ) ) ;
#10012=CARTESIAN_POINT ( 'NONE',  ( 13.04141134922778988, 74.62731371789853085, -8.927990412390371944 ) ) ;
#10018=CARTESIAN_POINT ( 'NONE',  ( 2.064181346179061460, 49.90231371789854364, 9.465287035748106703 ) ) ;
#10020=CARTESIAN_POINT ( 'NONE',  ( -8.152565276336593669, 108.5523137178985422, -5.233372021372610483 ) ) ;
#10022=CARTESIAN_POINT ( 'NONE',  ( -12.46528703574811558, 33.80231371789854933, 2.660918448318003726 ) ) ;
#10023=CARTESIAN_POINT ( 'NONE',  ( 8.962234695871762469, 80.56018628210145494, -8.715434833791931624 ) ) ;
#10031=CARTESIAN_POINT ( 'NONE',  ( 8.710071997420127943, 100.6851862821014834, 3.796722387233375073 ) ) ;
#10034=CARTESIAN_POINT ( 'NONE',  ( 11.61527771782819940, 136.3351862821014606, -4.622313124798573369 ) ) ;
#10049=CARTESIAN_POINT ( 'NONE',  ( 5.529263428287300108, 12.52731371789855963, 7.954856959092309943 ) ) ;
#10054=CARTESIAN_POINT ( 'NONE',  ( -10.49813415416004858, 24.02731371789855430, 7.228626920338840023 ) ) ;
#10056=CARTESIAN_POINT ( 'NONE',  ( 5.770363421894130873, 128.9648137178985792, -14.38691631536193860 ) ) ;
#10063=CARTESIAN_POINT ( 'NONE',  ( -10.69584247140444866, 131.4476862821014436, 6.932735513423972762 ) ) ;
#10074=CARTESIAN_POINT ( 'NONE',  ( -2.660918448318275509, 139.4976862821014549, 12.46528703574805874 ) ) ;
#10079=CARTESIAN_POINT ( 'NONE',  ( 5.770363421894130873, 9.364813717898543999, -14.38691631536193860 ) ) ;
#10082=CARTESIAN_POINT ( 'NONE',  ( -8.710071997420127943, 114.4851862821014663, -3.796722387233380402 ) ) ;
#10084=CARTESIAN_POINT ( 'NONE',  ( -10.69584247140444866, 21.04768628210144854, 6.932735513423972762 ) ) ;
#10088=CARTESIAN_POINT ( 'NONE',  ( 13.04141134922759804, 128.5726862821014436, 8.927990412390657937 ) ) ;
#10090=CARTESIAN_POINT ( 'NONE',  ( 6.840914352312096547, 6.960186282101432198, -6.594114490232313663 ) ) ;
#10096=CARTESIAN_POINT ( 'NONE',  ( 8.843639120294245259, 66.86481371789854222, 3.474262827703527901 ) ) ;
#10099=CARTESIAN_POINT ( 'NONE',  ( -4.944772684328424539, 81.81481371789855928, -11.48171059495408031 ) ) ;
#10104=CARTESIAN_POINT ( 'NONE',  ( 12.53471296425189330, 48.17731371789854933, 2.311890736173451977 ) ) ;
#10108=CARTESIAN_POINT ( 'NONE',  ( -2.660918448318275509, 29.09768628210144925, 12.46528703574805874 ) ) ;
#10114=CARTESIAN_POINT ( 'NONE',  ( -8.962234695871565293, 72.03981371789855359, -8.715434833792128799 ) ) ;
#10119=CARTESIAN_POINT ( 'NONE',  ( -8.927990412390371944, 63.12731371789852375, -13.04141134922778988 ) ) ;
#10122=CARTESIAN_POINT ( 'NONE',  ( 7.228626920339068285, 89.47268628210144925, -10.49813415415989581 ) ) ;
#10123=CARTESIAN_POINT ( 'NONE',  ( -13.04141134922759804, 31.97268628210143149, -8.927990412390657937 ) ) ;
#10127=CARTESIAN_POINT ( 'NONE',  ( -15.53471296425195369, 30.82268628210143291, 2.908627838312118019 ) ) ;
#10134=CARTESIAN_POINT ( 'NONE',  ( 10.49813415415989581, 18.17268628210144854, 7.228626920339068285 ) ) ;
#10136=CARTESIAN_POINT ( 'NONE',  ( 1.715153634034445762, 137.8773137178985735, -9.534712964251895073 ) ) ;
#10141=CARTESIAN_POINT ( 'NONE',  ( -10.69584247140429412, 126.9523137178985621, -6.932735513424201024 ) ) ;
#10147=CARTESIAN_POINT ( 'NONE',  ( -12.50000000000000355, 31.11018628210143788, -0.1745138560725492671 ) ) ;
#10154=CARTESIAN_POINT ( 'NONE',  ( -2.660918448318275509, 84.29768628210145209, 12.46528703574805874 ) ) ;
#10155=CARTESIAN_POINT ( 'NONE',  ( 5.770363421893814682, 138.6351862821014720, 14.38691631536207183 ) ) ;
#10161=CARTESIAN_POINT ( 'NONE',  ( -8.715434833792127023, 143.3398137178985507, 8.962234695871568846 ) ) ;
#10168=CARTESIAN_POINT ( 'NONE',  ( 14.38691631536194393, 122.0648137178985877, 5.770363421894124656 ) ) ;
#10172=CARTESIAN_POINT ( 'NONE',  ( -12.50000000000000355, 132.3101862821014549, -0.1745138560725492671 ) ) ;
#10175=CARTESIAN_POINT ( 'NONE',  ( 14.38691631536207538, 99.53518628210146346, -5.770363421893813793 ) ) ;
#10178=CARTESIAN_POINT ( 'NONE',  ( -8.152565276336710909, 48.64768628210144641, 5.233372021372435512 ) ) ;
#10182=CARTESIAN_POINT ( 'NONE',  ( -2.311890736173176641, 69.92268628210146630, -12.53471296425194836 ) ) ;
#10185=CARTESIAN_POINT ( 'NONE',  ( -1.715153634034234598, 42.32268628210145067, -9.534712964251941258 ) ) ;
#10196=CARTESIAN_POINT ( 'NONE',  ( -8.962234695871565293, 90.43981371789855928, -8.715434833792128799 ) ) ;
#10197=CARTESIAN_POINT ( 'NONE',  ( 12.46528703574805874, 81.99768628210145494, 2.660918448318279950 ) ) ;
#10204=CARTESIAN_POINT ( 'NONE',  ( -11.08355503943118592, 62.83981371789855785, -10.83675517735179383 ) ) ;
#10209=CARTESIAN_POINT ( 'NONE',  ( 9.534712964251900402, 57.37731371789855928, 1.715153634034445540 ) ) ;
#10212=CARTESIAN_POINT ( 'NONE',  ( 0.1745138560723095977, 105.3898137178985479, 9.500000000000005329 ) ) ;
#10214=CARTESIAN_POINT ( 'NONE',  ( 10.69584247140429589, 30.35231371789855359, 6.932735513424201024 ) ) ;
#10215=CARTESIAN_POINT ( 'NONE',  ( -4.622313124798576922, 78.83518628210146062, -11.61527771782819762 ) ) ;
#10223=CARTESIAN_POINT ( 'NONE',  ( 9.534712964251941258, 99.82268628210142936, -1.715153634034235708 ) ) ;
#10225=CARTESIAN_POINT ( 'NONE',  ( -2.311890736173176641, 134.3226862821014436, -12.53471296425194836 ) ) ;
#10235=CARTESIAN_POINT ( 'NONE',  ( -0.1745138560722763466, 137.5898137178985792, -12.50000000000000355 ) ) ;
#10240=CARTESIAN_POINT ( 'NONE',  ( -11.48171059495408208, 33.51481371789854791, 4.944772684328421875 ) ) ;
#10242=CARTESIAN_POINT ( 'NONE',  ( 13.04141134922778988, 120.6273137178985451, -8.927990412390371944 ) ) ;
#10249=CARTESIAN_POINT ( 'NONE',  ( 11.61527771782819940, 127.1351862821014578, -4.622313124798573369 ) ) ;
#10256=CARTESIAN_POINT ( 'NONE',  ( 2.311890736173175753, 138.9226862821014663, 12.53471296425194836 ) ) ;
#10262=CARTESIAN_POINT ( 'NONE',  ( 2.908627838312118019, 111.3226862821014578, 15.53471296425195369 ) ) ;
#10263=CARTESIAN_POINT ( 'NONE',  ( 5.233372021372432847, 110.7476862821014691, 8.152565276336710909 ) ) ;
#10266=CARTESIAN_POINT ( 'NONE',  ( 7.228626920339068285, 6.672686282101436106, -10.49813415415989581 ) ) ;
#10270=CARTESIAN_POINT ( 'NONE',  ( -5.233372021372430183, 87.74768628210144072, -8.152565276336710909 ) ) ;
#10272=CARTESIAN_POINT ( 'NONE',  ( -5.233372021372612259, 133.8523137178985394, 8.152565276336593669 ) ) ;
#10279=CARTESIAN_POINT ( 'NONE',  ( -3.796722387233185003, 63.41481371789855359, -8.710071997420207879 ) ) ;
#10282=CARTESIAN_POINT ( 'NONE',  ( 6.932735513424201024, 83.25231371789857349, -10.69584247140429412 ) ) ;
#10286=CARTESIAN_POINT ( 'NONE',  ( -4.944772684328424539, 45.01481371789854791, -11.48171059495408031 ) ) ;
#10291=CARTESIAN_POINT ( 'NONE',  ( 12.50000000000000355, 26.51018628210144357, 0.1745138560725507937 ) ) ;
#10296=CARTESIAN_POINT ( 'NONE',  ( -8.715434833792127023, 69.73981371789855643, 8.962234695871568846 ) ) ;
#10302=CARTESIAN_POINT ( 'NONE',  ( -2.908627838312453306, 41.27731371789855075, 15.53471296425188797 ) ) ;
#10306=CARTESIAN_POINT ( 'NONE',  ( -0.1745138560725500443, 65.61018628210145209, 12.50000000000000355 ) ) ;
#10307=CARTESIAN_POINT ( 'NONE',  ( -15.50000000000000533, 31.11018628210143433, -0.1745138560725808530 ) ) ;
#10311=CARTESIAN_POINT ( 'NONE',  ( -13.23911966647218463, 30.24768628210144783, 8.632099005475506459 ) ) ;
#10319=CARTESIAN_POINT ( 'NONE',  ( -5.233372021372612259, 124.6523137178985650, 8.152565276336593669 ) ) ;
#10327=CARTESIAN_POINT ( 'NONE',  ( -7.228626920338836470, 136.7273137178985678, -10.49813415416005213 ) ) ;
#10333=CARTESIAN_POINT ( 'NONE',  ( -4.944772684328673229, 29.38518628210144712, 11.48171059495397728 ) ) ;
#10341=CARTESIAN_POINT ( 'NONE',  ( 8.962234695871762469, 80.56018628210145494, -8.715434833791931624 ) ) ;
#10342=CARTESIAN_POINT ( 'NONE',  ( 13.04141134922778988, 10.22731371789853405, -8.927990412390371944 ) ) ;
#10347=CARTESIAN_POINT ( 'NONE',  ( 0.1745138560722779009, 123.7898137178985678, 12.50000000000000355 ) ) ;
#10354=CARTESIAN_POINT ( 'NONE',  ( 2.908627838312458636, 91.87731371789854506, -15.53471296425188442 ) ) ;
#10359=CARTESIAN_POINT ( 'NONE',  ( -12.50000000000000355, 123.1101862821014663, -0.1745138560725492671 ) ) ;
#10360=CARTESIAN_POINT ( 'NONE',  ( -15.50000000000000533, 77.11018628210145209, -0.1745138560725808530 ) ) ;
#10363=CARTESIAN_POINT ( 'NONE',  ( -15.53471296425195369, 86.02268628210144641, 2.908627838312118019 ) ) ;
#10366=CARTESIAN_POINT ( 'NONE',  ( 6.840914352312096547, 34.56018628210144783, -6.594114490232313663 ) ) ;
#10370=CARTESIAN_POINT ( 'NONE',  ( -10.49813415415989581, 50.37268628210145494, -7.228626920339068285 ) ) ;
#10373=CARTESIAN_POINT ( 'NONE',  ( 9.534712964251941258, 35.42268628210144499, -1.715153634034235708 ) ) ;
#10382=CARTESIAN_POINT ( 'NONE',  ( 6.932735513424201024, 83.25231371789857349, -10.69584247140429412 ) ) ;
#10383=CARTESIAN_POINT ( 'NONE',  ( 10.49813415415989581, 91.77268628210144641, 7.228626920339069173 ) ) ;
#10388=CARTESIAN_POINT ( 'NONE',  ( 0.1745138560722461762, 50.18981371789855217, 15.50000000000000533 ) ) ;
#10393=CARTESIAN_POINT ( 'NONE',  ( -9.465287035748106703, 43.00231371789853796, 2.064181346179061460 ) ) ;
#10398=CARTESIAN_POINT ( 'NONE',  ( 5.529263428287300108, 95.32731371789854791, 7.954856959092309943 ) ) ;
#10400=CARTESIAN_POINT ( 'NONE',  ( -12.50000000000000355, 24.88981371789854435, 0.1745138560722786503 ) ) ;
#10402=CARTESIAN_POINT ( 'NONE',  ( 2.660918448318279950, 88.89768628210146062, -12.46528703574805697 ) ) ;
#10411=CARTESIAN_POINT ( 'NONE',  ( -0.1745138560725182642, 93.21018628210146062, 9.500000000000005329 ) ) ;
#10413=CARTESIAN_POINT ( 'NONE',  ( -6.932735513423968321, 124.5476862821014663, -10.69584247140445221 ) ) ;
#10414=CARTESIAN_POINT ( 'NONE',  ( -11.00000000000001421, 143.0000000000000000, 1.001863997985030341 ) ) ;
#10424=CARTESIAN_POINT ( 'NONE',  ( 7.228626920338837358, 141.3273137178985337, 10.49813415416005036 ) ) ;
#10432=CARTESIAN_POINT ( 'NONE',  ( -8.632099005475794229, 106.2523137178985451, 13.23911966647199812 ) ) ;
#10438=CARTESIAN_POINT ( 'NONE',  ( 8.962234695871762469, 126.5601862821014691, -8.715434833791931624 ) ) ;
#10449=CARTESIAN_POINT ( 'NONE',  ( 11.08355503943142750, 126.5601862821014834, -10.83675517735155225 ) ) ;
#10450=CARTESIAN_POINT ( 'NONE',  ( -0.1745138560725500443, 19.61018628210144144, 12.50000000000000355 ) ) ;
#10455=CARTESIAN_POINT ( 'NONE',  ( 5.529263428287477744, 89.47268628210143504, -7.954856959092191815 ) ) ;
#10456=CARTESIAN_POINT ( 'NONE',  ( -6.594114490232462877, 134.1398137178985621, 6.840914352311949109 ) ) ;
#10462=CARTESIAN_POINT ( 'NONE',  ( -5.529263428287297444, 53.92731371789854222, -7.954856959092311719 ) ) ;
#10467=CARTESIAN_POINT ( 'NONE',  ( -6.932735513424201912, 60.25231371789854506, 10.69584247140429412 ) ) ;
#10471=CARTESIAN_POINT ( 'NONE',  ( -4.622313124798826500, 23.16481371789855359, 11.61527771782809637 ) ) ;
#10474=CARTESIAN_POINT ( 'NONE',  ( 12.50000000000000355, 17.31018628210144428, 0.1745138560725507937 ) ) ;
#10478=CARTESIAN_POINT ( 'NONE',  ( -0.1745138560722763466, 73.18981371789855928, -12.50000000000000355 ) ) ;
#10484=CARTESIAN_POINT ( 'NONE',  ( -5.770363421894122880, 41.56481371789855217, 14.38691631536194393 ) ) ;
#10488=CARTESIAN_POINT ( 'NONE',  ( 11.61527771782819940, 71.93518628210145494, -4.622313124798573369 ) ) ;
#10489=CARTESIAN_POINT ( 'NONE',  ( 3.257655550457285720, 15.29768628210142722, -15.46528703574804986 ) ) ;
#10493=CARTESIAN_POINT ( 'NONE',  ( 15.46528703574804986, 26.79768628210144144, 3.257655550457285720 ) ) ;
#10496=CARTESIAN_POINT ( 'NONE',  ( -12.50000000000000355, 6.489813717898557321, 0.1745138560722785670 ) ) ;
#10499=CARTESIAN_POINT ( 'NONE',  ( 10.69584247140445221, 7.247686282101428290, -6.932735513423970097 ) ) ;
#10503=CARTESIAN_POINT ( 'NONE',  ( -5.529263428287297444, 109.1273137178985451, -7.954856959092311719 ) ) ;
#10507=CARTESIAN_POINT ( 'NONE',  ( 0.1745138560722779009, 142.1898137178985735, 12.50000000000000355 ) ) ;
#10514=CARTESIAN_POINT ( 'NONE',  ( -12.46528703574805874, 31.39768628210144641, -2.660918448318280838 ) ) ;
#10523=CARTESIAN_POINT ( 'NONE',  ( 11.48171059495397728, 73.08518628210144641, 4.944772684328674117 ) ) ;
#10524=CARTESIAN_POINT ( 'NONE',  ( 13.04141134922759804, 137.7726862821014606, 8.927990412390657937 ) ) ;
#10532=CARTESIAN_POINT ( 'NONE',  ( 6.932735513424201024, 129.2523137178985451, -10.69584247140429412 ) ) ;
#10537=CARTESIAN_POINT ( 'NONE',  ( -14.38691631536193860, 99.06481371789857349, -5.770363421894132649 ) ) ;
#10542=CARTESIAN_POINT ( 'NONE',  ( 10.69584247140445221, 117.6476862821014464, -6.932735513423970097 ) ) ;
#10543=CARTESIAN_POINT ( 'NONE',  ( -15.53471296425195369, 67.62268628210145494, 2.908627838312118019 ) ) ;
#10547=CARTESIAN_POINT ( 'NONE',  ( 13.04141134922759804, 91.77268628210144641, 8.927990412390657937 ) ) ;
#10552=CARTESIAN_POINT ( 'NONE',  ( 9.465287035748067623, 45.19768628210142225, 2.064181346179272847 ) ) ;
#10555=CARTESIAN_POINT ( 'NONE',  ( 7.228626920339068285, 61.87268628210145494, -10.49813415415989581 ) ) ;
#10558=CARTESIAN_POINT ( 'NONE',  ( 5.233372021372432847, 18.74768628210143362, 8.152565276336710909 ) ) ;
#10567=CARTESIAN_POINT ( 'NONE',  ( 2.660918448318002838, 86.70231371789854791, 12.46528703574811558 ) ) ;
#10568=CARTESIAN_POINT ( 'NONE',  ( -4.622313124798576922, 88.03518628210144925, -11.61527771782819762 ) ) ;
#10574=CARTESIAN_POINT ( 'NONE',  ( -8.632099005475794229, 51.05231371789854222, 13.23911966647199812 ) ) ;
#10579=CARTESIAN_POINT ( 'NONE',  ( 6.594114490232462877, 46.73981371789855643, -6.840914352311949109 ) ) ;
#10582=CARTESIAN_POINT ( 'NONE',  ( -8.152565276336593669, 90.15231371789855075, -5.233372021372610483 ) ) ;
#10584=CARTESIAN_POINT ( 'NONE',  ( -12.46528703574811558, 15.40231371789854542, 2.660918448318003726 ) ) ;
#10585=CARTESIAN_POINT ( 'NONE',  ( -4.944772684328673229, 56.98518628210144499, 11.48171059495397728 ) ) ;
#10592=CARTESIAN_POINT ( 'NONE',  ( -7.954856959092191815, 87.17268628210142367, -5.529263428287477744 ) ) ;
#10594=CARTESIAN_POINT ( 'NONE',  ( 4.944772684328679446, 116.7851862821014635, -11.48171059495397373 ) ) ;
#10607=CARTESIAN_POINT ( 'NONE',  ( -12.50000000000000355, 144.4898137178985564, 0.1745138560722786503 ) ) ;
#10613=CARTESIAN_POINT ( 'NONE',  ( -10.69584247140429412, 7.352313717898545598, -6.932735513424201024 ) ) ;
#10616=CARTESIAN_POINT ( 'NONE',  ( -11.08355503943118592, 118.0398137178985536, -10.83675517735179383 ) ) ;
#10622=CARTESIAN_POINT ( 'NONE',  ( 10.49813415415989581, 119.3726862821014549, 7.228626920339068285 ) ) ;
#10634=CARTESIAN_POINT ( 'NONE',  ( 14.25334919248782661, 119.0851862821014606, 6.092822981423971385 ) ) ;
#10636=CARTESIAN_POINT ( 'NONE',  ( -2.311890736173176641, 14.72268628210143859, -12.53471296425194836 ) ) ;
#10639=CARTESIAN_POINT ( 'NONE',  ( -13.99999999999999467, 143.0000000000000000, -1.543483589373963192E-13 ) ) ;
#10640=CARTESIAN_POINT ( 'NONE',  ( -7.954856959092191815, 87.17268628210142367, -5.529263428287477744 ) ) ;
#10642=CARTESIAN_POINT ( 'NONE',  ( 9.465287035748106703, 130.4023137178985792, -2.064181346179063237 ) ) ;
#10649=CARTESIAN_POINT ( 'NONE',  ( 2.064181346179061460, 59.10231371789854649, 9.465287035748106703 ) ) ;
#10653=CARTESIAN_POINT ( 'NONE',  ( 12.50000000000000355, 66.28981371789855359, -0.1745138560722771515 ) ) ;
#10657=CARTESIAN_POINT ( 'NONE',  ( 11.48171059495408208, 28.91481371789854293, -4.944772684328420986 ) ) ;
#10667=CARTESIAN_POINT ( 'NONE',  ( -4.622313124798826500, 59.96481371789855075, 11.61527771782809637 ) ) ;
#10672=CARTESIAN_POINT ( 'NONE',  ( 10.83675517735179206, 46.73981371789855643, -11.08355503943118769 ) ) ;
#10674=CARTESIAN_POINT ( 'NONE',  ( -6.932735513423968321, 23.34768628210144570, -10.69584247140445221 ) ) ;
#10676=CARTESIAN_POINT ( 'NONE',  ( 0.1745138560725515708, 61.01018628210145067, -12.50000000000000355 ) ) ;
#10677=CARTESIAN_POINT ( 'NONE',  ( -6.092822981423970496, 10.98518628210143433, 14.25334919248782661 ) ) ;
#10681=CARTESIAN_POINT ( 'NONE',  ( 2.908627838312118019, 37.72268628210143504, 15.53471296425195369 ) ) ;
#10687=CARTESIAN_POINT ( 'NONE',  ( 11.48171059495397728, 8.685186282101437172, 4.944772684328674117 ) ) ;
#10689=CARTESIAN_POINT ( 'NONE',  ( -9.534712964251895073, 117.1773137178985706, -1.715153634034446428 ) ) ;
#10696=CARTESIAN_POINT ( 'NONE',  ( -12.50000000000000355, 126.0898137178985650, 0.1745138560722786503 ) ) ;
#10702=CARTESIAN_POINT ( 'NONE',  ( -7.228626920339070061, 29.67268628210143788, 10.49813415415989404 ) ) ;
#10710=CARTESIAN_POINT ( 'NONE',  ( 2.660918448318279950, 52.09768628210144215, -12.46528703574805697 ) ) ;
#10711=CARTESIAN_POINT ( 'NONE',  ( -14.38691631536207183, 140.9351862821014549, 5.770363421893814682 ) ) ;
#10718=CARTESIAN_POINT ( 'NONE',  ( -7.228626920338836470, 118.3273137178985621, -10.49813415416005213 ) ) ;
#10723=CARTESIAN_POINT ( 'NONE',  ( -8.927990412390371944, 99.92731371789854222, -13.04141134922778988 ) ) ;
#10727=CARTESIAN_POINT ( 'NONE',  ( -10.49813415415989581, 123.9726862821014493, -7.228626920339068285 ) ) ;
#10729=CARTESIAN_POINT ( 'NONE',  ( 15.46528703574804986, 63.59768628210142793, 3.257655550457285720 ) ) ;
#10733=CARTESIAN_POINT ( 'NONE',  ( 10.83675517735155225, 92.06018628210145494, 11.08355503943142573 ) ) ;
#10736=CARTESIAN_POINT ( 'NONE',  ( -0.1745138560725182642, 28.81018628210143717, 9.500000000000005329 ) ) ;
#10740=CARTESIAN_POINT ( 'NONE',  ( -7.228626920339069173, 66.47268628210144925, 10.49813415415989581 ) ) ;
#10743=CARTESIAN_POINT ( 'NONE',  ( -2.064181346179269738, 19.89768628210143930, 9.465287035748067623 ) ) ;
#10755=CARTESIAN_POINT ( 'NONE',  ( -4.944772684328424539, 81.81481371789855928, -11.48171059495408031 ) ) ;
#10756=CARTESIAN_POINT ( 'NONE',  ( 7.228626920339069173, 89.47268628210144925, -10.49813415415989404 ) ) ;
#10761=CARTESIAN_POINT ( 'NONE',  ( -14.38691631536193860, 62.26481371789854791, -5.770363421894132649 ) ) ;
#10766=CARTESIAN_POINT ( 'NONE',  ( 8.710071997420211432, 47.31481371789856638, -3.796722387233181895 ) ) ;
#10768=CARTESIAN_POINT ( 'NONE',  ( 0.1745138560723095977, 86.98981371789857064, 9.500000000000005329 ) ) ;
#10770=CARTESIAN_POINT ( 'NONE',  ( -0.1745138560722763466, 8.789813717898553591, -12.50000000000000355 ) ) ;
#10772=CARTESIAN_POINT ( 'NONE',  ( -10.69584247140444866, 57.84768628210144925, 6.932735513423972762 ) ) ;
#10781=CARTESIAN_POINT ( 'NONE',  ( 5.233372021372432847, 101.5476862821014663, 8.152565276336710909 ) ) ;
#10783=CARTESIAN_POINT ( 'NONE',  ( 10.69584247140445221, 117.6476862821014464, -6.932735513423970097 ) ) ;
#10797=CARTESIAN_POINT ( 'NONE',  ( 4.622313124798831829, 138.1648137178985678, -11.61527771782809282 ) ) ;
#10798=CARTESIAN_POINT ( 'NONE',  ( 10.69584247140445221, 136.0476862821014663, -6.932735513423970097 ) ) ;
#10803=CARTESIAN_POINT ( 'NONE',  ( -11.48171059495408208, 15.11481371789855110, 4.944772684328421875 ) ) ;
#10805=CARTESIAN_POINT ( 'NONE',  ( 14.25334919248795451, 120.9148137178985678, -6.092822981423661410 ) ) ;
#10811=CARTESIAN_POINT ( 'NONE',  ( -2.660918448318275509, 111.8976862821014606, 12.46528703574805874 ) ) ;
#10818=CARTESIAN_POINT ( 'NONE',  ( -11.48171059495397373, 123.6851862821014549, -4.944772684328680334 ) ) ;
#10823=CARTESIAN_POINT ( 'NONE',  ( 3.257655550457285720, 116.4976862821014549, -15.46528703574804986 ) ) ;
#10826=CARTESIAN_POINT ( 'NONE',  ( -11.48171059495397373, 13.28518628210142971, -4.944772684328680334 ) ) ;
#10830=CARTESIAN_POINT ( 'NONE',  ( -8.710071997420127943, 77.68518628210145494, -3.796722387233380402 ) ) ;
#10837=CARTESIAN_POINT ( 'NONE',  ( 1.715153634034445762, 64.27731371789853654, -9.534712964251895073 ) ) ;
#10842=CARTESIAN_POINT ( 'NONE',  ( 12.46528703574811558, 66.00231371789855928, -2.660918448318005947 ) ) ;
#10845=CARTESIAN_POINT ( 'NONE',  ( -6.932735513424201912, 32.65231371789854364, 10.69584247140429412 ) ) ;
#10855=CARTESIAN_POINT ( 'NONE',  ( -7.228626920338836470, 63.12731371789855217, -10.49813415416005213 ) ) ;
#10861=CARTESIAN_POINT ( 'NONE',  ( -6.092822981423666739, 35.81481371789853796, -14.25334919248795096 ) ) ;
#10863=CARTESIAN_POINT ( 'NONE',  ( 2.311890736173175753, 19.32268628210144712, 12.53471296425194836 ) ) ;
#10864=CARTESIAN_POINT ( 'NONE',  ( 2.660918448318279950, 70.49768628210145494, -12.46528703574805697 ) ) ;
#10866=CARTESIAN_POINT ( 'NONE',  ( -15.46528703574804986, 3.797686282101448096, -3.257655550457287497 ) ) ;
#10870=CARTESIAN_POINT ( 'NONE',  ( 2.908627838312118019, 28.52268628210144286, 15.53471296425195369 ) ) ;
#10878=CARTESIAN_POINT ( 'NONE',  ( -6.594114490232462877, 115.7398137178985564, 6.840914352311949109 ) ) ;
#10884=CARTESIAN_POINT ( 'NONE',  ( -10.49813415416004858, 125.2273137178985820, 7.228626920338840023 ) ) ;
#10898=CARTESIAN_POINT ( 'NONE',  ( -11.61527771782819940, 58.13518628210144357, 4.622313124798574258 ) ) ;
#10905=CARTESIAN_POINT ( 'NONE',  ( 2.660918448318002838, 114.3023137178985564, 12.46528703574811558 ) ) ;
#10910=CARTESIAN_POINT ( 'NONE',  ( 15.46528703574811736, 102.8023137178985422, -3.257655550456947768 ) ) ;
#10914=CARTESIAN_POINT ( 'NONE',  ( 0.1745138560725515708, 125.4101862821014635, -12.50000000000000355 ) ) ;
#10915=CARTESIAN_POINT ( 'NONE',  ( -5.770363421893818234, 60.43518628210146204, -14.38691631536207005 ) ) ;
#10919=CARTESIAN_POINT ( 'NONE',  ( 13.04141134922759804, 82.57268628210144357, 8.927990412390657937 ) ) ;
#10922=CARTESIAN_POINT ( 'NONE',  ( -8.152565276336710909, 21.04768628210144499, 5.233372021372435512 ) ) ;
#10926=CARTESIAN_POINT ( 'NONE',  ( -12.50000000000000355, 58.71018628210145351, -0.1745138560725492671 ) ) ;
#10929=CARTESIAN_POINT ( 'NONE',  ( -0.1745138560725182642, 28.81018628210143717, 9.500000000000005329 ) ) ;
#10942=CARTESIAN_POINT ( 'NONE',  ( -2.311890736173176641, 79.12268628210145494, -12.53471296425194659 ) ) ;
#10947=CARTESIAN_POINT ( 'NONE',  ( 15.46528703574811736, 56.80231371789854933, -3.257655550456947768 ) ) ;
#10952=CARTESIAN_POINT ( 'NONE',  ( -8.710071997420207879, 33.51481371789854791, 3.796722387233182339 ) ) ;
#10955=CARTESIAN_POINT ( 'NONE',  ( -8.710071997420207879, 88.71481371789855075, 3.796722387233182339 ) ) ;
#10957=CARTESIAN_POINT ( 'NONE',  ( -15.46528703574811736, 144.2023137178985905, 3.257655550456946436 ) ) ;
#10958=CARTESIAN_POINT ( 'NONE',  ( 12.46528703574805874, 63.59768628210145636, 2.660918448318279950 ) ) ;
#10966=CARTESIAN_POINT ( 'NONE',  ( -9.500000000000005329, 67.91018628210144925, -0.1745138560725176813 ) ) ;
#10968=CARTESIAN_POINT ( 'NONE',  ( -12.50000000000000355, 113.9101862821014493, -0.1745138560725492671 ) ) ;
#10982=CARTESIAN_POINT ( 'NONE',  ( 12.53471296425189330, 130.9773137178985678, 2.311890736173451977 ) ) ;
#10983=CARTESIAN_POINT ( 'NONE',  ( -8.715434833791929847, 133.4601862821014606, -8.962234695871762469 ) ) ;
#10989=CARTESIAN_POINT ( 'NONE',  ( -6.092822981423666739, 109.4148137178985536, -14.25334919248795096 ) ) ;
#10996=CARTESIAN_POINT ( 'NONE',  ( -0.1745138560725500443, 111.6101862821014521, 12.50000000000000355 ) ) ;
#11003=CARTESIAN_POINT ( 'NONE',  ( -12.53471296425194836, 122.8226862821014720, 2.311890736173176641 ) ) ;
#11007=CARTESIAN_POINT ( 'NONE',  ( 15.46528703574804986, 100.3976862821014606, 3.257655550457285720 ) ) ;
#11009=CARTESIAN_POINT ( 'NONE',  ( -12.50000000000000355, 12.71018628210143753, -0.1745138560725492671 ) ) ;
#11011=CARTESIAN_POINT ( 'NONE',  ( -7.954856959092191815, 133.1726862821014663, -5.529263428287477744 ) ) ;
#11016=CARTESIAN_POINT ( 'NONE',  ( 8.710071997420127943, 63.88518628210145778, 3.796722387233375073 ) ) ;
#11024=CARTESIAN_POINT ( 'NONE',  ( 8.843639120294245259, 48.46481371789856496, 3.474262827703527901 ) ) ;
#11028=CARTESIAN_POINT ( 'NONE',  ( -10.69584247140429412, 62.55231371789855643, -6.932735513424201024 ) ) ;
#11031=CARTESIAN_POINT ( 'NONE',  ( -12.50000000000000355, 34.08981371789854364, 0.1745138560722786503 ) ) ;
#11035=CARTESIAN_POINT ( 'NONE',  ( -10.49813415415989581, 4.372686282101440725, -7.228626920339068285 ) ) ;
#11046=CARTESIAN_POINT ( 'NONE',  ( 13.04141134922778988, 37.82731371789854080, -8.927990412390371944 ) ) ;
#11049=CARTESIAN_POINT ( 'NONE',  ( -4.622313124798576922, 5.235186282101428112, -11.61527771782819762 ) ) ;
#11050=CARTESIAN_POINT ( 'NONE',  ( -8.962234695871760692, 57.56018628210145494, 8.715434833791933400 ) ) ;
#11051=CARTESIAN_POINT ( 'NONE',  ( 0.1745138560725837118, 5.810186282101448718, -15.50000000000000533 ) ) ;
#11056=CARTESIAN_POINT ( 'NONE',  ( 13.23911966647218996, 7.247686282101430066, -8.632099005475504683 ) ) ;
#11065=CARTESIAN_POINT ( 'NONE',  ( 8.843639120294245259, 112.8648137178985564, 3.474262827703527901 ) ) ;
#11071=CARTESIAN_POINT ( 'NONE',  ( 4.622313124798831829, 110.5648137178985593, -11.61527771782809282 ) ) ;
#11085=CARTESIAN_POINT ( 'NONE',  ( 6.932735513423970097, 55.54768628210144499, 10.69584247140445044 ) ) ;
#11094=CARTESIAN_POINT ( 'NONE',  ( 8.962234695871567070, 113.4398137178985593, 8.715434833792127023 ) ) ;
#11100=CARTESIAN_POINT ( 'NONE',  ( 13.23911966647199812, 103.9523137178985763, 8.632099005475788900 ) ) ;
#11104=CARTESIAN_POINT ( 'NONE',  ( 4.622313124798573369, 120.2351862821014663, 11.61527771782819940 ) ) ;
#11105=CARTESIAN_POINT ( 'NONE',  ( 6.092822981423978490, 70.78518628210143504, -14.25334919248782306 ) ) ;
#11108=CARTESIAN_POINT ( 'NONE',  ( -8.632099005475501130, 78.54768628210145209, -13.23911966647218996 ) ) ;
#11110=CARTESIAN_POINT ( 'NONE',  ( 2.064181346179272847, 24.49768628210144072, -9.465287035748065847 ) ) ;
#11113=CARTESIAN_POINT ( 'NONE',  ( 12.50000000000000355, 54.11018628210144499, 0.1745138560725507937 ) ) ;
#11116=CARTESIAN_POINT ( 'NONE',  ( -9.534712964251941258, 21.62268628210143717, 1.715153634034234154 ) ) ;
#11129=CARTESIAN_POINT ( 'NONE',  ( -8.962234695871760692, 66.76018628210145778, 8.715434833791933400 ) ) ;
#11134=CARTESIAN_POINT ( 'NONE',  ( -8.632099005475794229, 41.85231371789854649, 13.23911966647199812 ) ) ;
#11135=EDGE_CURVE ( 'NONE', #15372, #33833, #6232, .T. ) ;
#11141=CARTESIAN_POINT ( 'NONE',  ( -6.594114490232462877, 32.93981371789854506, 6.840914352311949109 ) ) ;
#11143=CARTESIAN_POINT ( 'NONE',  ( 1.715153634034445762, 91.87731371789854506, -9.534712964251895073 ) ) ;
#11146=CARTESIAN_POINT ( 'NONE',  ( 6.092822981423662299, 141.6148137178985849, 14.25334919248795096 ) ) ;
#11148=CARTESIAN_POINT ( 'NONE',  ( -12.53471296425194836, 67.62268628210145494, 2.311890736173176641 ) ) ;
#11156=CARTESIAN_POINT ( 'NONE',  ( -3.796722387233375073, 84.58518628210146062, 8.710071997420127943 ) ) ;
#11158=CARTESIAN_POINT ( 'NONE',  ( -6.932735513423968321, 106.1476862821014606, -10.69584247140445221 ) ) ;
#11170=CARTESIAN_POINT ( 'NONE',  ( -2.311890736173448424, 124.0773137178985621, 12.53471296425189330 ) ) ;
#11171=CARTESIAN_POINT ( 'NONE',  ( -4.944772684328673229, 139.7851862821014493, 11.48171059495397728 ) ) ;
#11175=CARTESIAN_POINT ( 'NONE',  ( -12.46528703574811558, 15.40231371789854720, 2.660918448318004170 ) ) ;
#11176=CARTESIAN_POINT ( 'NONE',  ( -13.04141134922778456, 97.62731371789854506, 8.927990412390377273 ) ) ;
#11177=CARTESIAN_POINT ( 'NONE',  ( 2.660918448318279950, 98.09768628210146346, -12.46528703574805697 ) ) ;
#11181=CARTESIAN_POINT ( 'NONE',  ( -0.1745138560725500443, 120.8101862821014691, 12.50000000000000355 ) ) ;
#11186=CARTESIAN_POINT ( 'NONE',  ( 2.311890736173175753, 120.5226862821014606, 12.53471296425194836 ) ) ;
#11191=CARTESIAN_POINT ( 'NONE',  ( -15.50000000000000533, 104.7101862821014606, -0.1745138560725808530 ) ) ;
#11192=CARTESIAN_POINT ( 'NONE',  ( -10.69584247140444866, 11.84768628210144925, 6.932735513423972762 ) ) ;
#11195=CARTESIAN_POINT ( 'NONE',  ( -6.594114490232312775, 133.4601862821014606, -6.840914352312096547 ) ) ;
#11201=CARTESIAN_POINT ( 'NONE',  ( 9.534712964251941258, 63.02268628210144641, -1.715153634034235708 ) ) ;
#11208=CARTESIAN_POINT ( 'NONE',  ( -3.474262827703527901, 32.36481371789854933, 8.843639120294245259 ) ) ;
#11213=CARTESIAN_POINT ( 'NONE',  ( 6.932735513424201024, 55.65231371789855785, -10.69584247140429412 ) ) ;
#11216=CARTESIAN_POINT ( 'NONE',  ( 10.69584247140429589, 21.15231371789855430, 6.932735513424201024 ) ) ;
#11220=CARTESIAN_POINT ( 'NONE',  ( 8.962234695871762469, 6.960186282101432198, -8.715434833791931624 ) ) ;
#11233=CARTESIAN_POINT ( 'NONE',  ( 6.092822981423662299, 22.01481371789855501, 14.25334919248795096 ) ) ;
#11235=CARTESIAN_POINT ( 'NONE',  ( 4.622313124798573369, 9.835186282101449962, 11.61527771782819940 ) ) ;
#11236=CARTESIAN_POINT ( 'NONE',  ( -2.660918448318275509, 56.69768628210145067, 12.46528703574805874 ) ) ;
#11240=CARTESIAN_POINT ( 'NONE',  ( 15.50000000000000533, 17.31018628210144428, 0.1745138560725827404 ) ) ;
#11251=CARTESIAN_POINT ( 'NONE',  ( -2.064181346179062349, 118.9023137178985650, -9.465287035748106703 ) ) ;
#11258=CARTESIAN_POINT ( 'NONE',  ( 8.962234695871567070, 122.6398137178985621, 8.715434833792127023 ) ) ;
#11259=ADVANCED_FACE ( 'NONE', ( #4895 ), #16850, .T. ) ;
#11275=CARTESIAN_POINT ( 'NONE',  ( -11.61527771782819940, 67.33518628210144641, 4.622313124798574258 ) ) ;
#11280=CARTESIAN_POINT ( 'NONE',  ( -11.48171059495408208, 97.91481371789856780, 4.944772684328421875 ) ) ;
#11287=CARTESIAN_POINT ( 'NONE',  ( -14.25334919248795096, 79.51481371789856212, 6.092822981423662299 ) ) ;
#11291=CARTESIAN_POINT ( 'NONE',  ( -7.228626920339069173, 112.4726862821014493, 10.49813415415989581 ) ) ;
#11292=CARTESIAN_POINT ( 'NONE',  ( -3.257655550457281723, 65.89768628210143220, 15.46528703574804986 ) ) ;
#11295=CARTESIAN_POINT ( 'NONE',  ( 11.08355503943142750, 62.16018628210144925, -10.83675517735155225 ) ) ;
#11301=CARTESIAN_POINT ( 'NONE',  ( -12.50000000000000355, 31.11018628210143788, -0.1745138560725492671 ) ) ;
#11304=CARTESIAN_POINT ( 'NONE',  ( -0.1745138560725182642, 19.61018628210144144, 9.500000000000005329 ) ) ;
#11314=CARTESIAN_POINT ( 'NONE',  ( -6.932735513423968321, 69.34768628210144925, -10.69584247140445221 ) ) ;
#11320=CARTESIAN_POINT ( 'NONE',  ( 15.50000000000000533, 38.68981371789855217, -0.1745138560722452326 ) ) ;
#11327=CARTESIAN_POINT ( 'NONE',  ( -8.152565276336593669, 16.55231371789855643, -5.233372021372610483 ) ) ;
#11332=CARTESIAN_POINT ( 'NONE',  ( 10.69584247140429589, 11.95231371789853902, 6.932735513424201024 ) ) ;
#11335=CARTESIAN_POINT ( 'NONE',  ( 4.944772684328679446, 61.58518628210145351, -11.48171059495397373 ) ) ;
#11342=CARTESIAN_POINT ( 'NONE',  ( -9.465287035748065847, 77.39768628210144641, -2.064181346179273735 ) ) ;
#11345=CARTESIAN_POINT ( 'NONE',  ( 6.932735513423970097, 119.9476862821014578, 10.69584247140445044 ) ) ;
#11358=CARTESIAN_POINT ( 'NONE',  ( -4.944772684328424539, 127.8148137178985735, -11.48171059495408031 ) ) ;
#11359=CARTESIAN_POINT ( 'NONE',  ( 10.49813415415989581, 128.5726862821014720, 7.228626920339069173 ) ) ;
#11365=CARTESIAN_POINT ( 'NONE',  ( 10.83675517735179206, 92.73981371789854222, -11.08355503943118769 ) ) ;
#11366=CARTESIAN_POINT ( 'NONE',  ( 7.228626920339068285, 89.47268628210144925, -10.49813415415989581 ) ) ;
#11369=CARTESIAN_POINT ( 'NONE',  ( -4.944772684328673229, 112.1851862821014549, 11.48171059495397728 ) ) ;
#11374=CARTESIAN_POINT ( 'NONE',  ( -7.228626920339069173, 112.4726862821014493, 10.49813415415989581 ) ) ;
#11379=CARTESIAN_POINT ( 'NONE',  ( -13.04141134922759804, 105.5726862821014294, -8.927990412390657937 ) ) ;
#11380=CARTESIAN_POINT ( 'NONE',  ( 12.53471296425194659, 17.02268628210144996, -2.311890736173178418 ) ) ;
#11383=CARTESIAN_POINT ( 'NONE',  ( 3.474262827703335166, 138.6351862821014720, 8.843639120294326972 ) ) ;
#11387=CARTESIAN_POINT ( 'NONE',  ( 5.233372021372432847, 64.74768628210144072, 8.152565276336710909 ) ) ;
#11395=CARTESIAN_POINT ( 'NONE',  ( 5.529263428287300108, 30.92731371789853867, 7.954856959092309943 ) ) ;
#11401=CARTESIAN_POINT ( 'NONE',  ( 8.715434833792128799, 37.53981371789855359, -8.962234695871567070 ) ) ;
#11404=CARTESIAN_POINT ( 'NONE',  ( 6.932735513424201024, 18.85231371789855714, -10.69584247140429412 ) ) ;
#11422=CARTESIAN_POINT ( 'NONE',  ( 0.1745138560722461762, 13.38981371789854613, 15.50000000000000533 ) ) ;
#11424=CARTESIAN_POINT ( 'NONE',  ( -2.660918448318275509, 10.69768628210143646, 12.46528703574805874 ) ) ;
#11425=CARTESIAN_POINT ( 'NONE',  ( 10.69584247140445221, 53.24768628210144072, -6.932735513423970097 ) ) ;
#11436=CARTESIAN_POINT ( 'NONE',  ( 5.233372021372610483, 92.45231371789854791, -8.152565276336593669 ) ) ;
#11443=CARTESIAN_POINT ( 'NONE',  ( -4.944772684328424539, 109.4148137178985536, -11.48171059495408031 ) ) ;
#11447=CARTESIAN_POINT ( 'NONE',  ( 11.61527771782809637, 57.66481371789855359, 4.622313124798827388 ) ) ;
#11456=CARTESIAN_POINT ( 'NONE',  ( 10.49813415415989581, 54.97268628210144925, 7.228626920339068285 ) ) ;
#11463=CARTESIAN_POINT ( 'NONE',  ( -4.622313124798826500, 105.9648137178985650, 11.61527771782809637 ) ) ;
#11468=CARTESIAN_POINT ( 'NONE',  ( 15.50000000000000533, 75.48981371789854222, -0.1745138560722452326 ) ) ;
#11472=CARTESIAN_POINT ( 'NONE',  ( -2.660918448318275509, 111.8976862821014606, 12.46528703574805874 ) ) ;
#11473=CARTESIAN_POINT ( 'NONE',  ( -0.1745138560725817967, 47.21018628210144641, 15.50000000000000533 ) ) ;
#11476=CARTESIAN_POINT ( 'NONE',  ( -15.46528703574804986, 58.99768628210144783, -3.257655550457287497 ) ) ;
#11483=CARTESIAN_POINT ( 'NONE',  ( -10.69584247140444866, 48.64768628210144641, 6.932735513423972762 ) ) ;
#11486=CARTESIAN_POINT ( 'NONE',  ( 8.843639120294328748, 16.73518628210143788, -3.474262827703334722 ) ) ;
#11496=CARTESIAN_POINT ( 'NONE',  ( 10.49813415415989581, 64.17268628210145209, 7.228626920339069173 ) ) ;
#11503=CARTESIAN_POINT ( 'NONE',  ( -14.38691631536193860, 34.66481371789854649, -5.770363421894132649 ) ) ;
#11509=CARTESIAN_POINT ( 'NONE',  ( -9.465287035748106703, 24.60231371789854649, 2.064181346179061460 ) ) ;
#11514=CARTESIAN_POINT ( 'NONE',  ( 0.1745138560722461762, 123.7898137178985678, 15.50000000000000533 ) ) ;
#11517=CARTESIAN_POINT ( 'NONE',  ( 8.715434833791931624, 36.86018628210144499, 8.962234695871760692 ) ) ;
#11525=CARTESIAN_POINT ( 'NONE',  ( 1.715153634034233487, 83.72268628210143504, 9.534712964251941258 ) ) ;
#11528=CARTESIAN_POINT ( 'NONE',  ( 4.622313124798573369, 92.63518628210145778, 11.61527771782819940 ) ) ;
#11539=CARTESIAN_POINT ( 'NONE',  ( 12.46528703574811558, 121.2023137178985621, -2.660918448318005503 ) ) ;
#11540=CARTESIAN_POINT ( 'NONE',  ( 12.46528703574805874, 127.9976862821014549, 2.660918448318279950 ) ) ;
#11546=CARTESIAN_POINT ( 'NONE',  ( -0.1745138560722442889, 100.7898137178985536, -15.50000000000000533 ) ) ;
#11550=CARTESIAN_POINT ( 'NONE',  ( 0.1745138560723095977, 77.78981371789853938, 9.500000000000005329 ) ) ;
#11554=CARTESIAN_POINT ( 'NONE',  ( -8.715434833792127023, 42.13981371789854791, 8.962234695871568846 ) ) ;
#11556=CARTESIAN_POINT ( 'NONE',  ( -10.49813415415989581, 96.37268628210145494, -7.228626920339068285 ) ) ;
#11563=CARTESIAN_POINT ( 'NONE',  ( 13.23911966647218996, 108.4476862821014294, -8.632099005475504683 ) ) ;
#11564=CARTESIAN_POINT ( 'NONE',  ( 10.49813415415989581, 8.972686282101433264, 7.228626920339069173 ) ) ;
#11567=CARTESIAN_POINT ( 'NONE',  ( 9.500000000000005329, 127.7101862821014606, 0.1745138560725188748 ) ) ;
#11571=CARTESIAN_POINT ( 'NONE',  ( -5.233372021372430183, 69.34768628210143504, -8.152565276336710909 ) ) ;
#11578=CARTESIAN_POINT ( 'NONE',  ( -5.233372021372612259, 32.65231371789855075, 8.152565276336593669 ) ) ;
#11583=CARTESIAN_POINT ( 'NONE',  ( -12.50000000000000355, 52.48981371789855643, 0.1745138560722786503 ) ) ;
#11586=CARTESIAN_POINT ( 'NONE',  ( 14.38691631536194393, 140.4648137178985507, 5.770363421894124656 ) ) ;
#11601=CARTESIAN_POINT ( 'NONE',  ( 15.50000000000000533, 29.48981371789855288, -0.1745138560722452326 ) ) ;
#11603=CARTESIAN_POINT ( 'NONE',  ( 12.53471296425194836, 7.822686282101448896, -2.311890736173178418 ) ) ;
#11604=CARTESIAN_POINT ( 'NONE',  ( -11.61527771782819940, 48.93518628210144783, 4.622313124798574258 ) ) ;
#11616=CARTESIAN_POINT ( 'NONE',  ( -3.474262827703527901, 96.76481371789854791, 8.843639120294245259 ) ) ;
#11623=CARTESIAN_POINT ( 'NONE',  ( 8.962234695871567070, 95.03981371789856780, 8.715434833792127023 ) ) ;
#11627=CARTESIAN_POINT ( 'NONE',  ( -2.660918448318004614, 63.70231371789855501, -12.46528703574811558 ) ) ;
#11636=CARTESIAN_POINT ( 'NONE',  ( 8.715434833791931624, 46.06018628210144072, 8.962234695871760692 ) ) ;
#11641=CARTESIAN_POINT ( 'NONE',  ( -2.311890736173448424, 105.6773137178985564, 12.53471296425189330 ) ) ;
#11646=CARTESIAN_POINT ( 'NONE',  ( -13.04141134922778456, 79.22731371789853938, 8.927990412390377273 ) ) ;
#11650=CARTESIAN_POINT ( 'NONE',  ( 12.46528703574805874, 109.5976862821014493, 2.660918448318279950 ) ) ;
#11651=CARTESIAN_POINT ( 'NONE',  ( -3.257655550457281723, 47.49768628210145494, 15.46528703574804986 ) ) ;
#11654=CARTESIAN_POINT ( 'NONE',  ( -2.908627838312119351, 69.92268628210143788, -15.53471296425195369 ) ) ;
#11662=CARTESIAN_POINT ( 'NONE',  ( -4.622313124798576922, 42.03518628210144215, -11.61527771782819762 ) ) ;
#11665=CARTESIAN_POINT ( 'NONE',  ( -9.534712964251941258, 12.42268628210144144, 1.715153634034234154 ) ) ;
#11678=CARTESIAN_POINT ( 'NONE',  ( -0.1745138560725500443, 65.61018628210145209, 12.50000000000000355 ) ) ;
#11685=CARTESIAN_POINT ( 'NONE',  ( -3.257655550456946880, 36.10231371789854649, -15.46528703574811736 ) ) ;
#11692=CARTESIAN_POINT ( 'NONE',  ( 0.1745138560723095977, 22.58981371789854364, 9.500000000000005329 ) ) ;
#11697=CARTESIAN_POINT ( 'NONE',  ( 14.38691631536194393, 131.2648137178985621, 5.770363421894124656 ) ) ;
#11700=CARTESIAN_POINT ( 'NONE',  ( 11.48171059495397728, 54.68518628210144783, 4.944772684328674117 ) ) ;
#11707=CARTESIAN_POINT ( 'NONE',  ( 3.474262827703335166, 55.83518628210145351, 8.843639120294326972 ) ) ;
#11710=CARTESIAN_POINT ( 'NONE',  ( 12.53471296425194836, 99.82268628210144357, -2.311890736173178418 ) ) ;
#11725=CARTESIAN_POINT ( 'NONE',  ( 2.311890736173452865, 128.6773137178985564, -12.53471296425189152 ) ) ;
#11726=CARTESIAN_POINT ( 'NONE',  ( 2.311890736173175753, 120.5226862821014606, 12.53471296425194659 ) ) ;
#11732=CARTESIAN_POINT ( 'NONE',  ( -13.04141134922778456, 88.42731371789855643, 8.927990412390377273 ) ) ;
#11738=CARTESIAN_POINT ( 'NONE',  ( 6.594114490232462877, 83.53981371789856780, -6.840914352311949109 ) ) ;
#11742=CARTESIAN_POINT ( 'NONE',  ( 11.48171059495408208, 56.51481371789855501, -4.944772684328420986 ) ) ;
#11744=CARTESIAN_POINT ( 'NONE',  ( -12.46528703574805697, 95.79768628210143788, -2.660918448318280838 ) ) ;
#11747=CARTESIAN_POINT ( 'NONE',  ( -10.69584247140444866, 140.6476862821014890, 6.932735513423972762 ) ) ;
#11749=CARTESIAN_POINT ( 'NONE',  ( 15.46528703574804986, 109.5976862821014493, 3.257655550457285720 ) ) ;
#11750=CARTESIAN_POINT ( 'NONE',  ( 0.1745138560725515708, 15.01018628210143468, -12.50000000000000355 ) ) ;
#11753=CARTESIAN_POINT ( 'NONE',  ( 1.715153634034233487, 129.7226862821014208, 9.534712964251941258 ) ) ;
#11759=CARTESIAN_POINT ( 'NONE',  ( -7.954856959092191815, 59.57268628210145067, -5.529263428287477744 ) ) ;
#11768=CARTESIAN_POINT ( 'NONE',  ( -1.715153634034442431, 41.27731371789855075, 9.534712964251900402 ) ) ;
#11773=CARTESIAN_POINT ( 'NONE',  ( 12.53471296425189330, 38.97731371789854649, 2.311890736173451533 ) ) ;
#11776=CARTESIAN_POINT ( 'NONE',  ( 10.69584247140429589, 11.95231371789853902, 6.932735513424201024 ) ) ;
#11789=CARTESIAN_POINT ( 'NONE',  ( -14.38691631536193860, 16.26481371789853370, -5.770363421894132649 ) ) ;
#11791=CARTESIAN_POINT ( 'NONE',  ( -8.715434833791929847, 13.86018628210145032, -8.962234695871762469 ) ) ;
#11793=CARTESIAN_POINT ( 'NONE',  ( -7.228626920339069173, 57.27268628210144641, 10.49813415415989581 ) ) ;
#11798=CARTESIAN_POINT ( 'NONE',  ( 6.594114490232313663, 18.46018628210144286, 6.840914352312096547 ) ) ;
#11805=CARTESIAN_POINT ( 'NONE',  ( 5.529263428287300108, 95.32731371789854791, 7.954856959092309943 ) ) ;
#11810=CARTESIAN_POINT ( 'NONE',  ( -12.46528703574811558, 98.20231371789856212, 2.660918448318004170 ) ) ;
#11814=CARTESIAN_POINT ( 'NONE',  ( 4.944772684328420986, 68.01481371789854791, 11.48171059495408208 ) ) ;
#11823=CARTESIAN_POINT ( 'NONE',  ( -6.932735513423968321, 32.54768628210144499, -10.69584247140445221 ) ) ;
#11828=CARTESIAN_POINT ( 'NONE',  ( 10.69584247140429589, 94.75231371789854506, 6.932735513424201024 ) ) ;
#11833=CARTESIAN_POINT ( 'NONE',  ( 14.38691631536194393, 76.06481371789855928, 5.770363421894124656 ) ) ;
#11838=CARTESIAN_POINT ( 'NONE',  ( 8.715434833791931624, 101.2601862821014578, 8.962234695871760692 ) ) ;
#11839=CARTESIAN_POINT ( 'NONE',  ( 8.927990412390657937, 52.67268628210144499, -13.04141134922759804 ) ) ;
#11843=CARTESIAN_POINT ( 'NONE',  ( -6.092822981423970496, 66.18518628210145494, 14.25334919248782661 ) ) ;
#11849=CARTESIAN_POINT ( 'NONE',  ( 4.944772684328679446, 43.18518628210144072, -11.48171059495397373 ) ) ;
#11852=CARTESIAN_POINT ( 'NONE',  ( -2.064181346179269738, 10.69768628210143646, 9.465287035748067623 ) ) ;
#11862=CARTESIAN_POINT ( 'NONE',  ( -2.660918448318275509, 65.89768628210146062, 12.46528703574805874 ) ) ;
#11869=CARTESIAN_POINT ( 'NONE',  ( -3.257655550456946880, 45.30231371789854933, -15.46528703574811736 ) ) ;
#11876=CARTESIAN_POINT ( 'NONE',  ( 9.465287035748106703, 20.00231371789855217, -2.064181346179063237 ) ) ;
#11883=CARTESIAN_POINT ( 'NONE',  ( -15.50000000000000533, 126.0898137178985650, 0.1745138560722471477 ) ) ;
#11886=CARTESIAN_POINT ( 'NONE',  ( 2.660918448318279950, 52.09768628210144215, -12.46528703574805697 ) ) ;
#11894=CARTESIAN_POINT ( 'NONE',  ( 9.534712964251941258, 63.02268628210144641, -1.715153634034235708 ) ) ;
#11898=CARTESIAN_POINT ( 'NONE',  ( 2.311890736173175753, 92.92268628210145209, 12.53471296425194836 ) ) ;
#11900=B_SPLINE_CURVE_WITH_KNOTS ( 'NONE', 3,
 ( #33164, #10414, #27664, #21801, #33353, #4903, #16297, #12694, #7762, #30700, #24266, #15735, #18962, #27285, #27845, #35810, #36554, #19342, #30516, #1316 ),
 .UNSPECIFIED., .F., .F.,
 ( 4, 2, 2, 2, 2, 2, 2, 2, 2, 4 ),
 ( 0.000000000000000000, 0.002984115787595702056, 0.005968231575191402377, 0.008952347362787101831, 0.01044440525658495156, 0.01119043420348387642, 0.01156344867693333799, 0.01174995591365806703, 0.01184320953202043329, 0.01193646315038279955 ),
 .UNSPECIFIED. ) ;
#11911=CARTESIAN_POINT ( 'NONE',  ( 4.622313124798831829, 119.7648137178985763, -11.61527771782809282 ) ) ;
#11912=CARTESIAN_POINT ( 'NONE',  ( -4.622313124798576922, 115.6351862821014578, -11.61527771782819762 ) ) ;
#11918=CARTESIAN_POINT ( 'NONE',  ( 8.927990412390371944, 86.12731371789853085, 13.04141134922778811 ) ) ;
#11922=CARTESIAN_POINT ( 'NONE',  ( 6.840914352311949109, 76.63981371789854791, 6.594114490232462877 ) ) ;
#11926=CARTESIAN_POINT ( 'NONE',  ( 8.962234695871567070, 49.03981371789854649, 8.715434833792127023 ) ) ;
#11927=CARTESIAN_POINT ( 'NONE',  ( -8.962234695871760692, 103.5601862821014549, 8.715434833791933400 ) ) ;
#11932=CARTESIAN_POINT ( 'NONE',  ( 8.927990412390657937, 89.47268628210143504, -13.04141134922759804 ) ) ;
#11934=CARTESIAN_POINT ( 'NONE',  ( -12.50000000000000355, 3.510186282101451560, -0.1745138560725492671 ) ) ;
#11938=CARTESIAN_POINT ( 'NONE',  ( -3.796722387233375073, 121.3851862821014578, 8.710071997420127943 ) ) ;
#11941=CARTESIAN_POINT ( 'NONE',  ( 10.83675517735155225, 9.260186282101427580, 11.08355503943142573 ) ) ;
#11946=CARTESIAN_POINT ( 'NONE',  ( -5.529263428287477744, 48.07268628210143646, 7.954856959092191815 ) ) ;
#11953=CARTESIAN_POINT ( 'NONE',  ( -9.500000000000005329, 43.28981371789856070, 0.1745138560723101806 ) ) ;
#11957=CARTESIAN_POINT ( 'NONE',  ( 8.715434833792128799, 46.73981371789854933, -8.962234695871567070 ) ) ;
#11959=CARTESIAN_POINT ( 'NONE',  ( 12.50000000000000355, 11.08981371789855075, -0.1745138560722771515 ) ) ;
#11974=CARTESIAN_POINT ( 'NONE',  ( -2.908627838312453306, 13.67731371789853867, 15.53471296425188797 ) ) ;
#11978=CARTESIAN_POINT ( 'NONE',  ( 8.843639120294328748, 127.1351862821014720, -3.474262827703334722 ) ) ;
#11979=CARTESIAN_POINT ( 'NONE',  ( 2.660918448318279950, 33.69768628210145067, -12.46528703574805697 ) ) ;
#11985=CARTESIAN_POINT ( 'NONE',  ( -2.064181346179269738, 29.09768628210144925, 9.465287035748067623 ) ) ;
#11992=CARTESIAN_POINT ( 'NONE',  ( 3.796722387233182339, 86.41481371789855359, 8.710071997420207879 ) ) ;
#11998=CARTESIAN_POINT ( 'NONE',  ( 2.311890736173452421, 101.0773137178985621, -12.53471296425189152 ) ) ;
#12002=CARTESIAN_POINT ( 'NONE',  ( -10.49813415416004858, 70.02731371789855075, 7.228626920338839135 ) ) ;
#12009=CARTESIAN_POINT ( 'NONE',  ( -6.932735513423968321, 41.74768628210144783, -10.69584247140445221 ) ) ;
#12016=CARTESIAN_POINT ( 'NONE',  ( 7.228626920338837358, 104.5273137178985650, 10.49813415416005036 ) ) ;
#12023=CARTESIAN_POINT ( 'NONE',  ( -15.50000000000000533, 80.08981371789856496, 0.1745138560722471477 ) ) ;
#12027=CARTESIAN_POINT ( 'NONE',  ( -10.49813415415989581, 96.37268628210145494, -7.228626920339068285 ) ) ;
#12028=CARTESIAN_POINT ( 'NONE',  ( -8.632099005475501130, 41.74768628210143362, -13.23911966647218996 ) ) ;
#12031=CARTESIAN_POINT ( 'NONE',  ( -0.1745138560725817967, 65.61018628210146630, 15.50000000000000533 ) ) ;
#12037=CARTESIAN_POINT ( 'NONE',  ( 12.50000000000000355, 35.71018628210144641, 0.1745138560725507937 ) ) ;
#12039=CARTESIAN_POINT ( 'NONE',  ( 5.529263428287477744, 15.87268628210144605, -7.954856959092191815 ) ) ;
#12049=CARTESIAN_POINT ( 'NONE',  ( -6.932735513423968321, 41.74768628210144783, -10.69584247140445221 ) ) ;
#12056=CARTESIAN_POINT ( 'NONE',  ( -10.49813415415989581, 96.37268628210145494, -7.228626920339068285 ) ) ;
#12057=CARTESIAN_POINT ( 'NONE',  ( 14.38691631536194393, 20.86481371789854578, 5.770363421894124656 ) ) ;
#12063=CARTESIAN_POINT ( 'NONE',  ( -6.594114490232462877, 14.53981371789855892, 6.840914352311949109 ) ) ;
#12069=CARTESIAN_POINT ( 'NONE',  ( -13.04141134922778456, 125.2273137178985394, 8.927990412390377273 ) ) ;
#12072=CARTESIAN_POINT ( 'NONE',  ( 12.53471296425194836, 44.62268628210144783, -2.311890736173178418 ) ) ;
#12079=CARTESIAN_POINT ( 'NONE',  ( 8.710071997420127943, 63.88518628210145778, 3.796722387233375073 ) ) ;
#12082=CARTESIAN_POINT ( 'NONE',  ( -10.69584247140444866, 103.8476862821014493, 6.932735513423972762 ) ) ;
#12094=CARTESIAN_POINT ( 'NONE',  ( -11.48171059495408208, 97.91481371789856780, 4.944772684328421875 ) ) ;
#12095=CARTESIAN_POINT ( 'NONE',  ( -12.50000000000000355, 132.3101862821014549, -0.1745138560725492671 ) ) ;
#12100=CARTESIAN_POINT ( 'NONE',  ( -14.25334919248795096, 79.51481371789856212, 6.092822981423662299 ) ) ;
#12104=CARTESIAN_POINT ( 'NONE',  ( 2.064181346179272847, 98.09768628210146346, -9.465287035748065847 ) ) ;
#12106=CARTESIAN_POINT ( 'NONE',  ( -7.954856959092309943, 79.22731371789853938, 5.529263428287300108 ) ) ;
#12109=CARTESIAN_POINT ( 'NONE',  ( 8.962234695871567070, 39.83981371789855075, 8.715434833792127023 ) ) ;
#12112=CARTESIAN_POINT ( 'NONE',  ( 12.46528703574805874, 109.5976862821014493, 2.660918448318279950 ) ) ;
#12117=CARTESIAN_POINT ( 'NONE',  ( -0.1745138560725817967, 74.81018628210145494, 15.50000000000000533 ) ) ;
#12122=CARTESIAN_POINT ( 'NONE',  ( -0.1745138560725182642, 120.8101862821014691, 9.500000000000005329 ) ) ;
#12124=CARTESIAN_POINT ( 'NONE',  ( -0.1745138560725817967, 10.41018628210144037, 15.50000000000000533 ) ) ;
#12136=CARTESIAN_POINT ( 'NONE',  ( 5.233372021372610483, 18.85231371789855359, -8.152565276336593669 ) ) ;
#12140=CARTESIAN_POINT ( 'NONE',  ( -8.962234695871565293, 44.43981371789855217, -8.715434833792128799 ) ) ;
#12142=CARTESIAN_POINT ( 'NONE',  ( -10.69584247140429412, 7.352313717898545598, -6.932735513424201024 ) ) ;
#12143=( BOUNDED_CURVE ( )  B_SPLINE_CURVE ( 2, ( #1792, #4633, #7304, #33445, #10507, #7488, #1414, #13359, #16212, #4447, #27761, #1040, #24729, #16027, #18876, #21532, #35722, #24914, #27576, #33079, #12796, #21346, #1605, #10327, #12992, #30427, #22087, #13173, #21897, #9768, #33637, #15461, #18312, #29852, #3889, #1224, #27015, #21714, #12611, #30044, #4261, #24177, #32885, #6934, #4078, #15650, #27198, #36097, #24365, #35909, #9952, #7122, #18694, #30235, #15836, #27384, #24547, #10141, #34191, #36841, #10696, #16399, #8049, #10884, #5374, #22273, #7676, #33826, #16768, #8238, #25658, #19813, #11258, #28496, #7863, #5004, #5193, #30987, #17142, #25100, #22646, #4818, #31347, #34004, #2352, #22457, #16586, #16953, #2539, #14106, #25844, #37212, #19437, #13924, #22830, #28131, #27944, #37393, #2160, #1975, #37025, #13743, #36658, #34378, #8419, #13547, #25289, #31171, #19624, #19988, #28314, #31532, #5557, #25474, #11071, #28678, #2716, #14292, #11443, #23010, #19256, #30795, #31904, #6505, #17888, #23569, #26210, #56, #8599, #246, #18080, #615, #8974, #17325, #26776, #26400, #14475, #29621, #3656, #3091, #14659, #34746, #5933, #32088, #20361, #15227, #26028, #11998, #35114, #35296, #3469, #28868, #20545, #17512, #29047, #8789, #5745, #11810, #20170, #32273, #23380, #9162, #23198, #31718, #807, #34929, #2902, #433, #11623, #12378, #34560, #6120, #17698, #29238, #3278, #14851, #20730, #6316, #29433, #15038, #26586, #12184, #23757, #9352, #20923, #32462, #30192, #12947, #35867, #6694, #32840, #6885, #15987, #24686, #36056, #30383, #4594, #36240, #13132, #23948, #24508, #21114, #18460, #29809, #30003, #1560, #32653, #19021, #21304, #10282, #7083, #18651, #27535, #26966, #10099, #4404, #4218, #21669, #21856, #33223, #33409, #15796, #7262, #18837, #4032, #7447, #35680, #30578, #27346, #21493, #1377, #18265, #9732, #9909, #995, #16171, #15604, #27721, #1750, #3842, #12571, #27160, #1183, #35490, #15420, #9540, #12757, #24138, #24325, #33033, #34148, #2310, #4960, #16353, #24875, #16542, #22785, #16914, #25248, #33596, #5514, #22416, #13884, #31308, #25433, #28455, #8195, #13501, #10653, #10842, #36612, #34334, #30758, #28274, #36985, #14066, #19771, #7635, #36798, #22232, #7821, #11028, #22603, #31491, #5336, #25059, #8005, #2491, #1933, #10467, #17099, #33783, #22045, #5147, #19212, #28638, #8379, #19398, #33963, #28088, #30941, #25615, #2120, #37172, #4780, #11213, #19950, #13697, #19578, #31130, #27902, #16728, #13317, #36424, #14619, #22972, #11583, #23158, #32234, #3425, #14810, #17850, #32421, #29388, #23339, #23715, #26544, #26355, #14993, #34520, #9122, #391, #3237, #5893, #20127, #573, #11957, #17471, #34700, #2676, #35073, #20688, #34890, #23527, #12140, #6273, #35256, #31674, #9311, #37349, #20882, #6465, #8930, #6075, #2859, #5703, #17283, #18036, #14251, #8560, #28824, #20507, #25987, #11773, #14433, #32044, #29006, #25800, #11401, #17, #8747, #20318, #31859, #3050, #26171, #17660, #207, #29195, #21816, #13091, #30339, #36015, #10240, #4363, #18798, #29580, #18608, #15943, #26731, #24092, #35449, #954, #7225, #765, #24646, #26924, #27495, #12711, #24282, #21630, #32612, #4180, #18226, #12333, #15752, #1517, #15562, #27302, #9867, #12904, #1334, #12529, #24468, #35827, #32988, #10054, #27119, #33181, #36196, #21448, #3618, #35637, #33368, #7405, #23907, #29766, #3797, #30152, #9684, #15184, #15375, #9497, #21073, #1142, #6650, #21261, #32800, #6836, #18414, #7041, #29960, #3988, #22559, #30899, #1705, #11175, #10803, #36383, #28412, #25575, #25016, #36571, #22376, #22749, #33924, #31270, #19540, #8158, #28237, #19358, #16129, #25392, #13277, #4920, #4738, #13464, #30718, #27679, #19170, #4554, #16690, #7780, #5111, #10613, #31087, #19732, #16501 ),
 .UNSPECIFIED., .F., .F. ) 
 B_SPLINE_CURVE_WITH_KNOTS ( ( 3, 2, 2, 2, 2, 2, 2, 2, 2, 2, 2, 2, 2, 2, 2, 2, 2, 2, 2, 2, 2, 2, 2, 2, 2, 2, 2, 2, 2, 2, 2, 2, 2, 2, 2, 2, 2, 2, 2, 2, 2, 2, 2, 2, 2, 2, 2, 2, 2, 2, 2, 2, 2, 2, 2, 2, 2, 2, 2, 2, 2, 2, 2, 2, 2, 2, 2, 2, 2, 2, 2, 2, 2, 2, 2, 2, 2, 2, 2, 2, 2, 2, 2, 2, 2, 2, 2, 2, 2, 2, 2, 2, 2, 2, 2, 2, 2, 2, 2, 2, 2, 2, 2, 2, 2, 2, 2, 2, 2, 2, 2, 2, 2, 2, 2, 2, 2, 2, 2, 2, 2, 2, 2, 2, 2, 2, 2, 2, 2, 2, 2, 2, 2, 2, 2, 2, 2, 2, 2, 2, 2, 2, 2, 2, 2, 2, 2, 2, 2, 2, 2, 2, 2, 2, 2, 2, 2, 2, 2, 2, 2, 2, 2, 2, 2, 2, 2, 2, 2, 2, 2, 2, 2, 2, 2, 2, 2, 2, 2, 2, 2, 2, 2, 2, 2, 2, 2, 2, 2, 2, 2, 2, 2, 2, 2, 2, 2, 2, 2, 2, 2, 2, 2, 2, 2, 2, 2, 2, 2, 2, 2, 2, 2, 2, 2, 2, 2, 2, 2, 2, 2, 2, 2, 2, 2, 2, 2, 2, 2, 2, 2, 2, 2, 2, 2, 2, 2, 2, 3 ),
 ( 0.01079222792828509608, 0.01250000000000000069, 0.01666666666666666644, 0.02083333333333333218, 0.02500000000000000139, 0.02916666666666666713, 0.03333333333333333287, 0.03749999999999999861, 0.04166666666666666435, 0.04583333333333333010, 0.05000000000000000278, 0.05416666666666666852, 0.05833333333333333426, 0.06250000000000000000, 0.06666666666666666574, 0.07083333333333333148, 0.07500000000000001110, 0.07916666666666666297, 0.08333333333333334259, 0.08749999999999999445, 0.09166666666666667407, 0.09583333333333335369, 0.1000000000000000056, 0.1041666666666666852, 0.1083333333333333370, 0.1125000000000000167, 0.1166666666666666685, 0.1208333333333333481, 0.1250000000000000000, 0.1291666666666666796, 0.1333333333333333315, 0.1375000000000000111, 0.1416666666666666630, 0.1458333333333333426, 0.1499999999999999944, 0.1541666666666666741, 0.1583333333333333259, 0.1625000000000000056, 0.1666666666666666574, 0.1708333333333333370, 0.1749999999999999889, 0.1791666666666666685, 0.1833333333333333204, 0.1875000000000000000, 0.1916666666666666796, 0.1958333333333333315, 0.2000000000000000111, 0.2041666666666666630, 0.2083333333333333426, 0.2124999999999999944, 0.2166666666666666741, 0.2208333333333333259, 0.2250000000000000056, 0.2291666666666666574, 0.2333333333333333370, 0.2374999999999999889, 0.2416666666666666685, 0.2458333333333333204, 0.2500000000000000000, 0.2541666666666666519, 0.2583333333333333592, 0.2625000000000000111, 0.2666666666666666630, 0.2708333333333333148, 0.2750000000000000222, 0.2791666666666666741, 0.2833333333333333259, 0.2874999999999999778, 0.2916666666666666852, 0.2958333333333333370, 0.2999999999999999889, 0.3041666666666666408, 0.3083333333333333481, 0.3125000000000000000, 0.3166666666666666519, 0.3208333333333333592, 0.3250000000000000111, 0.3291666666666666630, 0.3333333333333333148, 0.3375000000000000222, 0.3416666666666666741, 0.3458333333333333259, 0.3499999999999999778, 0.3541666666666666852, 0.3583333333333333370, 0.3624999999999999889, 0.3666666666666666408, 0.3708333333333333481, 0.3750000000000000000, 0.3791666666666666519, 0.3833333333333333592, 0.3875000000000000111, 0.3916666666666666630, 0.3958333333333333148, 0.4000000000000000222, 0.4041666666666666741, 0.4083333333333333259, 0.4124999999999999778, 0.4166666666666666852, 0.4208333333333333370, 0.4249999999999999889, 0.4291666666666666408, 0.4333333333333333481, 0.4375000000000000000, 0.4416666666666666519, 0.4458333333333333592, 0.4500000000000000111, 0.4541666666666666630, 0.4583333333333333148, 0.4625000000000000222, 0.4666666666666666741, 0.4708333333333333259, 0.4749999999999999778, 0.4791666666666666852, 0.4833333333333333370, 0.4874999999999999889, 0.4916666666666666408, 0.4958333333333333481, 0.5000000000000000000, 0.5041666666666666519, 0.5083333333333333037, 0.5124999999999999556, 0.5166666666666667185, 0.5208333333333333703, 0.5250000000000000222, 0.5291666666666666741, 0.5333333333333333259, 0.5374999999999999778, 0.5416666666666666297, 0.5458333333333332815, 0.5500000000000000444, 0.5541666666666666963, 0.5583333333333333481, 0.5625000000000000000, 0.5666666666666666519, 0.5708333333333333037, 0.5749999999999999556, 0.5791666666666667185, 0.5833333333333333703, 0.5875000000000000222, 0.5916666666666666741, 0.5958333333333332149, 0.5999999999999999778, 0.6041666666666666297, 0.6083333333333332815, 0.6125000000000000444, 0.6166666666666666963, 0.6208333333333333481, 0.6250000000000000000, 0.6291666666666666519, 0.6333333333333333037, 0.6374999999999999556, 0.6416666666666667185, 0.6458333333333333703, 0.6500000000000000222, 0.6541666666666666741, 0.6583333333333333259, 0.6624999999999999778, 0.6666666666666666297, 0.6708333333333332815, 0.6750000000000000444, 0.6791666666666666963, 0.6833333333333333481, 0.6875000000000000000, 0.6916666666666666519, 0.6958333333333333037, 0.6999999999999999556, 0.7041666666666667185, 0.7083333333333333703, 0.7125000000000000222, 0.7166666666666666741, 0.7208333333333333259, 0.7249999999999999778, 0.7291666666666666297, 0.7333333333333332815, 0.7375000000000000444, 0.7416666666666666963, 0.7458333333333333481, 0.7500000000000000000, 0.7541666666666666519, 0.7583333333333333037, 0.7624999999999999556, 0.7666666666666667185, 0.7708333333333333703, 0.7750000000000000222, 0.7791666666666666741, 0.7833333333333333259, 0.7874999999999999778, 0.7916666666666666297, 0.7958333333333332815, 0.8000000000000000444, 0.8041666666666666963, 0.8083333333333333481, 0.8125000000000000000, 0.8166666666666666519, 0.8208333333333333037, 0.8249999999999999556, 0.8291666666666667185, 0.8333333333333333703, 0.8375000000000000222, 0.8416666666666666741, 0.8458333333333332149, 0.8499999999999999778, 0.8541666666666666297, 0.8583333333333332815, 0.8625000000000000444, 0.8666666666666666963, 0.8708333333333333481, 0.8750000000000000000, 0.8791666666666666519, 0.8833333333333333037, 0.8874999999999999556, 0.8916666666666667185, 0.8958333333333333703, 0.9000000000000000222, 0.9041666666666666741, 0.9083333333333333259, 0.9124999999999999778, 0.9166666666666666297, 0.9208333333333332815, 0.9250000000000000444, 0.9291666666666666963, 0.9333333333333333481, 0.9375000000000000000, 0.9416666666666666519, 0.9458333333333333037, 0.9499999999999999556, 0.9541666666666667185, 0.9583333333333333703, 0.9625000000000000222, 0.9666666666666666741, 0.9708333333333333259, 0.9749999999999999778, 0.9791666666666666297, 0.9833333333333332815, 0.9875000000000000444, 0.9916666666666666963, 0.9958333333333333481, 1.000000000000000000 ),
 .UNSPECIFIED. ) 
 CURVE ( )  GEOMETRIC_REPRESENTATION_ITEM ( )  RATIONAL_B_SPLINE_CURVE ( ( 0.9907048511358500509, 0.9921245532416329560, 1.000000000000000000, 0.9807852804032304306, 1.000000000000000000, 0.9807852804032304306, 1.000000000000000000, 0.9807852804032304306, 1.000000000000000000, 0.9807852804032304306, 1.000000000000000000, 0.9807852804032304306, 1.000000000000000000, 0.9807852804032304306, 1.000000000000000000, 0.9807852804032304306, 1.000000000000000000, 0.9807852804032304306, 1.000000000000000000, 0.9807852804032304306, 1.000000000000000000, 0.9807852804032304306, 1.000000000000000000, 0.9807852804032304306, 1.000000000000000000, 0.9807852804032304306, 1.000000000000000000, 0.9807852804032304306, 1.000000000000000000, 0.9807852804032304306, 1.000000000000000000, 0.9807852804032304306, 1.000000000000000000, 0.9807852804032304306, 1.000000000000000000, 0.9807852804032304306, 1.000000000000000000, 0.9807852804032304306, 1.000000000000000000, 0.9807852804032304306, 1.000000000000000000, 0.9807852804032304306, 1.000000000000000000, 0.9807852804032304306, 1.000000000000000000, 0.9807852804032304306, 1.000000000000000000, 0.9807852804032304306, 1.000000000000000000, 0.9807852804032304306, 1.000000000000000000, 0.9807852804032304306, 1.000000000000000000, 0.9807852804032304306, 1.000000000000000000, 0.9807852804032304306, 1.000000000000000000, 0.9807852804032304306, 1.000000000000000000, 0.9807852804032304306, 1.000000000000000000, 0.9807852804032304306, 1.000000000000000000, 0.9807852804032304306, 1.000000000000000000, 0.9807852804032304306, 1.000000000000000000, 0.9807852804032304306, 1.000000000000000000, 0.9807852804032304306, 1.000000000000000000, 0.9807852804032304306, 1.000000000000000000, 0.9807852804032304306, 1.000000000000000000, 0.9807852804032304306, 1.000000000000000000, 0.9807852804032304306, 1.000000000000000000, 0.9807852804032304306, 1.000000000000000000, 0.9807852804032304306, 1.000000000000000000, 0.9807852804032304306, 1.000000000000000000, 0.9807852804032304306, 1.000000000000000000, 0.9807852804032304306, 1.000000000000000000, 0.9807852804032304306, 1.000000000000000000, 0.9807852804032304306, 1.000000000000000000, 0.9807852804032304306, 1.000000000000000000, 0.9807852804032304306, 1.000000000000000000, 0.9807852804032304306, 1.000000000000000000, 0.9807852804032304306, 1.000000000000000000, 0.9807852804032304306, 1.000000000000000000, 0.9807852804032304306, 1.000000000000000000, 0.9807852804032304306, 1.000000000000000000, 0.9807852804032304306, 1.000000000000000000, 0.9807852804032304306, 1.000000000000000000, 0.9807852804032304306, 1.000000000000000000, 0.9807852804032304306, 1.000000000000000000, 0.9807852804032304306, 1.000000000000000000, 0.9807852804032304306, 1.000000000000000000, 0.9807852804032304306, 1.000000000000000000, 0.9807852804032304306, 1.000000000000000000, 0.9807852804032304306, 1.000000000000000000, 0.9807852804032304306, 1.000000000000000000, 0.9807852804032304306, 1.000000000000000000, 0.9807852804032304306, 1.000000000000000000, 0.9807852804032304306, 1.000000000000000000, 0.9807852804032304306, 1.000000000000000000, 0.9807852804032304306, 1.000000000000000000, 0.9807852804032304306, 1.000000000000000000, 0.9807852804032304306, 1.000000000000000000, 0.9807852804032304306, 1.000000000000000000, 0.9807852804032304306, 1.000000000000000000, 0.9807852804032304306, 1.000000000000000000, 0.9807852804032304306, 1.000000000000000000, 0.9807852804032304306, 1.000000000000000000, 0.9807852804032304306, 1.000000000000000000, 0.9807852804032304306, 1.000000000000000000, 0.9807852804032304306, 1.000000000000000000, 0.9807852804032304306, 1.000000000000000000, 0.9807852804032304306, 1.000000000000000000, 0.9807852804032304306, 1.000000000000000000, 0.9807852804032304306, 1.000000000000000000, 0.9807852804032304306, 1.000000000000000000, 0.9807852804032304306, 1.000000000000000000, 0.9807852804032304306, 1.000000000000000000, 0.9807852804032304306, 1.000000000000000000, 0.9807852804032304306, 1.000000000000000000, 0.9807852804032304306, 1.000000000000000000, 0.9807852804032304306, 1.000000000000000000, 0.9807852804032304306, 1.000000000000000000, 0.9807852804032304306, 1.000000000000000000, 0.9807852804032304306, 1.000000000000000000, 0.9807852804032304306, 1.000000000000000000, 0.9807852804032304306, 1.000000000000000000, 0.9807852804032304306, 1.000000000000000000, 0.9807852804032304306, 1.000000000000000000, 0.9807852804032304306, 1.000000000000000000, 0.9807852804032304306, 1.000000000000000000, 0.9807852804032304306, 1.000000000000000000, 0.9807852804032304306, 1.000000000000000000, 0.9807852804032304306, 1.000000000000000000, 0.9807852804032304306, 1.000000000000000000, 0.9807852804032304306, 1.000000000000000000, 0.9807852804032304306, 1.000000000000000000, 0.9807852804032304306, 1.000000000000000000, 0.9807852804032304306, 1.000000000000000000, 0.9807852804032304306, 1.000000000000000000, 0.9807852804032304306, 1.000000000000000000, 0.9807852804032304306, 1.000000000000000000, 0.9807852804032304306, 1.000000000000000000, 0.9807852804032304306, 1.000000000000000000, 0.9807852804032304306, 1.000000000000000000, 0.9807852804032304306, 1.000000000000000000, 0.9807852804032304306, 1.000000000000000000, 0.9807852804032304306, 1.000000000000000000, 0.9807852804032304306, 1.000000000000000000, 0.9807852804032304306, 1.000000000000000000, 0.9807852804032304306, 1.000000000000000000, 0.9807852804032304306, 1.000000000000000000, 0.9807852804032304306, 1.000000000000000000, 0.9807852804032304306, 1.000000000000000000, 0.9807852804032304306, 1.000000000000000000, 0.9807852804032304306, 1.000000000000000000, 0.9807852804032304306, 1.000000000000000000, 0.9807852804032304306, 1.000000000000000000, 0.9807852804032304306, 1.000000000000000000, 0.9807852804032304306, 1.000000000000000000, 0.9807852804032304306, 1.000000000000000000, 0.9807852804032304306, 1.000000000000000000, 0.9807852804032304306, 1.000000000000000000, 0.9807852804032304306, 1.000000000000000000, 0.9807852804032304306, 1.000000000000000000, 0.9807852804032304306, 1.000000000000000000, 0.9807852804032304306, 1.000000000000000000, 0.9807852804032304306, 1.000000000000000000, 0.9807852804032304306, 1.000000000000000000, 0.9807852804032304306, 1.000000000000000000, 0.9807852804032304306, 1.000000000000000000, 0.9807852804032304306, 1.000000000000000000, 0.9807852804032304306, 1.000000000000000000, 0.9807852804032304306, 1.000000000000000000, 0.9807852804032304306, 1.000000000000000000, 0.9807852804032304306, 1.000000000000000000, 0.9807852804032304306, 1.000000000000000000, 0.9807852804032304306, 1.000000000000000000, 0.9807852804032304306, 1.000000000000000000, 0.9807852804032304306, 1.000000000000000000, 0.9807852804032304306, 1.000000000000000000, 0.9807852804032304306, 1.000000000000000000, 0.9807852804032304306, 1.000000000000000000, 0.9807852804032304306, 1.000000000000000000, 0.9807852804032304306, 1.000000000000000000, 0.9807852804032304306, 1.000000000000000000, 0.9807852804032304306, 1.000000000000000000, 0.9807852804032304306, 1.000000000000000000, 0.9807852804032304306, 1.000000000000000000, 0.9807852804032304306, 1.000000000000000000, 0.9807852804032304306, 1.000000000000000000, 0.9807852804032304306, 1.000000000000000000, 0.9807852804032304306, 1.000000000000000000, 0.9807852804032304306, 1.000000000000000000, 0.9807852804032304306, 1.000000000000000000, 0.9807852804032304306, 1.000000000000000000, 0.9807852804032304306, 1.000000000000000000, 0.9807852804032304306, 1.000000000000000000, 0.9807852804032304306, 1.000000000000000000, 0.9807852804032304306, 1.000000000000000000, 0.9807852804032304306, 1.000000000000000000, 0.9807852804032304306, 1.000000000000000000, 0.9807852804032304306, 1.000000000000000000, 0.9807852804032304306, 1.000000000000000000, 0.9807852804032304306, 1.000000000000000000, 0.9807852804032304306, 1.000000000000000000, 0.9807852804032304306, 1.000000000000000000, 0.9807852804032304306, 1.000000000000000000, 0.9807852804032304306, 1.000000000000000000, 0.9807852804032304306, 1.000000000000000000, 0.9807852804032304306, 1.000000000000000000, 0.9807852804032304306, 1.000000000000000000, 0.9807852804032304306, 1.000000000000000000, 0.9807852804032304306, 1.000000000000000000, 0.9807852804032304306, 1.000000000000000000, 0.9807852804032304306, 1.000000000000000000, 0.9807852804032304306, 1.000000000000000000, 0.9807852804032304306, 1.000000000000000000, 0.9807852804032304306, 1.000000000000000000, 0.9807852804032304306, 1.000000000000000000, 0.9807852804032304306, 1.000000000000000000, 0.9807852804032304306, 1.000000000000000000, 0.9807852804032304306, 1.000000000000000000, 0.9807852804032304306, 1.000000000000000000, 0.9807852804032304306, 1.000000000000000000, 0.9807852804032304306, 1.000000000000000000, 0.9807852804032304306, 1.000000000000000000, 0.9807852804032304306, 1.000000000000000000, 0.9807852804032304306, 1.000000000000000000, 0.9807852804032304306, 1.000000000000000000, 0.9807852804032304306, 1.000000000000000000, 0.9807852804032304306, 1.000000000000000000, 0.9807852804032304306, 1.000000000000000000, 0.9807852804032304306, 1.000000000000000000, 0.9807852804032304306, 1.000000000000000000, 0.9807852804032304306, 1.000000000000000000, 0.9807852804032304306, 1.000000000000000000, 0.9807852804032304306, 1.000000000000000000, 0.9807852804032304306, 1.000000000000000000, 0.9807852804032304306, 1.000000000000000000, 0.9807852804032304306, 1.000000000000000000, 0.9807852804032304306, 1.000000000000000000, 0.9807852804032304306, 1.000000000000000000, 0.9807852804032304306, 1.000000000000000000, 0.9807852804032304306, 1.000000000000000000, 0.9807852804032304306, 1.000000000000000000, 0.9807852804032304306, 1.000000000000000000, 0.9807852804032304306, 1.000000000000000000, 0.9807852804032304306, 1.000000000000000000, 0.9807852804032304306, 1.000000000000000000, 0.9807852804032304306, 1.000000000000000000, 0.9807852804032304306, 1.000000000000000000, 0.9807852804032304306, 1.000000000000000000, 0.9807852804032304306, 1.000000000000000000, 0.9807852804032304306, 1.000000000000000000, 0.9807852804032304306, 1.000000000000000000, 0.9807852804032304306, 1.000000000000000000, 0.9807852804032304306, 1.000000000000000000, 0.9807852804032304306, 1.000000000000000000, 0.9807852804032304306, 1.000000000000000000, 0.9807852804032304306, 1.000000000000000000, 0.9807852804032304306, 1.000000000000000000, 0.9807852804032304306, 1.000000000000000000, 0.9807852804032304306, 1.000000000000000000, 0.9807852804032304306, 1.000000000000000000, 0.9807852804032304306, 1.000000000000000000, 0.9807852804032304306, 1.000000000000000000, 0.9807852804032304306, 1.000000000000000000, 0.9807852804032304306, 1.000000000000000000, 0.9807852804032304306, 1.000000000000000000, 0.9807852804032304306, 1.000000000000000000 ) ) 
 REPRESENTATION_ITEM ( '' )  );
#12162=CARTESIAN_POINT ( 'NONE',  ( 15.50000000000000533, 136.9101862821014777, 0.1745138560725827404 ) ) ;
#12164=CARTESIAN_POINT ( 'NONE',  ( -3.474262827703337830, 134.0351862821014493, -8.843639120294326972 ) ) ;
#12166=CARTESIAN_POINT ( 'NONE',  ( 8.962234695871762469, 34.56018628210144783, -8.715434833791931624 ) ) ;
#12170=CARTESIAN_POINT ( 'NONE',  ( -13.04141134922759804, 123.9726862821014493, -8.927990412390657937 ) ) ;
#12172=CARTESIAN_POINT ( 'NONE',  ( -9.465287035748065847, 3.797686282101448096, -2.064181346179273735 ) ) ;
#12179=CARTESIAN_POINT ( 'NONE',  ( -8.152565276336593669, 80.95231371789854791, -5.233372021372610483 ) ) ;
#12181=AXIS2_PLACEMENT_3D ( 'NONE', #1310, #24445, #26711 ) ;
#12184=CARTESIAN_POINT ( 'NONE',  ( -2.660918448318005058, 91.30231371789855643, -12.46528703574811558 ) ) ;
#12189=CARTESIAN_POINT ( 'NONE',  ( -12.53471296425189152, 71.17731371789855643, -2.311890736173453753 ) ) ;
#12196=CARTESIAN_POINT ( 'NONE',  ( -11.48171059495397373, 40.88518628210144357, -4.944772684328680334 ) ) ;
#12204=CARTESIAN_POINT ( 'NONE',  ( 8.715434833792128799, 92.73981371789855643, -8.962234695871567070 ) ) ;
#12209=CARTESIAN_POINT ( 'NONE',  ( 3.257655550456945548, 59.10231371789854649, 15.46528703574811736 ) ) ;
#12213=CARTESIAN_POINT ( 'NONE',  ( 12.53471296425194836, 81.42268628210145209, -2.311890736173178418 ) ) ;
#12214=CARTESIAN_POINT ( 'NONE',  ( 11.08355503943142750, 43.76018628210144357, -10.83675517735155225 ) ) ;
#12218=CARTESIAN_POINT ( 'NONE',  ( -15.53471296425195369, 49.22268628210144215, 2.908627838312118019 ) ) ;
#12224=CARTESIAN_POINT ( 'NONE',  ( 10.49813415415989581, 27.37268628210144783, 7.228626920339068285 ) ) ;
#12226=CARTESIAN_POINT ( 'NONE',  ( 5.529263428287300108, 141.3273137178985621, 7.954856959092309943 ) ) ;
#12237=CARTESIAN_POINT ( 'NONE',  ( 4.622313124798573369, 46.63518628210145067, 11.61527771782819940 ) ) ;
#12245=CARTESIAN_POINT ( 'NONE',  ( 11.48171059495397728, 91.48518628210145209, 4.944772684328674117 ) ) ;
#12246=CARTESIAN_POINT ( 'NONE',  ( 14.38691631536194393, 11.66481371789854293, 5.770363421894124656 ) ) ;
#12253=CARTESIAN_POINT ( 'NONE',  ( 0.1745138560722779009, 132.9898137178985564, 12.50000000000000355 ) ) ;
#12260=CARTESIAN_POINT ( 'NONE',  ( 13.23911966647199812, 140.7523137178985166, 8.632099005475788900 ) ) ;
#12263=CARTESIAN_POINT ( 'NONE',  ( -11.48171059495397373, 40.88518628210144357, -4.944772684328680334 ) ) ;
#12268=CARTESIAN_POINT ( 'NONE',  ( 8.927990412390657937, 107.8726862821014549, -13.04141134922759804 ) ) ;
#12271=CARTESIAN_POINT ( 'NONE',  ( -6.840914352312096547, 66.76018628210144357, 6.594114490232313663 ) ) ;
#12275=CARTESIAN_POINT ( 'NONE',  ( 7.228626920339068285, 89.47268628210144925, -10.49813415415989581 ) ) ;
#12288=CARTESIAN_POINT ( 'NONE',  ( -8.962234695871565293, 108.8398137178985507, -8.715434833792128799 ) ) ;
#12289=CARTESIAN_POINT ( 'NONE',  ( -6.932735513423968321, 96.94768628210145778, -10.69584247140445221 ) ) ;
#12293=CARTESIAN_POINT ( 'NONE',  ( -14.25334919248795096, 70.31481371789853085, 6.092822981423662299 ) ) ;
#12296=CARTESIAN_POINT ( 'NONE',  ( 8.710071997420127943, 91.48518628210145209, 3.796722387233375073 ) ) ;
#12298=CARTESIAN_POINT ( 'NONE',  ( -8.843639120294245259, 71.46481371789856496, -3.474262827703533230 ) ) ;
#12300=CARTESIAN_POINT ( 'NONE',  ( -6.594114490232462877, 106.5398137178985536, 6.840914352311949109 ) ) ;
#12302=CARTESIAN_POINT ( 'NONE',  ( 2.660918448318002838, 49.90231371789855075, 12.46528703574811558 ) ) ;
#12305=CARTESIAN_POINT ( 'NONE',  ( -8.715434833791929847, 105.8601862821014521, -8.962234695871762469 ) ) ;
#12308=CARTESIAN_POINT ( 'NONE',  ( -2.311890736173176641, 134.3226862821014436, -12.53471296425194836 ) ) ;
#12310=CARTESIAN_POINT ( 'NONE',  ( 14.25334919248782661, 91.48518628210145209, 6.092822981423971385 ) ) ;
#12315=CARTESIAN_POINT ( 'NONE',  ( 8.710071997420127943, 119.0851862821014606, 3.796722387233375073 ) ) ;
#12317=CARTESIAN_POINT ( 'NONE',  ( 8.632099005475504683, 18.74768628210143362, 13.23911966647218996 ) ) ;
#12328=CARTESIAN_POINT ( 'NONE',  ( 7.954856959092311719, 28.62731371789854506, -5.529263428287300108 ) ) ;
#12333=CARTESIAN_POINT ( 'NONE',  ( 2.311890736173452421, 27.47731371789855004, -12.53471296425189152 ) ) ;
#12335=CARTESIAN_POINT ( 'NONE',  ( -2.908627838312453306, 124.0773137178985621, 15.53471296425188797 ) ) ;
#12354=CARTESIAN_POINT ( 'NONE',  ( -8.632099005475501130, 133.7476862821013981, -13.23911966647218996 ) ) ;
#12357=CARTESIAN_POINT ( 'NONE',  ( -9.465287035748065847, 132.5976862821014493, -2.064181346179273735 ) ) ;
#12360=CARTESIAN_POINT ( 'NONE',  ( -2.311890736173176641, 23.92268628210143788, -12.53471296425194836 ) ) ;
#12365=CARTESIAN_POINT ( 'NONE',  ( -6.092822981423970496, 130.5851862821014606, 14.25334919248782661 ) ) ;
#12367=CARTESIAN_POINT ( 'NONE',  ( 5.233372021372610483, 138.4523137178985621, -8.152565276336593669 ) ) ;
#12372=ADVANCED_FACE ( 'NONE', ( #29269 ), #17727, .T. ) ;
#12374=CARTESIAN_POINT ( 'NONE',  ( -3.474262827703527901, 78.36481371789855643, 8.843639120294245259 ) ) ;
#12378=CARTESIAN_POINT ( 'NONE',  ( 10.69584247140429589, 94.75231371789854506, 6.932735513424201024 ) ) ;
#12382=CARTESIAN_POINT ( 'NONE',  ( -0.1745138560722763466, 54.78981371789855359, -12.50000000000000355 ) ) ;
#12390=CARTESIAN_POINT ( 'NONE',  ( -10.49813415415989581, 41.17268628210144499, -7.228626920339068285 ) ) ;
#12394=CARTESIAN_POINT ( 'NONE',  ( 4.944772684328420986, 86.41481371789855359, 11.48171059495408208 ) ) ;
#12399=CARTESIAN_POINT ( 'NONE',  ( 14.38691631536194393, 57.66481371789855359, 5.770363421894124656 ) ) ;
#12403=CARTESIAN_POINT ( 'NONE',  ( -12.46528703574805697, 86.59768628210144925, -2.660918448318280838 ) ) ;
#12404=CARTESIAN_POINT ( 'NONE',  ( 8.927990412390657937, 34.27268628210144641, -13.04141134922759804 ) ) ;
#12407=CARTESIAN_POINT ( 'NONE',  ( -6.092822981423970496, 47.78518628210144215, 14.25334919248782661 ) ) ;
#12415=CARTESIAN_POINT ( 'NONE',  ( -8.715434833791929847, 13.86018628210145032, -8.962234695871762469 ) ) ;
#12418=CARTESIAN_POINT ( 'NONE',  ( -8.710071997420207879, 125.5148137178985763, 3.796722387233182339 ) ) ;
#12429=CARTESIAN_POINT ( 'NONE',  ( 6.932735513423970097, 55.54768628210145209, 10.69584247140445044 ) ) ;
#12437=CARTESIAN_POINT ( 'NONE',  ( 4.944772684328679446, 98.38518628210145778, -11.48171059495397373 ) ) ;
#12438=CARTESIAN_POINT ( 'NONE',  ( -13.04141134922778456, 24.02731371789854364, 8.927990412390377273 ) ) ;
#12446=CARTESIAN_POINT ( 'NONE',  ( 3.474262827703532341, 9.364813717898543999, -8.843639120294245259 ) ) ;
#12451=CARTESIAN_POINT ( 'NONE',  ( -14.25334919248795096, 116.3148137178985735, 6.092822981423662299 ) ) ;
#12455=CARTESIAN_POINT ( 'NONE',  ( -7.228626920339069173, 29.67268628210144499, 10.49813415415989581 ) ) ;
#12459=CARTESIAN_POINT ( 'NONE',  ( 13.04141134922759804, 110.1726862821014663, 8.927990412390657937 ) ) ;
#12462=CARTESIAN_POINT ( 'NONE',  ( -6.594114490232312775, 59.86018628210145209, -6.840914352312096547 ) ) ;
#12465=CARTESIAN_POINT ( 'NONE',  ( -2.660918448318275509, 84.29768628210145209, 12.46528703574805874 ) ) ;
#12478=CARTESIAN_POINT ( 'NONE',  ( -12.46528703574811558, 107.4023137178985650, 2.660918448318003726 ) ) ;
#12479=CARTESIAN_POINT ( 'NONE',  ( 12.46528703574805874, 100.3976862821014464, 2.660918448318279950 ) ) ;
#12484=CARTESIAN_POINT ( 'NONE',  ( -13.04141134922778456, 79.22731371789853938, 8.927990412390377273 ) ) ;
#12488=CARTESIAN_POINT ( 'NONE',  ( 6.594114490232313663, 101.2601862821014436, 6.840914352312096547 ) ) ;
#12491=CARTESIAN_POINT ( 'NONE',  ( 8.843639120294245259, 57.66481371789855359, 3.474262827703527901 ) ) ;
#12494=CARTESIAN_POINT ( 'NONE',  ( -8.152565276336593669, 117.7523137178985735, -5.233372021372610483 ) ) ;
#12496=CARTESIAN_POINT ( 'NONE',  ( 2.311890736173452865, 36.67731371789854933, -12.53471296425189152 ) ) ;
#12498=CARTESIAN_POINT ( 'NONE',  ( 6.932735513423970097, 73.94768628210145778, 10.69584247140445044 ) ) ;
#12505=CARTESIAN_POINT ( 'NONE',  ( 15.46528703574804986, 81.99768628210142651, 3.257655550457285720 ) ) ;
#12510=CARTESIAN_POINT ( 'NONE',  ( -9.465287035748065847, 114.1976862821014578, -2.064181346179273735 ) ) ;
#12512=CARTESIAN_POINT ( 'NONE',  ( -8.715434833791929847, 133.4601862821014606, -8.962234695871762469 ) ) ;
#12524=CARTESIAN_POINT ( 'NONE',  ( -9.534712964251895073, 25.17731371789854933, -1.715153634034446428 ) ) ;
#12529=CARTESIAN_POINT ( 'NONE',  ( -12.53471296425189152, 25.17731371789855288, -2.311890736173453309 ) ) ;
#12531=CARTESIAN_POINT ( 'NONE',  ( 8.632099005475788900, 138.4523137178985621, -13.23911966647199812 ) ) ;
#12539=CARTESIAN_POINT ( 'NONE',  ( 2.311890736173175753, 138.9226862821014663, 12.53471296425194836 ) ) ;
#12550=CARTESIAN_POINT ( 'NONE',  ( -13.23911966647218463, 131.4476862821014436, 8.632099005475506459 ) ) ;
#12552=CARTESIAN_POINT ( 'NONE',  ( -5.529263428287477744, 121.6726862821014521, 7.954856959092191815 ) ) ;
#12554=CARTESIAN_POINT ( 'NONE',  ( 7.228626920339068285, 34.27268628210144641, -10.49813415415989581 ) ) ;
#12558=CARTESIAN_POINT ( 'NONE',  ( 8.927990412390657937, 117.0726862821014294, -13.04141134922759804 ) ) ;
#12560=CARTESIAN_POINT ( 'NONE',  ( -5.233372021372612259, 143.0523137178985280, 8.152565276336593669 ) ) ;
#12567=CARTESIAN_POINT ( 'NONE',  ( -6.840914352311947333, 72.03981371789855359, -6.594114490232462877 ) ) ;
#12571=CARTESIAN_POINT ( 'NONE',  ( 8.715434833792128799, 74.33981371789855075, -8.962234695871567070 ) ) ;
#12573=CARTESIAN_POINT ( 'NONE',  ( -13.99999999999999467, 143.0000000000000000, -1.543483589373963192E-13 ) ) ;
#12575=CARTESIAN_POINT ( 'NONE',  ( 11.48171059495408208, 47.31481371789855928, -4.944772684328420986 ) ) ;
#12579=CARTESIAN_POINT ( 'NONE',  ( -12.46528703574805697, 22.19768628210145067, -2.660918448318280838 ) ) ;
#12584=CARTESIAN_POINT ( 'NONE',  ( 11.61527771782809637, 85.26481371789856212, 4.622313124798827388 ) ) ;
#12589=CARTESIAN_POINT ( 'NONE',  ( 13.04141134922778988, 56.22731371789854649, -8.927990412390371944 ) ) ;
#12593=CARTESIAN_POINT ( 'NONE',  ( -7.228626920339069173, 84.87268628210146915, 10.49813415415989581 ) ) ;
#12594=CARTESIAN_POINT ( 'NONE',  ( 10.83675517735155225, 27.66018628210143859, 11.08355503943142573 ) ) ;
#12599=CARTESIAN_POINT ( 'NONE',  ( -3.257655550457281723, 56.69768628210144357, 15.46528703574804986 ) ) ;
#12605=CARTESIAN_POINT ( 'NONE',  ( 4.944772684328679446, 24.78518628210143859, -11.48171059495397373 ) ) ;
#12606=CARTESIAN_POINT ( 'NONE',  ( -2.064181346179062349, 128.1023137178985678, -9.465287035748106703 ) ) ;
#12611=CARTESIAN_POINT ( 'NONE',  ( 4.944772684328420986, 132.4148137178985678, 11.48171059495408208 ) ) ;
#12617=CARTESIAN_POINT ( 'NONE',  ( 8.715434833791931624, 46.06018628210144072, 8.962234695871760692 ) ) ;
#12626=CARTESIAN_POINT ( 'NONE',  ( -0.1745138560725500443, 84.01018628210145778, 12.50000000000000355 ) ) ;
#12627=CARTESIAN_POINT ( 'NONE',  ( -6.092822981423666739, 17.41481371789854649, -14.25334919248795096 ) ) ;
#12633=CARTESIAN_POINT ( 'NONE',  ( 8.962234695871567070, 141.0398137178985678, 8.715434833792127023 ) ) ;
#12639=CARTESIAN_POINT ( 'NONE',  ( -5.770363421894122880, 105.9648137178985650, 14.38691631536194393 ) ) ;
#12643=CARTESIAN_POINT ( 'NONE',  ( -8.962234695871760692, 29.96018628210143930, 8.715434833791933400 ) ) ;
#12647=CARTESIAN_POINT ( 'NONE',  ( 14.25334919248782661, 109.8851862821014720, 6.092822981423971385 ) ) ;
#12650=CARTESIAN_POINT ( 'NONE',  ( 9.465287035748067623, 35.99768628210143362, 2.064181346179272847 ) ) ;
#12654=CARTESIAN_POINT ( 'NONE',  ( 11.61527771782819940, 81.13518628210145778, -4.622313124798573369 ) ) ;
#12657=CARTESIAN_POINT ( 'NONE',  ( 5.233372021372432847, 46.34768628210144925, 8.152565276336710909 ) ) ;
#12665=CARTESIAN_POINT ( 'NONE',  ( -2.311890736173448424, 96.47731371789855359, 12.53471296425189330 ) ) ;
#12666=CARTESIAN_POINT ( 'NONE',  ( -2.311890736173176641, 106.7226862821014635, -12.53471296425194659 ) ) ;
#12667=EDGE_LOOP ( 'NONE', ( #7039, #30243, #19756, #29848, #16169 ) ) ;
#12672=CARTESIAN_POINT ( 'NONE',  ( -8.927990412390371944, 72.32731371789854791, -13.04141134922778988 ) ) ;
#12675=CARTESIAN_POINT ( 'NONE',  ( -5.233372021372430183, 96.94768628210147199, -8.152565276336710909 ) ) ;
#12677=CARTESIAN_POINT ( 'NONE',  ( -3.796722387233185003, 63.41481371789855359, -8.710071997420207879 ) ) ;
#12679=CARTESIAN_POINT ( 'NONE',  ( 2.064181346179061460, 114.3023137178985422, 9.465287035748106703 ) ) ;
#12681=CARTESIAN_POINT ( 'NONE',  ( -8.962234695871565293, 35.23981371789855643, -8.715434833792128799 ) ) ;
#12683=CARTESIAN_POINT ( 'NONE',  ( 8.962234695871762469, 89.76018628210144357, -8.715434833791931624 ) ) ;
#12690=CARTESIAN_POINT ( 'NONE',  ( -9.465287035748065847, 104.9976862821014549, -2.064181346179273735 ) ) ;
#12692=CARTESIAN_POINT ( 'NONE',  ( 10.49813415415989581, 128.5726862821014720, 7.228626920339068285 ) ) ;
#12694=CARTESIAN_POINT ( 'NONE',  ( -7.751135216212685641, 143.0000000000000568, 8.679851443715339343 ) ) ;
#12705=CARTESIAN_POINT ( 'NONE',  ( -9.500000000000005329, 15.68981371789854329, 0.1745138560723101806 ) ) ;
#12711=CARTESIAN_POINT ( 'NONE',  ( 12.46528703574811558, 29.20231371789855501, -2.660918448318005947 ) ) ;
#12714=CARTESIAN_POINT ( 'NONE',  ( 15.46528703574811736, 139.6023137178985394, -3.257655550456947768 ) ) ;
#12723=CARTESIAN_POINT ( 'NONE',  ( 8.962234695871762469, 135.7601862821014720, -8.715434833791931624 ) ) ;
#12732=CARTESIAN_POINT ( 'NONE',  ( -10.69584247140444866, 140.6476862821014890, 6.932735513423972762 ) ) ;
#12736=CARTESIAN_POINT ( 'NONE',  ( -15.53471296425195369, 132.0226862821014322, 2.908627838312118019 ) ) ;
#12738=CARTESIAN_POINT ( 'NONE',  ( 7.954856959092191815, 119.3726862821014265, 5.529263428287477744 ) ) ;
#12740=CARTESIAN_POINT ( 'NONE',  ( 11.48171059495397728, 27.08518628210144996, 4.944772684328674117 ) ) ;
#12744=CARTESIAN_POINT ( 'NONE',  ( 11.08355503943142750, 117.3601862821014663, -10.83675517735155225 ) ) ;
#12746=CARTESIAN_POINT ( 'NONE',  ( -8.710071997420207879, 143.9148137178985678, 3.796722387233182339 ) ) ;
#12754=CARTESIAN_POINT ( 'NONE',  ( 3.474262827703532341, 82.96481371789856496, -8.843639120294245259 ) ) ;
#12757=CARTESIAN_POINT ( 'NONE',  ( -4.944772684328424539, 72.61481371789855643, -11.48171059495408031 ) ) ;
#12761=CARTESIAN_POINT ( 'NONE',  ( -4.622313124798826500, 41.56481371789855217, 11.61527771782809637 ) ) ;
#12766=CARTESIAN_POINT ( 'NONE',  ( -6.932735513423968321, 14.14768628210144463, -10.69584247140445221 ) ) ;
#12770=CARTESIAN_POINT ( 'NONE',  ( 4.622313124798831829, 82.96481371789856496, -11.61527771782809282 ) ) ;
#12775=CARTESIAN_POINT ( 'NONE',  ( -2.908627838312453306, 50.47731371789854649, 15.53471296425188797 ) ) ;
#12778=CARTESIAN_POINT ( 'NONE',  ( 12.50000000000000355, 81.71018628210144641, 0.1745138560725507937 ) ) ;
#12779=CARTESIAN_POINT ( 'NONE',  ( -6.092822981423970496, 20.18518628210144783, 14.25334919248782661 ) ) ;
#12784=CARTESIAN_POINT ( 'NONE',  ( -8.632099005475501130, 41.74768628210143362, -13.23911966647218996 ) ) ;
#12790=CARTESIAN_POINT ( 'NONE',  ( 8.715434833791931624, 27.66018628210144215, 8.962234695871760692 ) ) ;
#12792=CARTESIAN_POINT ( 'NONE',  ( -9.534712964251895073, 135.5773137178985905, -1.715153634034446428 ) ) ;
#12796=CARTESIAN_POINT ( 'NONE',  ( -0.1745138560722763466, 137.5898137178985792, -12.50000000000000355 ) ) ;
#12801=CARTESIAN_POINT ( 'NONE',  ( -7.228626920339070061, 57.27268628210143930, 10.49813415415989404 ) ) ;
#12810=CARTESIAN_POINT ( 'NONE',  ( 11.48171059495397728, 82.28518628210146346, 4.944772684328674117 ) ) ;
#12811=CARTESIAN_POINT ( 'NONE',  ( 3.257655550456945548, 13.10231371789855181, 15.46528703574811736 ) ) ;
#12817=CARTESIAN_POINT ( 'NONE',  ( -8.152565276336593669, 7.352313717898546486, -5.233372021372610483 ) ) ;
#12823=CARTESIAN_POINT ( 'NONE',  ( -10.83675517735179028, 106.5398137178985536, 11.08355503943118947 ) ) ;
#12826=CARTESIAN_POINT ( 'NONE',  ( -10.49813415415989581, 22.77268628210143575, -7.228626920339068285 ) ) ;
#12831=CARTESIAN_POINT ( 'NONE',  ( 11.08355503943142750, 108.1601862821014635, -10.83675517735155225 ) ) ;
#12835=CARTESIAN_POINT ( 'NONE',  ( 9.500000000000005329, 35.71018628210144641, 0.1745138560725188748 ) ) ;
#12840=CARTESIAN_POINT ( 'NONE',  ( 0.1745138560725515708, 79.41018628210144925, -12.50000000000000355 ) ) ;
#12842=CARTESIAN_POINT ( 'NONE',  ( 8.843639120294328748, 53.53518628210145636, -3.474262827703334722 ) ) ;
#12853=CARTESIAN_POINT ( 'NONE',  ( -10.49813415416004858, 79.22731371789855359, 7.228626920338839135 ) ) ;
#12854=CARTESIAN_POINT ( 'NONE',  ( 7.228626920339069173, 98.67268628210146630, -10.49813415415989404 ) ) ;
#12860=CARTESIAN_POINT ( 'NONE',  ( 14.38691631536194393, 66.86481371789854222, 5.770363421894124656 ) ) ;
#12864=CARTESIAN_POINT ( 'NONE',  ( 1.715153634034233487, 92.92268628210145209, 9.534712964251941258 ) ) ;
#12866=CARTESIAN_POINT ( 'NONE',  ( -3.474262827703527901, 50.76481371789856212, 8.843639120294245259 ) ) ;
#12868=CARTESIAN_POINT ( 'NONE',  ( -8.710071997420207879, 116.3148137178985735, 3.796722387233182339 ) ) ;
#12870=CARTESIAN_POINT ( 'NONE',  ( 12.50000000000000355, 38.68981371789855217, -0.1745138560722771515 ) ) ;
#12871=CARTESIAN_POINT ( 'NONE',  ( -0.1745138560725500443, 84.01018628210145778, 12.50000000000000355 ) ) ;
#12880=CARTESIAN_POINT ( 'NONE',  ( -2.064181346179269738, 93.49768628210142651, 9.465287035748067623 ) ) ;
#12883=CARTESIAN_POINT ( 'NONE',  ( 12.53471296425194836, 127.4226862821014663, -2.311890736173178418 ) ) ;
#12897=CARTESIAN_POINT ( 'NONE',  ( 0.1745138560723095977, 13.38981371789854613, 9.500000000000005329 ) ) ;
#12904=CARTESIAN_POINT ( 'NONE',  ( -10.69584247140429412, 25.75231371789854506, -6.932735513424201024 ) ) ;
#12906=CARTESIAN_POINT ( 'NONE',  ( -15.46528703574811736, 125.8023137178985706, 3.257655550456946436 ) ) ;
#12913=CARTESIAN_POINT ( 'NONE',  ( -4.944772684328673229, 130.5851862821014606, 11.48171059495397728 ) ) ;
#12921=CARTESIAN_POINT ( 'NONE',  ( 7.228626920339068285, 135.4726862821014493, -10.49813415415989581 ) ) ;
#12925=CARTESIAN_POINT ( 'NONE',  ( 8.632099005475504683, 138.3476862821014208, 13.23911966647218996 ) ) ;
#12927=CARTESIAN_POINT ( 'NONE',  ( -3.474262827703337830, 115.6351862821014436, -8.843639120294326972 ) ) ;
#12931=CARTESIAN_POINT ( 'NONE',  ( -0.1745138560725500443, 10.41018628210144215, 12.50000000000000355 ) ) ;
#12935=CARTESIAN_POINT ( 'NONE',  ( -14.38691631536207183, 113.3351862821014606, 5.770363421893814682 ) ) ;
#12937=CARTESIAN_POINT ( 'NONE',  ( -9.465287035748106703, 144.2023137178985905, 2.064181346179061460 ) ) ;
#12942=CIRCLE ( 'NONE', #37138, 1.499999999999990452 ) ;
#12944=CARTESIAN_POINT ( 'NONE',  ( 3.474262827703532341, 73.76481371789856212, -8.843639120294245259 ) ) ;
#12947=CARTESIAN_POINT ( 'NONE',  ( -12.53471296425189152, 89.57731371789856212, -2.311890736173453309 ) ) ;
#12949=CARTESIAN_POINT ( 'NONE',  ( -6.769757451167472517, 143.0000000000000568, 10.84521838874742627 ) ) ;
#12951=CARTESIAN_POINT ( 'NONE',  ( 0.1745138560722779009, 50.18981371789854506, 12.50000000000000355 ) ) ;
#12956=CARTESIAN_POINT ( 'NONE',  ( -0.1745138560725500443, 19.61018628210144144, 12.50000000000000355 ) ) ;
#12962=CARTESIAN_POINT ( 'NONE',  ( 2.660918448318002838, 77.50231371789855928, 12.46528703574811558 ) ) ;
#12968=CARTESIAN_POINT ( 'NONE',  ( -13.23911966647199812, 62.55231371789854222, -8.632099005475788900 ) ) ;
#12972=CARTESIAN_POINT ( 'NONE',  ( -12.53471296425194836, 76.82268628210145778, 2.311890736173176641 ) ) ;
#12974=CARTESIAN_POINT ( 'NONE',  ( 15.46528703574804986, 26.79768628210144144, 3.257655550457285720 ) ) ;
#12978=CARTESIAN_POINT ( 'NONE',  ( 2.908627838312118019, 46.92268628210143788, 15.53471296425195369 ) ) ;
#12984=CARTESIAN_POINT ( 'NONE',  ( -6.932735513423968321, 23.34768628210144570, -10.69584247140445221 ) ) ;
#12986=CARTESIAN_POINT ( 'NONE',  ( -8.843639120294245259, 135.8648137178985849, -3.474262827703533230 ) ) ;
#12992=CARTESIAN_POINT ( 'NONE',  ( -8.962234695871565293, 136.4398137178985735, -8.715434833792128799 ) ) ;
#12998=CARTESIAN_POINT ( 'NONE',  ( -8.962234695871760692, 39.16018628210144215, 8.715434833791933400 ) ) ;
#13006=CARTESIAN_POINT ( 'NONE',  ( -10.69584247140444866, 76.24768628210144072, 6.932735513423972762 ) ) ;
#13007=CARTESIAN_POINT ( 'NONE',  ( -14.25334919248782306, 132.8851862821014436, -6.092822981423979378 ) ) ;
#13013=CARTESIAN_POINT ( 'NONE',  ( 9.500000000000005329, 11.08981371789854897, -0.1745138560723090149 ) ) ;
#13019=CARTESIAN_POINT ( 'NONE',  ( 8.927990412390371944, 104.5273137178985650, 13.04141134922778811 ) ) ;
#13023=CARTESIAN_POINT ( 'NONE',  ( 6.932735513423970097, 138.3476862821014493, 10.69584247140445044 ) ) ;
#13026=CARTESIAN_POINT ( 'NONE',  ( -5.770363421893818234, 106.4351862821014691, -14.38691631536207005 ) ) ;
#13029=CARTESIAN_POINT ( 'NONE',  ( 8.710071997420127943, 45.48518628210144499, 3.796722387233375073 ) ) ;
#13034=CARTESIAN_POINT ( 'NONE',  ( 0.1745138560725515708, 70.21018628210144641, -12.50000000000000355 ) ) ;
#13037=CARTESIAN_POINT ( 'NONE',  ( -3.474262827703337830, 42.03518628210144925, -8.843639120294326972 ) ) ;
#13047=CARTESIAN_POINT ( 'NONE',  ( 4.622313124798831829, 92.16481371789855359, -11.61527771782809282 ) ) ;
#13048=CARTESIAN_POINT ( 'NONE',  ( 4.622313124798573369, 111.0351862821014635, 11.61527771782819940 ) ) ;
#13053=CARTESIAN_POINT ( 'NONE',  ( 14.25334919248795451, 65.71481371789855075, -6.092822981423661410 ) ) ;
#13059=CARTESIAN_POINT ( 'NONE',  ( 5.233372021372610483, 64.85231371789855359, -8.152565276336593669 ) ) ;
#13061=CARTESIAN_POINT ( 'NONE',  ( -5.233372021372612259, 106.2523137178985451, 8.152565276336593669 ) ) ;
#13063=CARTESIAN_POINT ( 'NONE',  ( 11.48171059495408208, 28.91481371789854293, -4.944772684328420986 ) ) ;
#13064=CARTESIAN_POINT ( 'NONE',  ( -8.962234695871760692, 85.16018628210144925, 8.715434833791933400 ) ) ;
#13073=CARTESIAN_POINT ( 'NONE',  ( 1.715153634034233487, 92.92268628210145209, 9.534712964251941258 ) ) ;
#13076=CARTESIAN_POINT ( 'NONE',  ( 7.228626920339068285, 135.4726862821014493, -10.49813415415989581 ) ) ;
#13086=CARTESIAN_POINT ( 'NONE',  ( -12.46528703574811558, 144.2023137178985621, 2.660918448318003726 ) ) ;
#13091=CARTESIAN_POINT ( 'NONE',  ( -12.53471296425189152, 34.37731371789855217, -2.311890736173453309 ) ) ;
#13093=CARTESIAN_POINT ( 'NONE',  ( 13.23911966647199812, 122.3523137178985394, 8.632099005475788900 ) ) ;
#13099=CARTESIAN_POINT ( 'NONE',  ( 6.932735513423970097, 138.3476862821014493, 10.69584247140445044 ) ) ;
#13111=CARTESIAN_POINT ( 'NONE',  ( -13.23911966647218463, 113.0476862821014663, 8.632099005475506459 ) ) ;
#13115=CARTESIAN_POINT ( 'NONE',  ( 9.500000000000005329, 118.5101862821014720, 0.1745138560725188748 ) ) ;
#13117=CARTESIAN_POINT ( 'NONE',  ( 8.715434833791931624, 9.260186282101429356, 8.962234695871760692 ) ) ;
#13121=CARTESIAN_POINT ( 'NONE',  ( 8.152565276336714462, 90.04768628210145209, -5.233372021372432847 ) ) ;
#13123=CARTESIAN_POINT ( 'NONE',  ( -1.715153634034442431, 133.2773137178985507, 9.534712964251900402 ) ) ;
#13129=CARTESIAN_POINT ( 'NONE',  ( 3.474262827703532341, 64.56481371789854506, -8.843639120294245259 ) ) ;
#13132=CARTESIAN_POINT ( 'NONE',  ( 4.944772684328420986, 86.41481371789855359, 11.48171059495408208 ) ) ;
#13136=CARTESIAN_POINT ( 'NONE',  ( -12.53471296425189152, 43.57731371789855501, -2.311890736173453753 ) ) ;
#13140=CARTESIAN_POINT ( 'NONE',  ( 11.48171059495397728, 27.08518628210144996, 4.944772684328674117 ) ) ;
#13147=CARTESIAN_POINT ( 'NONE',  ( -4.944772684328424539, 72.61481371789855643, -11.48171059495408031 ) ) ;
#13152=CARTESIAN_POINT ( 'NONE',  ( 14.25334919248795451, 47.31481371789856638, -6.092822981423661410 ) ) ;
#13155=CARTESIAN_POINT ( 'NONE',  ( -10.69584247140444866, 76.24768628210144072, 6.932735513423972762 ) ) ;
#13156=CARTESIAN_POINT ( 'NONE',  ( 6.092822981423978490, 24.78518628210144215, -14.25334919248782306 ) ) ;
#13160=CARTESIAN_POINT ( 'NONE',  ( 8.927990412390657937, 25.07268628210145067, -13.04141134922759804 ) ) ;
#13168=CARTESIAN_POINT ( 'NONE',  ( -6.840914352311947333, 127.2398137178985422, -6.594114490232462877 ) ) ;
#13173=CARTESIAN_POINT ( 'NONE',  ( -12.53471296425189152, 135.5773137178985905, -2.311890736173453309 ) ) ;
#13181=CARTESIAN_POINT ( 'NONE',  ( -10.69584247140444866, 30.24768628210144783, 6.932735513423972762 ) ) ;
#13189=CARTESIAN_POINT ( 'NONE',  ( -0.1745138560725500443, 74.81018628210145494, 12.50000000000000355 ) ) ;
#13191=CARTESIAN_POINT ( 'NONE',  ( -15.53471296425188442, 6.777313717898553413, -2.908627838312459080 ) ) ;
#13199=CARTESIAN_POINT ( 'NONE',  ( 4.622313124798831829, 119.7648137178985763, -11.61527771782809282 ) ) ;
#13206=CARTESIAN_POINT ( 'NONE',  ( 11.08355503943118769, 104.2398137178985706, 10.83675517735179028 ) ) ;
#13210=CARTESIAN_POINT ( 'NONE',  ( -0.1745138560725500443, 130.0101862821014436, 12.50000000000000355 ) ) ;
#13211=CARTESIAN_POINT ( 'NONE',  ( 11.08355503943142750, 89.76018628210145778, -10.83675517735155225 ) ) ;
#13214=CARTESIAN_POINT ( 'NONE',  ( 14.38691631536207538, 90.33518628210144641, -5.770363421893813793 ) ) ;
#13218=CARTESIAN_POINT ( 'NONE',  ( 9.534712964251941258, 44.62268628210144783, -1.715153634034235708 ) ) ;
#13222=CARTESIAN_POINT ( 'NONE',  ( -11.61527771782819940, 67.33518628210144641, 4.622313124798574258 ) ) ;
#13227=CARTESIAN_POINT ( 'NONE',  ( -3.796722387233375073, 47.78518628210144215, 8.710071997420127943 ) ) ;
#13236=CARTESIAN_POINT ( 'NONE',  ( 10.69584247140429589, 85.55231371789857064, 6.932735513424201024 ) ) ;
#13237=CARTESIAN_POINT ( 'NONE',  ( 8.962234695871762469, 89.76018628210144357, -8.715434833791931624 ) ) ;
#13243=CARTESIAN_POINT ( 'NONE',  ( -5.770363421894122880, 50.76481371789856212, 14.38691631536194393 ) ) ;
#13248=CARTESIAN_POINT ( 'NONE',  ( 0.1745138560723095977, 59.38981371789856212, 9.500000000000005329 ) ) ;
#13251=CARTESIAN_POINT ( 'NONE',  ( -8.152565276336593669, 99.35231371789856780, -5.233372021372610483 ) ) ;
#13253=CARTESIAN_POINT ( 'NONE',  ( -8.962234695871565293, 26.03981371789855359, -8.715434833792128799 ) ) ;
#13254=CARTESIAN_POINT ( 'NONE',  ( -11.48171059495397373, 77.68518628210145494, -4.944772684328680334 ) ) ;
#13260=CARTESIAN_POINT ( 'NONE',  ( -5.233372021372430183, 87.74768628210144072, -8.152565276336710909 ) ) ;
#13262=CARTESIAN_POINT ( 'NONE',  ( 2.660918448318279950, 125.6976862821014578, -12.46528703574805697 ) ) ;
#13272=CARTESIAN_POINT ( 'NONE',  ( -8.715434833792127023, 143.3398137178985507, 8.962234695871568846 ) ) ;
#13277=CARTESIAN_POINT ( 'NONE',  ( 11.48171059495408208, 10.51481371789855856, -4.944772684328420986 ) ) ;
#13279=CARTESIAN_POINT ( 'NONE',  ( -11.08355503943118592, 108.8398137178985507, -10.83675517735179383 ) ) ;
#13285=CARTESIAN_POINT ( 'NONE',  ( -4.944772684328673229, 139.7851862821014493, 11.48171059495397728 ) ) ;
#13293=CARTESIAN_POINT ( 'NONE',  ( -10.69584247140444866, 131.4476862821014436, 6.932735513423972762 ) ) ;
#13298=CARTESIAN_POINT ( 'NONE',  ( 2.908627838312118019, 120.5226862821014322, 15.53471296425195369 ) ) ;
#13300=CARTESIAN_POINT ( 'NONE',  ( 4.944772684328679446, 15.58518628210145351, -11.48171059495397373 ) ) ;
#13305=CARTESIAN_POINT ( 'NONE',  ( 9.500000000000005329, 81.71018628210144641, 0.1745138560725188748 ) ) ;
#13306=CARTESIAN_POINT ( 'NONE',  ( 8.152565276336593669, 122.3523137178985394, 5.233372021372610483 ) ) ;
#13313=CARTESIAN_POINT ( 'NONE',  ( -0.1745138560723084320, 63.98981371789855643, -9.500000000000005329 ) ) ;
#13317=CARTESIAN_POINT ( 'NONE',  ( -8.962234695871565293, 53.63981371789855501, -8.715434833792128799 ) ) ;
#13321=CARTESIAN_POINT ( 'NONE',  ( 12.53471296425189330, 29.77731371789854720, 2.311890736173451977 ) ) ;
#13325=CARTESIAN_POINT ( 'NONE',  ( -2.311890736173176641, 23.92268628210143788, -12.53471296425194836 ) ) ;
#13331=CARTESIAN_POINT ( 'NONE',  ( 7.228626920338837358, 67.72731371789856780, 10.49813415416005036 ) ) ;
#13336=CARTESIAN_POINT ( 'NONE',  ( 15.53471296425188797, 48.17731371789854222, 2.908627838312457747 ) ) ;
#13340=CARTESIAN_POINT ( 'NONE',  ( 8.962234695871762469, 62.16018628210144215, -8.715434833791931624 ) ) ;
#13341=CARTESIAN_POINT ( 'NONE',  ( 14.38691631536207538, 7.535186282101451916, -5.770363421893813793 ) ) ;
#13345=CARTESIAN_POINT ( 'NONE',  ( -15.50000000000000533, 31.11018628210143433, -0.1745138560725808530 ) ) ;
#13352=CARTESIAN_POINT ( 'NONE',  ( -0.1745138560725500443, 10.41018628210144215, 12.50000000000000355 ) ) ;
#13354=CARTESIAN_POINT ( 'NONE',  ( -7.954856959092309943, 116.0273137178985792, 5.529263428287300108 ) ) ;
#13359=CARTESIAN_POINT ( 'NONE',  ( 7.228626920338837358, 141.3273137178985621, 10.49813415416005036 ) ) ;
#13365=CARTESIAN_POINT ( 'NONE',  ( 2.311890736173175753, 28.52268628210144641, 12.53471296425194659 ) ) ;
#13373=CARTESIAN_POINT ( 'NONE',  ( -11.48171059495397373, 77.68518628210145494, -4.944772684328680334 ) ) ;
#13374=CARTESIAN_POINT ( 'NONE',  ( 10.83675517735179206, 9.939813717898537959, -11.08355503943118769 ) ) ;
#13381=CARTESIAN_POINT ( 'NONE',  ( 11.48171059495408208, 120.9148137178985536, -4.944772684328420986 ) ) ;
#13387=CARTESIAN_POINT ( 'NONE',  ( -5.770363421894122880, 96.76481371789854791, 14.38691631536194393 ) ) ;
#13391=CARTESIAN_POINT ( 'NONE',  ( -7.228626920339069173, 121.6726862821014521, 10.49813415415989581 ) ) ;
#13392=CARTESIAN_POINT ( 'NONE',  ( 11.08355503943142750, 62.16018628210144925, -10.83675517735155225 ) ) ;
#13396=CARTESIAN_POINT ( 'NONE',  ( 14.38691631536207538, 81.13518628210145778, -5.770363421893813793 ) ) ;
#13400=CARTESIAN_POINT ( 'NONE',  ( -0.1745138560725182642, 38.01018628210144357, 9.500000000000005329 ) ) ;
#13404=CARTESIAN_POINT ( 'NONE',  ( -2.311890736173176641, 60.72268628210144925, -12.53471296425194836 ) ) ;
#13407=CARTESIAN_POINT ( 'NONE',  ( -5.529263428287477744, 20.47268628210143859, 7.954856959092191815 ) ) ;
#13417=CARTESIAN_POINT ( 'NONE',  ( -2.311890736173448424, 87.27731371789856496, 12.53471296425189330 ) ) ;
#13418=CARTESIAN_POINT ( 'NONE',  ( -4.944772684328673229, 84.58518628210146062, 11.48171059495397728 ) ) ;
#13423=CARTESIAN_POINT ( 'NONE',  ( -8.927990412390371944, 53.92731371789854222, -13.04141134922778988 ) ) ;
#13428=CARTESIAN_POINT ( 'NONE',  ( -3.796722387233185003, 35.81481371789853796, -8.710071997420207879 ) ) ;
#13430=CARTESIAN_POINT ( 'NONE',  ( 0.1745138560723095977, 96.18981371789855928, 9.500000000000005329 ) ) ;
#13432=CARTESIAN_POINT ( 'NONE',  ( 4.622313124798831829, 9.364813717898545775, -11.61527771782809282 ) ) ;
#13435=CARTESIAN_POINT ( 'NONE',  ( -6.932735513423968321, 69.34768628210143504, -10.69584247140445221 ) ) ;
#13444=CARTESIAN_POINT ( 'NONE',  ( -9.500000000000005329, 95.51018628210147199, -0.1745138560725176813 ) ) ;
#13447=CARTESIAN_POINT ( 'NONE',  ( 10.49813415415989581, 119.3726862821014549, 7.228626920339068285 ) ) ;
#13459=CARTESIAN_POINT ( 'NONE',  ( 2.660918448318002838, 141.9023137178985792, 12.46528703574811558 ) ) ;
#13464=CARTESIAN_POINT ( 'NONE',  ( 6.932735513424201024, 9.652313717898541867, -10.69584247140429412 ) ) ;
#13466=CARTESIAN_POINT ( 'NONE',  ( 5.770363421894130873, 119.7648137178985905, -14.38691631536193860 ) ) ;
#13472=CARTESIAN_POINT ( 'NONE',  ( 0.1745138560725515708, 116.2101862821014606, -12.50000000000000355 ) ) ;
#13478=CARTESIAN_POINT ( 'NONE',  ( 0.1745138560725515708, 134.6101862821014663, -12.50000000000000355 ) ) ;
#13482=CARTESIAN_POINT ( 'NONE',  ( -15.50000000000000533, 123.1101862821014663, -0.1745138560725808530 ) ) ;
#13484=CARTESIAN_POINT ( 'NONE',  ( -10.49813415415989581, 4.372686282101440725, -7.228626920339068285 ) ) ;
#13488=CARTESIAN_POINT ( 'NONE',  ( -9.500000000000005329, 77.11018628210145209, -0.1745138560725176813 ) ) ;
#13490=CARTESIAN_POINT ( 'NONE',  ( 8.710071997420211432, 130.1148137178985564, -3.796722387233181895 ) ) ;
#13497=CARTESIAN_POINT ( 'NONE',  ( -9.534712964251895073, 61.97731371789853938, -1.715153634034446428 ) ) ;
#13501=CARTESIAN_POINT ( 'NONE',  ( 12.53471296425189330, 66.57731371789856212, 2.311890736173451533 ) ) ;
#13505=CARTESIAN_POINT ( 'NONE',  ( -11.61527771782809282, 34.66481371789854649, -4.622313124798832717 ) ) ;
#13516=CARTESIAN_POINT ( 'NONE',  ( -10.49813415416004858, 60.82731371789855501, 7.228626920338839135 ) ) ;
#13521=CARTESIAN_POINT ( 'NONE',  ( 5.770363421894130873, 46.16481371789854649, -14.38691631536193860 ) ) ;
#13524=CARTESIAN_POINT ( 'NONE',  ( 0.1745138560725515708, 33.41018628210144925, -12.50000000000000355 ) ) ;
#13526=CARTESIAN_POINT ( 'NONE',  ( -11.48171059495397373, 59.28518628210144215, -4.944772684328680334 ) ) ;
#13527=CARTESIAN_POINT ( 'NONE',  ( -14.25334919248782306, 13.28518628210143149, -6.092822981423979378 ) ) ;
#13532=CARTESIAN_POINT ( 'NONE',  ( -0.1745138560725817967, 28.81018628210143717, 15.50000000000000533 ) ) ;
#13539=CARTESIAN_POINT ( 'NONE',  ( 12.50000000000000355, 8.110186282101444988, 0.1745138560725507937 ) ) ;
#13542=CARTESIAN_POINT ( 'NONE',  ( -2.064181346179062349, 109.7023137178985479, -9.465287035748106703 ) ) ;
#13547=CARTESIAN_POINT ( 'NONE',  ( 10.69584247140429589, 113.1523137178985650, 6.932735513424201024 ) ) ;
#13553=CARTESIAN_POINT ( 'NONE',  ( 12.50000000000000355, 26.51018628210144357, 0.1745138560725507937 ) ) ;
#13562=CARTESIAN_POINT ( 'NONE',  ( 6.932735513423970097, 64.74768628210145494, 10.69584247140445044 ) ) ;
#13563=CARTESIAN_POINT ( 'NONE',  ( -2.908627838312119351, 134.3226862821014436, -15.53471296425195369 ) ) ;
#13570=CARTESIAN_POINT ( 'NONE',  ( -12.50000000000000355, 126.0898137178985650, 0.1745138560722786503 ) ) ;
#13576=CARTESIAN_POINT ( 'NONE',  ( 15.53471296425188797, 94.17731371789857064, 2.908627838312457747 ) ) ;
#13581=CARTESIAN_POINT ( 'NONE',  ( 0.1745138560725515708, 116.2101862821014606, -12.50000000000000355 ) ) ;
#13582=CARTESIAN_POINT ( 'NONE',  ( 15.50000000000000533, 72.51018628210145778, 0.1745138560725827404 ) ) ;
#13586=CARTESIAN_POINT ( 'NONE',  ( 0.1745138560725837118, 79.41018628210144925, -15.50000000000000533 ) ) ;
#13592=CARTESIAN_POINT ( 'NONE',  ( -9.534712964251941258, 21.62268628210143717, 1.715153634034234154 ) ) ;
#13596=CARTESIAN_POINT ( 'NONE',  ( -4.622313124798576922, 51.23518628210143788, -11.61527771782819762 ) ) ;
#13599=CARTESIAN_POINT ( 'NONE',  ( -6.594114490232312775, 23.06018628210144783, -6.840914352312096547 ) ) ;
#13612=CARTESIAN_POINT ( 'NONE',  ( -6.932735513424201912, 87.85231371789855359, 10.69584247140429412 ) ) ;
#13613=CARTESIAN_POINT ( 'NONE',  ( -8.962234695871760692, 94.36018628210145209, 8.715434833791933400 ) ) ;
#13618=CARTESIAN_POINT ( 'NONE',  ( -6.092822981423666739, 54.21481371789855785, -14.25334919248795096 ) ) ;
#13624=CARTESIAN_POINT ( 'NONE',  ( 9.534712964251900402, 38.97731371789853938, 1.715153634034445540 ) ) ;
#13626=CARTESIAN_POINT ( 'NONE',  ( 9.534712964251900402, 94.17731371789857064, 1.715153634034445540 ) ) ;
#13628=CARTESIAN_POINT ( 'NONE',  ( 8.715434833792128799, 9.939813717898537959, -8.962234695871567070 ) ) ;
#13630=CARTESIAN_POINT ( 'NONE',  ( 4.622313124798573369, 55.83518628210144641, 11.61527771782819940 ) ) ;
#13638=CARTESIAN_POINT ( 'NONE',  ( -0.1745138560725182642, 102.4101862821014493, 9.500000000000005329 ) ) ;
#13639=CARTESIAN_POINT ( 'NONE',  ( -6.932735513423968321, 115.3476862821014635, -10.69584247140445221 ) ) ;
#13651=CARTESIAN_POINT ( 'NONE',  ( 10.69584247140429589, 140.7523137178985735, 6.932735513424201024 ) ) ;
#13652=CARTESIAN_POINT ( 'NONE',  ( 11.48171059495397728, 137.4851862821014663, 4.944772684328674117 ) ) ;
#13659=CARTESIAN_POINT ( 'NONE',  ( -10.83675517735179028, 115.7398137178985564, 11.08355503943118947 ) ) ;
#13667=CARTESIAN_POINT ( 'NONE',  ( -12.53471296425194836, 122.8226862821014720, 2.311890736173176641 ) ) ;
#13676=CARTESIAN_POINT ( 'NONE',  ( -2.311890736173176641, 115.9226862821014521, -12.53471296425194836 ) ) ;
#13682=CARTESIAN_POINT ( 'NONE',  ( -10.83675517735155047, 115.0601862821014691, -11.08355503943142750 ) ) ;
#13684=CARTESIAN_POINT ( 'NONE',  ( -11.61527771782819940, 12.13518628210144534, 4.622313124798574258 ) ) ;
#13688=CARTESIAN_POINT ( 'NONE',  ( -1.715153634034234598, 79.12268628210145494, -9.534712964251941258 ) ) ;
#13693=CARTESIAN_POINT ( 'NONE',  ( -7.954856959092309943, 51.62731371789855928, 5.529263428287300108 ) ) ;
#13697=CARTESIAN_POINT ( 'NONE',  ( 2.311890736173452421, 55.07731371789854791, -12.53471296425189152 ) ) ;
#13701=CARTESIAN_POINT ( 'NONE',  ( -2.660918448318004614, 26.90231371789854364, -12.46528703574811558 ) ) ;
#13713=CARTESIAN_POINT ( 'NONE',  ( 10.49813415416005213, 74.62731371789855928, -7.228626920338837358 ) ) ;
#13719=CARTESIAN_POINT ( 'NONE',  ( -11.08355503943118592, 35.23981371789855643, -10.83675517735179383 ) ) ;
#13721=CARTESIAN_POINT ( 'NONE',  ( -4.944772684328673229, 20.18518628210144783, 11.48171059495397728 ) ) ;
#13722=CARTESIAN_POINT ( 'NONE',  ( 4.944772684328679446, 61.58518628210145351, -11.48171059495397373 ) ) ;
#13723=CARTESIAN_POINT ( 'NONE',  ( -13.04141134922759804, 4.372686282101438948, -8.927990412390657937 ) ) ;
#13728=CARTESIAN_POINT ( 'NONE',  ( 11.08355503943142750, 25.36018628210144854, -10.83675517735155225 ) ) ;
#13736=CARTESIAN_POINT ( 'NONE',  ( -8.710071997420207879, 116.3148137178985735, 3.796722387233182339 ) ) ;
#13743=CARTESIAN_POINT ( 'NONE',  ( 2.660918448318003282, 114.3023137178985564, 12.46528703574811558 ) ) ;
#13756=CARTESIAN_POINT ( 'NONE',  ( -0.1745138560725500443, 65.61018628210145209, 12.50000000000000355 ) ) ;
#13762=CARTESIAN_POINT ( 'NONE',  ( -0.1745138560722763466, 119.1898137178985593, -12.50000000000000355 ) ) ;
#13767=CARTESIAN_POINT ( 'NONE',  ( -15.50000000000000533, 98.48981371789855643, 0.1745138560722471477 ) ) ;
#13772=CARTESIAN_POINT ( 'NONE',  ( 12.50000000000000355, 127.7101862821014606, 0.1745138560725507937 ) ) ;
#13773=CARTESIAN_POINT ( 'NONE',  ( -15.53471296425195369, 58.42268628210145209, 2.908627838312118019 ) ) ;
#13776=CARTESIAN_POINT ( 'NONE',  ( 5.770363421893814682, 83.43518628210145494, 14.38691631536207183 ) ) ;
#13779=CARTESIAN_POINT ( 'NONE',  ( -9.534712964251941258, 12.42268628210144144, 1.715153634034234154 ) ) ;
#13784=CARTESIAN_POINT ( 'NONE',  ( -10.69584247140444866, 67.04768628210145209, 6.932735513423972762 ) ) ;
#13787=CARTESIAN_POINT ( 'NONE',  ( 9.465287035748067623, 26.79768628210144144, 2.064181346179272847 ) ) ;
#13799=CARTESIAN_POINT ( 'NONE',  ( 7.228626920339069173, 80.27268628210146062, -10.49813415415989404 ) ) ;
#13804=CARTESIAN_POINT ( 'NONE',  ( -14.25334919248795096, 51.91481371789856070, 6.092822981423662299 ) ) ;
#13811=CARTESIAN_POINT ( 'NONE',  ( -8.843639120294245259, 34.66481371789854649, -3.474262827703533230 ) ) ;
#13813=CARTESIAN_POINT ( 'NONE',  ( -9.534712964251895073, 98.77731371789855075, -1.715153634034446428 ) ) ;
#13815=CARTESIAN_POINT ( 'NONE',  ( 12.53471296425189330, 11.37731371789854506, 2.311890736173451977 ) ) ;
#13816=CARTESIAN_POINT ( 'NONE',  ( -10.69584247140444866, 67.04768628210145209, 6.932735513423972762 ) ) ;
#13824=CARTESIAN_POINT ( 'NONE',  ( -6.594114490232312775, 69.06018628210144072, -6.840914352312096547 ) ) ;
#13826=CARTESIAN_POINT ( 'NONE',  ( 2.660918448318279950, 107.2976862821014521, -12.46528703574805697 ) ) ;
#13839=CARTESIAN_POINT ( 'NONE',  ( 10.69584247140429589, 131.5523137178985564, 6.932735513424201024 ) ) ;
#13840=CARTESIAN_POINT ( 'NONE',  ( 0.1745138560725515708, 134.6101862821014663, -12.50000000000000355 ) ) ;
#13846=CARTESIAN_POINT ( 'NONE',  ( -0.1745138560722442889, 109.9898137178985706, -15.50000000000000533 ) ) ;
#13852=CARTESIAN_POINT ( 'NONE',  ( -2.311890736173176641, 115.9226862821014521, -12.53471296425194836 ) ) ;
#13858=CARTESIAN_POINT ( 'NONE',  ( 12.50000000000000355, 118.5101862821014578, 0.1745138560725507937 ) ) ;
#13863=CARTESIAN_POINT ( 'NONE',  ( 5.770363421893814682, 111.0351862821014635, 14.38691631536207183 ) ) ;
#13864=CARTESIAN_POINT ( 'NONE',  ( -0.1745138560725500443, 10.41018628210144215, 12.50000000000000355 ) ) ;
#13866=CARTESIAN_POINT ( 'NONE',  ( -0.1745138560725182642, 139.2101862821014890, 9.500000000000005329 ) ) ;
#13871=CARTESIAN_POINT ( 'NONE',  ( 9.465287035748067623, 72.79768628210145209, 2.064181346179272847 ) ) ;
#13880=CARTESIAN_POINT ( 'NONE',  ( 3.796722387233182339, 49.61481371789856354, 8.710071997420207879 ) ) ;
#13884=CARTESIAN_POINT ( 'NONE',  ( 4.944772684328420986, 68.01481371789854791, 11.48171059495408208 ) ) ;
#13887=CARTESIAN_POINT ( 'NONE',  ( -12.50000000000000355, 24.88981371789854435, 0.1745138560722786503 ) ) ;
#13902=CARTESIAN_POINT ( 'NONE',  ( 5.770363421894130873, 36.96481371789853654, -14.38691631536193860 ) ) ;
#13904=CARTESIAN_POINT ( 'NONE',  ( -4.944772684328673229, 10.98518628210143433, 11.48171059495397728 ) ) ;
#13905=CARTESIAN_POINT ( 'NONE',  ( -11.61527771782819940, 58.13518628210144357, 4.622313124798574258 ) ) ;
#13906=CARTESIAN_POINT ( 'NONE',  ( -0.1745138560725817967, 10.41018628210144037, 15.50000000000000533 ) ) ;
#13910=CARTESIAN_POINT ( 'NONE',  ( 14.38691631536207538, 35.13518628210143646, -5.770363421893813793 ) ) ;
#13919=CARTESIAN_POINT ( 'NONE',  ( 5.529263428287300108, 113.7273137178985678, 7.954856959092309943 ) ) ;
#13924=CARTESIAN_POINT ( 'NONE',  ( -12.46528703574811558, 116.6023137178985536, 2.660918448318004170 ) ) ;
#13938=CARTESIAN_POINT ( 'NONE',  ( 11.61527771782819940, 53.53518628210144925, -4.622313124798573369 ) ) ;
#13945=CARTESIAN_POINT ( 'NONE',  ( 10.49813415416005213, 120.6273137178985735, -7.228626920338837358 ) ) ;
#13951=CARTESIAN_POINT ( 'NONE',  ( 8.927990412390371944, 86.12731371789853085, 13.04141134922778811 ) ) ;
#13955=CARTESIAN_POINT ( 'NONE',  ( 2.311890736173175753, 129.7226862821014777, 12.53471296425194836 ) ) ;
#13956=CARTESIAN_POINT ( 'NONE',  ( -3.257655550457281723, 56.69768628210144357, 15.46528703574804986 ) ) ;
#13959=CARTESIAN_POINT ( 'NONE',  ( 8.927990412390657937, 80.27268628210143220, -13.04141134922759804 ) ) ;
#13961=CARTESIAN_POINT ( 'NONE',  ( -6.840914352312096547, 29.96018628210143575, 6.594114490232313663 ) ) ;
#13965=CARTESIAN_POINT ( 'NONE',  ( 2.311890736173175753, 56.12268628210144072, 12.53471296425194836 ) ) ;
#13968=CARTESIAN_POINT ( 'NONE',  ( 9.534712964251941258, 26.22268628210144925, -1.715153634034235708 ) ) ;
#13978=CARTESIAN_POINT ( 'NONE',  ( 10.49813415415989581, 73.37268628210144072, 7.228626920339069173 ) ) ;
#13983=CARTESIAN_POINT ( 'NONE',  ( -15.46528703574811736, 43.00231371789853796, 3.257655550456946436 ) ) ;
#13990=CARTESIAN_POINT ( 'NONE',  ( -8.152565276336593669, 44.15231371789854364, -5.233372021372610483 ) ) ;
#13993=CARTESIAN_POINT ( 'NONE',  ( -3.796722387233185003, 100.2148137178985650, -8.710071997420207879 ) ) ;
#13995=CARTESIAN_POINT ( 'NONE',  ( 3.257655550456945548, 141.9023137178985507, 15.46528703574811736 ) ) ;
#13996=CARTESIAN_POINT ( 'NONE',  ( -4.622313124798576922, 69.63518628210145778, -11.61527771782819762 ) ) ;
#14003=CARTESIAN_POINT ( 'NONE',  ( -3.474262827703337830, 78.83518628210146062, -8.843639120294326972 ) ) ;
#14006=CARTESIAN_POINT ( 'NONE',  ( -8.715434833791929847, 115.0601862821014549, -8.962234695871762469 ) ) ;
#14013=ADVANCED_FACE ( 'NONE', ( #36030 ), #294, .T. ) ;
#14021=CARTESIAN_POINT ( 'NONE',  ( -12.46528703574811558, 116.6023137178985678, 2.660918448318003726 ) ) ;
#14022=CARTESIAN_POINT ( 'NONE',  ( -10.49813415415989404, 133.1726862821014663, -7.228626920339069173 ) ) ;
#14027=CARTESIAN_POINT ( 'NONE',  ( 10.83675517735179206, 101.9398137178985735, -11.08355503943118769 ) ) ;
#14033=CARTESIAN_POINT ( 'NONE',  ( 7.228626920339068285, 117.0726862821014720, -10.49813415415989581 ) ) ;
#14040=CARTESIAN_POINT ( 'NONE',  ( -6.932735513423968321, 124.5476862821014663, -10.69584247140445221 ) ) ;
#14045=CARTESIAN_POINT ( 'NONE',  ( -0.1745138560725817967, 102.4101862821014493, 15.50000000000000533 ) ) ;
#14046=CARTESIAN_POINT ( 'NONE',  ( 8.715434833791931624, 18.46018628210144286, 8.962234695871760692 ) ) ;
#14049=CARTESIAN_POINT ( 'NONE',  ( -5.529263428287477744, 140.0726862821014151, 7.954856959092191815 ) ) ;
#14054=CARTESIAN_POINT ( 'NONE',  ( 0.1745138560725194299, 61.01018628210145067, -9.500000000000005329 ) ) ;
#14062=CARTESIAN_POINT ( 'NONE',  ( 9.465287035748106703, 38.40231371789853654, -2.064181346179063237 ) ) ;
#14066=CARTESIAN_POINT ( 'NONE',  ( 2.311890736173452421, 64.27731371789855075, -12.53471296425189152 ) ) ;
#14069=CARTESIAN_POINT ( 'NONE',  ( 4.944772684328420986, 22.01481371789855501, 11.48171059495408208 ) ) ;
#14072=CARTESIAN_POINT ( 'NONE',  ( 10.69584247140445221, 7.247686282101428290, -6.932735513423970097 ) ) ;
#14084=CARTESIAN_POINT ( 'NONE',  ( 10.83675517735179206, 19.13981371789855146, -11.08355503943118769 ) ) ;
#14086=CARTESIAN_POINT ( 'NONE',  ( 3.474262827703335166, 138.6351862821014720, 8.843639120294326972 ) ) ;
#14087=CARTESIAN_POINT ( 'NONE',  ( 7.228626920339068285, 43.47268628210144925, -10.49813415415989581 ) ) ;
#14091=CARTESIAN_POINT ( 'NONE',  ( 11.08355503943142750, 16.16018628210144570, -10.83675517735155225 ) ) ;
#14099=CARTESIAN_POINT ( 'NONE',  ( 2.064181346179061460, 114.3023137178985422, 9.465287035748106703 ) ) ;
#14106=CARTESIAN_POINT ( 'NONE',  ( -10.69584247140429412, 117.7523137178986019, -6.932735513424201024 ) ) ;
#14119=CARTESIAN_POINT ( 'NONE',  ( -12.50000000000000355, 49.51018628210145067, -0.1745138560725492671 ) ) ;
#14126=CARTESIAN_POINT ( 'NONE',  ( 12.53471296425189330, 103.3773137178985735, 2.311890736173451977 ) ) ;
#14132=CARTESIAN_POINT ( 'NONE',  ( 13.04141134922778988, 102.2273137178985678, -8.927990412390371944 ) ) ;
#14136=CARTESIAN_POINT ( 'NONE',  ( 12.53471296425194836, 99.82268628210144357, -2.311890736173178418 ) ) ;
#14137=CARTESIAN_POINT ( 'NONE',  ( 15.53471296425195369, 72.22268628210143504, -2.908627838312120684 ) ) ;
#14141=CARTESIAN_POINT ( 'NONE',  ( 15.50000000000000533, 63.31018628210144783, 0.1745138560725827404 ) ) ;
#14144=CARTESIAN_POINT ( 'NONE',  ( 7.954856959092191815, 27.37268628210144428, 5.529263428287477744 ) ) ;
#14147=CARTESIAN_POINT ( 'NONE',  ( -8.715434833791929847, 50.66018628210144925, -8.962234695871762469 ) ) ;
#14150=CARTESIAN_POINT ( 'NONE',  ( 9.465287035748067623, 17.59768628210143504, 2.064181346179272847 ) ) ;
#14161=CARTESIAN_POINT ( 'NONE',  ( 12.46528703574805874, 72.79768628210145209, 2.660918448318279950 ) ) ;
#14166=CARTESIAN_POINT ( 'NONE',  ( 2.908627838312458636, 36.67731371789854933, -15.53471296425188442 ) ) ;
#14173=CARTESIAN_POINT ( 'NONE',  ( 1.715153634034445762, 27.47731371789854649, -9.534712964251895073 ) ) ;
#14177=CARTESIAN_POINT ( 'NONE',  ( -4.622313124798826500, 13.96481371789853831, 11.61527771782809637 ) ) ;
#14181=CARTESIAN_POINT ( 'NONE',  ( 8.962234695871762469, 62.16018628210144215, -8.715434833791931624 ) ) ;
#14190=CARTESIAN_POINT ( 'NONE',  ( 9.534712964251941258, 81.42268628210145209, -1.715153634034235708 ) ) ;
#14192=CARTESIAN_POINT ( 'NONE',  ( -11.48171059495397373, 105.2851862821014493, -4.944772684328680334 ) ) ;
#14205=CARTESIAN_POINT ( 'NONE',  ( -11.48171059495408208, 125.5148137178985763, 4.944772684328421875 ) ) ;
#14206=CARTESIAN_POINT ( 'NONE',  ( -2.311890736173176641, 125.1226862821014691, -12.53471296425194659 ) ) ;
#14213=CARTESIAN_POINT ( 'NONE',  ( 0.1745138560722461762, 96.18981371789855928, 15.50000000000000533 ) ) ;
#14214=CARTESIAN_POINT ( 'NONE',  ( -11.48171059495397373, 96.08518628210146062, -4.944772684328680334 ) ) ;
#14217=CARTESIAN_POINT ( 'NONE',  ( 11.48171059495397728, 119.0851862821014606, 4.944772684328674117 ) ) ;
#14222=CARTESIAN_POINT ( 'NONE',  ( 4.944772684328679446, 125.9851862821014521, -11.48171059495397373 ) ) ;
#14228=CARTESIAN_POINT ( 'NONE',  ( -15.53471296425195369, 95.22268628210143504, 2.908627838312118019 ) ) ;
#14229=CARTESIAN_POINT ( 'NONE',  ( -8.715434833791929847, 23.06018628210145138, -8.962234695871762469 ) ) ;
#14233=CARTESIAN_POINT ( 'NONE',  ( 6.594114490232313663, 138.0601862821014549, 6.840914352312096547 ) ) ;
#14239=CARTESIAN_POINT ( 'NONE',  ( 5.529263428287477744, 71.07268628210144357, -7.954856959092191815 ) ) ;
#14246=CARTESIAN_POINT ( 'NONE',  ( 3.796722387233182339, 31.21481371789855430, 8.710071997420207879 ) ) ;
#14251=CARTESIAN_POINT ( 'NONE',  ( 4.944772684328420986, 40.41481371789855359, 11.48171059495408208 ) ) ;
#14254=CARTESIAN_POINT ( 'NONE',  ( -8.632099005475794229, 143.0523137178985280, 13.23911966647199812 ) ) ;
#14258=CARTESIAN_POINT ( 'NONE',  ( -11.61527771782819940, 12.13518628210144534, 4.622313124798574258 ) ) ;
#14271=CARTESIAN_POINT ( 'NONE',  ( 13.23911966647199812, 30.35231371789855359, 8.632099005475788900 ) ) ;
#14273=CARTESIAN_POINT ( 'NONE',  ( 12.46528703574805874, 17.59768628210143859, 2.660918448318279950 ) ) ;
#14274=CARTESIAN_POINT ( 'NONE',  ( -8.962234695871760692, 48.36018628210145209, 8.715434833791933400 ) ) ;
#14285=CARTESIAN_POINT ( 'NONE',  ( 2.064181346179061460, 95.90231371789855075, 9.465287035748106703 ) ) ;
#14292=CARTESIAN_POINT ( 'NONE',  ( -2.660918448318005058, 109.7023137178985763, -12.46528703574811558 ) ) ;
#14296=CARTESIAN_POINT ( 'NONE',  ( -12.50000000000000355, 70.88981371789856212, 0.1745138560722786503 ) ) ;
#14306=CARTESIAN_POINT ( 'NONE',  ( -2.660918448318275509, 56.69768628210145067, 12.46528703574805874 ) ) ;
#14311=CARTESIAN_POINT ( 'NONE',  ( -8.715434833792127023, 97.33981371789855075, 8.962234695871568846 ) ) ;
#14317=CARTESIAN_POINT ( 'NONE',  ( -5.770363421894122880, 69.16481371789853938, 14.38691631536194393 ) ) ;
#14321=CARTESIAN_POINT ( 'NONE',  ( 8.715434833791931624, 110.4601862821014606, 8.962234695871760692 ) ) ;
#14322=CARTESIAN_POINT ( 'NONE',  ( 13.23911966647218996, 53.24768628210144783, -8.632099005475504683 ) ) ;
#14325=CARTESIAN_POINT ( 'NONE',  ( -14.38691631536207183, 58.13518628210145067, 5.770363421893814682 ) ) ;
#14331=CARTESIAN_POINT ( 'NONE',  ( 2.660918448318279950, 33.69768628210145067, -12.46528703574805697 ) ) ;
#14334=CARTESIAN_POINT ( 'NONE',  ( -0.1745138560725182642, 10.41018628210144037, 9.500000000000005329 ) ) ;
#14346=CARTESIAN_POINT ( 'NONE',  ( -8.715434833791929847, 59.86018628210145209, -8.962234695871762469 ) ) ;
#14353=CARTESIAN_POINT ( 'NONE',  ( -14.38691631536193860, 43.86481371789854933, -5.770363421894132649 ) ) ;
#14360=CARTESIAN_POINT ( 'NONE',  ( 8.843639120294245259, 11.66481371789854293, 3.474262827703527901 ) ) ;
#14364=CARTESIAN_POINT ( 'NONE',  ( -14.25334919248795096, 134.7148137178985507, 6.092822981423662299 ) ) ;
#14367=CARTESIAN_POINT ( 'NONE',  ( 2.311890736173175753, 37.72268628210144215, 12.53471296425194836 ) ) ;
#14374=CARTESIAN_POINT ( 'NONE',  ( 8.710071997420127943, 73.08518628210143220, 3.796722387233375073 ) ) ;
#14375=CARTESIAN_POINT ( 'NONE',  ( -4.622313124798576922, 97.23518628210145209, -11.61527771782819762 ) ) ;
#14388=CARTESIAN_POINT ( 'NONE',  ( 7.228626920338837358, 113.7273137178985820, 10.49813415416005036 ) ) ;
#14389=CARTESIAN_POINT ( 'NONE',  ( 10.69584247140445221, 126.8476862821014635, -6.932735513423970097 ) ) ;
#14395=CARTESIAN_POINT ( 'NONE',  ( -11.08355503943118592, 99.63981371789857633, -10.83675517735179383 ) ) ;
#14399=CARTESIAN_POINT ( 'NONE',  ( -2.064181346179062349, 82.10231371789853938, -9.465287035748106703 ) ) ;
#14402=CARTESIAN_POINT ( 'NONE',  ( 8.715434833792128799, 74.33981371789855075, -8.962234695871567070 ) ) ;
#14405=CARTESIAN_POINT ( 'NONE',  ( 2.311890736173175753, 111.3226862821014720, 12.53471296425194836 ) ) ;
#14411=CARTESIAN_POINT ( 'NONE',  ( -14.38691631536207183, 104.1351862821014720, 5.770363421893814682 ) ) ;
#14412=CARTESIAN_POINT ( 'NONE',  ( -12.50000000000000355, 21.91018628210143859, -0.1745138560725492671 ) ) ;
#14415=CARTESIAN_POINT ( 'NONE',  ( 8.843639120294328748, 127.1351862821014720, -3.474262827703334722 ) ) ;
#14419=CARTESIAN_POINT ( 'NONE',  ( -3.474262827703337830, 69.63518628210144357, -8.843639120294326972 ) ) ;
#14426=CARTESIAN_POINT ( 'NONE',  ( -3.796722387233185003, 35.81481371789853796, -8.710071997420207879 ) ) ;
#14433=CARTESIAN_POINT ( 'NONE',  ( 12.50000000000000355, 38.68981371789855217, -0.1745138560722771515 ) ) ;
#14436=CARTESIAN_POINT ( 'NONE',  ( -5.770363421894122880, 142.7648137178985621, 14.38691631536194393 ) ) ;
#14451=CARTESIAN_POINT ( 'NONE',  ( 14.38691631536194393, 20.86481371789854578, 5.770363421894124656 ) ) ;
#14453=CARTESIAN_POINT ( 'NONE',  ( 11.48171059495397728, 8.685186282101437172, 4.944772684328674117 ) ) ;
#14454=CARTESIAN_POINT ( 'NONE',  ( 6.932735513423970097, 55.54768628210144499, 10.69584247140445044 ) ) ;
#14467=CARTESIAN_POINT ( 'NONE',  ( -1.715153634034442431, 96.47731371789852517, 9.534712964251900402 ) ) ;
#14475=CARTESIAN_POINT ( 'NONE',  ( 8.962234695871567070, 104.2398137178985564, 8.715434833792127023 ) ) ;
#14479=CARTESIAN_POINT ( 'NONE',  ( 4.622313124798831829, 64.56481371789855928, -11.61527771782809282 ) ) ;
#14487=CARTESIAN_POINT ( 'NONE',  ( -2.311890736173176641, 42.32268628210145067, -12.53471296425194836 ) ) ;
#14492=CARTESIAN_POINT ( 'NONE',  ( -0.1745138560722763466, 109.9898137178985706, -12.50000000000000355 ) ) ;
#14497=CARTESIAN_POINT ( 'NONE',  ( 8.927990412390371944, 76.92731371789854222, 13.04141134922778811 ) ) ;
#14502=CARTESIAN_POINT ( 'NONE',  ( 4.622313124798573369, 111.0351862821014635, 11.61527771782819940 ) ) ;
#14503=CARTESIAN_POINT ( 'NONE',  ( 15.50000000000000533, 54.11018628210144499, 0.1745138560725827404 ) ) ;
#14507=CARTESIAN_POINT ( 'NONE',  ( 15.50000000000000533, 72.51018628210145778, 0.1745138560725827404 ) ) ;
#14514=CARTESIAN_POINT ( 'NONE',  ( 12.46528703574805874, 45.19768628210143646, 2.660918448318279950 ) ) ;
#14517=CARTESIAN_POINT ( 'NONE',  ( -8.710071997420207879, 143.9148137178985678, 3.796722387233182339 ) ) ;
#14527=CARTESIAN_POINT ( 'NONE',  ( 11.48171059495397728, 73.08518628210144641, 4.944772684328674117 ) ) ;
#14536=CARTESIAN_POINT ( 'NONE',  ( 8.927990412390371944, 40.12731371789853796, 13.04141134922778811 ) ) ;
#14542=CARTESIAN_POINT ( 'NONE',  ( -2.064181346179062349, 26.90231371789854364, -9.465287035748106703 ) ) ;
#14548=CARTESIAN_POINT ( 'NONE',  ( -6.092822981423666739, 127.8148137178985735, -14.25334919248795096 ) ) ;
#14551=CARTESIAN_POINT ( 'NONE',  ( 7.228626920339068285, 43.47268628210144925, -10.49813415415989581 ) ) ;
#14559=CARTESIAN_POINT ( 'NONE',  ( -7.954856959092191815, 68.77268628210143220, -5.529263428287477744 ) ) ;
#14562=CARTESIAN_POINT ( 'NONE',  ( 10.49813415415989581, 91.77268628210144641, 7.228626920339068285 ) ) ;
#14574=CARTESIAN_POINT ( 'NONE',  ( 8.715434833792128799, 129.5398137178985678, -8.962234695871567070 ) ) ;
#14575=CARTESIAN_POINT ( 'NONE',  ( -6.932735513423968321, 124.5476862821014521, -10.69584247140445221 ) ) ;
#14581=CARTESIAN_POINT ( 'NONE',  ( -15.50000000000000533, 89.28981371789856780, 0.1745138560722471477 ) ) ;
#14585=CARTESIAN_POINT ( 'NONE',  ( 5.529263428287300108, 67.72731371789853938, 7.954856959092309943 ) ) ;
#14590=CARTESIAN_POINT ( 'NONE',  ( -4.944772684328424539, 45.01481371789854791, -11.48171059495408031 ) ) ;
#14592=CARTESIAN_POINT ( 'NONE',  ( 7.228626920339068285, 107.8726862821014549, -10.49813415415989581 ) ) ;
#14599=CARTESIAN_POINT ( 'NONE',  ( 11.08355503943142750, 98.96018628210144641, -10.83675517735155225 ) ) ;
#14600=CARTESIAN_POINT ( 'NONE',  ( -7.228626920339070061, 20.47268628210143859, 10.49813415415989404 ) ) ;
#14603=CARTESIAN_POINT ( 'NONE',  ( 6.594114490232313663, 128.8601862821014663, 6.840914352312096547 ) ) ;
#14608=CARTESIAN_POINT ( 'NONE',  ( 7.954856959092191815, 64.17268628210143788, 5.529263428287477744 ) ) ;
#14614=CARTESIAN_POINT ( 'NONE',  ( -9.534712964251895073, 43.57731371789854080, -1.715153634034446428 ) ) ;
#14619=CARTESIAN_POINT ( 'NONE',  ( -11.61527771782809282, 53.06481371789854506, -4.622313124798832717 ) ) ;
#14623=CARTESIAN_POINT ( 'NONE',  ( -7.228626920338836470, 17.12731371789854862, -10.49813415416005213 ) ) ;
#14637=CARTESIAN_POINT ( 'NONE',  ( 14.25334919248795451, 28.91481371789854649, -6.092822981423661410 ) ) ;
#14641=CARTESIAN_POINT ( 'NONE',  ( 8.715434833791931624, 9.260186282101429356, 8.962234695871760692 ) ) ;
#14642=CARTESIAN_POINT ( 'NONE',  ( 12.50000000000000355, 44.91018628210144215, 0.1745138560725507937 ) ) ;
#14653=CARTESIAN_POINT ( 'NONE',  ( -9.500000000000005329, 89.28981371789856780, 0.1745138560723101806 ) ) ;
#14659=CARTESIAN_POINT ( 'NONE',  ( 12.50000000000000355, 103.0898137178985650, -0.1745138560722771515 ) ) ;
#14663=CARTESIAN_POINT ( 'NONE',  ( -0.1745138560722763466, 73.18981371789855928, -12.50000000000000355 ) ) ;
#14672=CARTESIAN_POINT ( 'NONE',  ( 12.46528703574805874, 35.99768628210144072, 2.660918448318279950 ) ) ;
#14677=CARTESIAN_POINT ( 'NONE',  ( 8.715434833792128799, 111.1398137178985621, -8.962234695871567070 ) ) ;
#14683=CARTESIAN_POINT ( 'NONE',  ( 10.83675517735179206, 83.53981371789856780, -11.08355503943118769 ) ) ;
#14687=CARTESIAN_POINT ( 'NONE',  ( 12.53471296425194836, 109.0226862821014606, -2.311890736173178418 ) ) ;
#14688=CARTESIAN_POINT ( 'NONE',  ( 14.38691631536207538, 53.53518628210145636, -5.770363421893813793 ) ) ;
#14692=CARTESIAN_POINT ( 'NONE',  ( -14.38691631536207183, 67.33518628210143220, 5.770363421893814682 ) ) ;
#14699=CARTESIAN_POINT ( 'NONE',  ( 6.932735513423970097, 46.34768628210145636, 10.69584247140445044 ) ) ;
#14702=CARTESIAN_POINT ( 'NONE',  ( -1.715153634034234598, 14.72268628210143859, -9.534712964251941258 ) ) ;
#14714=CARTESIAN_POINT ( 'NONE',  ( -4.944772684328673229, 75.38518628210144357, 11.48171059495397728 ) ) ;
#14722=CARTESIAN_POINT ( 'NONE',  ( -15.53471296425188442, 43.57731371789854080, -2.908627838312459080 ) ) ;
#14729=CARTESIAN_POINT ( 'NONE',  ( 8.152565276336593669, 21.15231371789855430, 5.233372021372610483 ) ) ;
#14736=CARTESIAN_POINT ( 'NONE',  ( 15.46528703574811736, 130.4023137178985792, -3.257655550456947768 ) ) ;
#14739=CARTESIAN_POINT ( 'NONE',  ( -7.228626920339069173, 48.07268628210143646, 10.49813415415989581 ) ) ;
#14747=CARTESIAN_POINT ( 'NONE',  ( -1.715153634034234598, 60.72268628210144925, -9.534712964251941258 ) ) ;
#14752=CARTESIAN_POINT ( 'NONE',  ( 6.932735513423970097, 101.5476862821014379, 10.69584247140445044 ) ) ;
#14763=CARTESIAN_POINT ( 'NONE',  ( 11.48171059495408208, 130.1148137178985564, -4.944772684328420986 ) ) ;
#14765=CARTESIAN_POINT ( 'NONE',  ( -8.962234695871760692, 131.1601862821014777, 8.715434833791933400 ) ) ;
#14771=CARTESIAN_POINT ( 'NONE',  ( 15.53471296425188797, 94.17731371789857064, 2.908627838312457747 ) ) ;
#14777=CARTESIAN_POINT ( 'NONE',  ( 3.796722387233182339, 77.21481371789855075, 8.710071997420207879 ) ) ;
#14781=CARTESIAN_POINT ( 'NONE',  ( -4.622313124798826500, 41.56481371789855217, 11.61527771782809637 ) ) ;
#14783=CARTESIAN_POINT ( 'NONE',  ( 8.715434833791931624, 92.06018628210145494, 8.962234695871760692 ) ) ;
#14787=CARTESIAN_POINT ( 'NONE',  ( 8.927990412390657937, 107.8726862821014549, -13.04141134922759804 ) ) ;
#14790=CARTESIAN_POINT ( 'NONE',  ( -2.064181346179269738, 111.8976862821014606, 9.465287035748067623 ) ) ;
#14792=CARTESIAN_POINT ( 'NONE',  ( -2.908627838312119351, 14.72268628210143859, -15.53471296425195369 ) ) ;
#14798=CARTESIAN_POINT ( 'NONE',  ( -9.500000000000005329, 67.91018628210144925, -0.1745138560725176813 ) ) ;
#14806=CARTESIAN_POINT ( 'NONE',  ( -8.710071997420207879, 42.71481371789855075, 3.796722387233182339 ) ) ;
#14810=CARTESIAN_POINT ( 'NONE',  ( -8.715434833792127023, 51.33981371789855785, 8.962234695871568846 ) ) ;
#14812=CARTESIAN_POINT ( 'NONE',  ( -2.660918448318004614, 17.70231371789854435, -12.46528703574811558 ) ) ;
#14814=EDGE_CURVE ( 'NONE', #5242, #21580, #35700, .T. ) ;
#14816=EDGE_LOOP ( 'NONE', ( #33736, #29283, #28409 ) ) ;
#14823=FILL_AREA_STYLE_COLOUR ( '', #5056 ) ;
#14831=CARTESIAN_POINT ( 'NONE',  ( -13.04141134922778456, 14.82731371789855324, 8.927990412390377273 ) ) ;
#14833=CARTESIAN_POINT ( 'NONE',  ( 1.715153634034233487, 129.7226862821014208, 9.534712964251941258 ) ) ;
#14834=CARTESIAN_POINT ( 'NONE',  ( -12.46528703574805697, 40.59768628210144215, -2.660918448318280838 ) ) ;
#14839=CARTESIAN_POINT ( 'NONE',  ( -9.465287035748065847, 22.19768628210144001, -2.064181346179273735 ) ) ;
#14846=CARTESIAN_POINT ( 'NONE',  ( -3.474262827703527901, 87.56481371789857349, 8.843639120294245259 ) ) ;
#14851=CARTESIAN_POINT ( 'NONE',  ( 10.49813415416005213, 93.02731371789856496, -7.228626920338837358 ) ) ;
#14855=CARTESIAN_POINT ( 'NONE',  ( 12.46528703574811558, 66.00231371789855928, -2.660918448318005503 ) ) ;
#14863=CARTESIAN_POINT ( 'NONE',  ( -8.962234695871760692, 48.36018628210145209, 8.715434833791933400 ) ) ;
#14868=CARTESIAN_POINT ( 'NONE',  ( 6.932735513424201024, 101.6523137178985650, -10.69584247140429412 ) ) ;
#14872=CARTESIAN_POINT ( 'NONE',  ( -8.927990412390371944, 72.32731371789854791, -13.04141134922778988 ) ) ;
#14877=CARTESIAN_POINT ( 'NONE',  ( -4.622313124798576922, 97.23518628210145209, -11.61527771782819762 ) ) ;
#14878=CARTESIAN_POINT ( 'NONE',  ( -10.83675517735155047, 41.46018628210145351, -11.08355503943142750 ) ) ;
#14880=DIRECTION ( 'NONE',  ( 0.000000000000000000, 0.9932091452657081376, 0.1163425707149433885 ) ) ;
#14882=CARTESIAN_POINT ( 'NONE',  ( 13.04141134922759804, 64.17268628210143788, 8.927990412390657937 ) ) ;
#14888=CARTESIAN_POINT ( 'NONE',  ( -10.49813415415989581, 41.17268628210144499, -7.228626920339068285 ) ) ;
#14891=CARTESIAN_POINT ( 'NONE',  ( 5.529263428287477744, 6.672686282101436106, -7.954856959092191815 ) ) ;
#14901=CARTESIAN_POINT ( 'NONE',  ( 11.61527771782819940, 44.33518628210145351, -4.622313124798573369 ) ) ;
#14906=CARTESIAN_POINT ( 'NONE',  ( 6.932735513423970097, 92.34768628210144925, 10.69584247140445044 ) ) ;
#14907=CARTESIAN_POINT ( 'NONE',  ( -8.632099005475794229, 23.45231371789854435, 13.23911966647199812 ) ) ;
#14914=CARTESIAN_POINT ( 'NONE',  ( -8.843639120294245259, 16.26481371789853370, -3.474262827703533230 ) ) ;
#14918=PRODUCT_CONTEXT ( 'NONE', #8119, 'mechanical' ) ;
#14921=CARTESIAN_POINT ( 'NONE',  ( -0.1745138560722442889, 137.5898137178985792, -15.50000000000000533 ) ) ;
#14925=CARTESIAN_POINT ( 'NONE',  ( 4.622313124798573369, 46.63518628210145067, 11.61527771782819940 ) ) ;
#14933=CARTESIAN_POINT ( 'NONE',  ( -8.843639120294326972, 58.13518628210145067, 3.474262827703335166 ) ) ;
#14937=CARTESIAN_POINT ( 'NONE',  ( -11.61527771782819940, 94.93518628210145494, 4.622313124798574258 ) ) ;
#14948=CARTESIAN_POINT ( 'NONE',  ( 11.61527771782809637, 103.6648137178985678, 4.622313124798827388 ) ) ;
#14949=CARTESIAN_POINT ( 'NONE',  ( -11.48171059495397373, 114.4851862821014521, -4.944772684328680334 ) ) ;
#14957=CARTESIAN_POINT ( 'NONE',  ( -5.770363421894122880, 78.36481371789855643, 14.38691631536194393 ) ) ;
#14960=CARTESIAN_POINT ( 'NONE',  ( 8.710071997420127943, 100.6851862821014834, 3.796722387233375073 ) ) ;
#14962=CARTESIAN_POINT ( 'NONE',  ( -9.534712964251895073, 80.37731371789853085, -1.715153634034446428 ) ) ;
#14965=CARTESIAN_POINT ( 'NONE',  ( 11.61527771782809637, 48.46481371789855785, 4.622313124798827388 ) ) ;
#14967=CARTESIAN_POINT ( 'NONE',  ( 12.50000000000000355, 100.1101862821014521, 0.1745138560725507937 ) ) ;
#14972=CARTESIAN_POINT ( 'NONE',  ( -14.25334919248782306, 77.68518628210145494, -6.092822981423979378 ) ) ;
#14974=CARTESIAN_POINT ( 'NONE',  ( -4.622313124798576922, 5.235186282101428112, -11.61527771782819762 ) ) ;
#14976=CARTESIAN_POINT ( 'NONE',  ( 3.474262827703335166, 111.0351862821014635, 8.843639120294326972 ) ) ;
#14978=CARTESIAN_POINT ( 'NONE',  ( -15.46528703574804986, 12.99768628210143362, -3.257655550457287497 ) ) ;
#14989=CARTESIAN_POINT ( 'NONE',  ( 8.152565276336593669, 11.95231371789853902, 5.233372021372610483 ) ) ;
#14993=CARTESIAN_POINT ( 'NONE',  ( 8.962234695871567070, 49.03981371789854649, 8.715434833792127023 ) ) ;
#14995=CARTESIAN_POINT ( 'NONE',  ( -7.228626920338836470, 7.927313717898537782, -10.49813415416005213 ) ) ;
#15012=CARTESIAN_POINT ( 'NONE',  ( 13.23911966647199812, 11.95231371789853902, 8.632099005475788900 ) ) ;
#15015=CARTESIAN_POINT ( 'NONE',  ( -5.233372021372430183, 133.7476862821013981, -8.152565276336710909 ) ) ;
#15017=CARTESIAN_POINT ( 'NONE',  ( -4.622313124798576922, 32.83518628210143930, -11.61527771782819762 ) ) ;
#15020=EDGE_LOOP ( 'NONE', ( #33041, #612, #26784, #7733, #30242 ) ) ;
#15022=CARTESIAN_POINT ( 'NONE',  ( -15.53471296425195369, 122.8226862821014294, 2.908627838312118019 ) ) ;
#15024=CARTESIAN_POINT ( 'NONE',  ( -8.710071997420127943, 4.085186282101443744, -3.796722387233380402 ) ) ;
#15032=CARTESIAN_POINT ( 'NONE',  ( 9.500000000000005329, 84.68981371789855928, -0.1745138560723090149 ) ) ;
#15038=CARTESIAN_POINT ( 'NONE',  ( 2.311890736173452421, 91.87731371789855928, -12.53471296425189152 ) ) ;
#15042=CARTESIAN_POINT ( 'NONE',  ( 11.48171059495408208, 74.91481371789855359, -4.944772684328420986 ) ) ;
#15049=CARTESIAN_POINT ( 'NONE',  ( 7.228626920339068285, 34.27268628210144641, -10.49813415415989581 ) ) ;
#15055=CARTESIAN_POINT ( 'NONE',  ( -11.61527771782809282, 80.66481371789856780, -4.622313124798832717 ) ) ;
#15061=CARTESIAN_POINT ( 'NONE',  ( -8.927990412390371944, 81.52731371789856496, -13.04141134922778988 ) ) ;
#15064=CARTESIAN_POINT ( 'NONE',  ( 8.715434833791931624, 92.06018628210145494, 8.962234695871760692 ) ) ;
#15066=CARTESIAN_POINT ( 'NONE',  ( 3.257655550457285720, 42.89768628210143220, -15.46528703574804986 ) ) ;
#15068=CARTESIAN_POINT ( 'NONE',  ( 11.08355503943142750, 52.96018628210144641, -10.83675517735155225 ) ) ;
#15074=CARTESIAN_POINT ( 'NONE',  ( -12.46528703574805697, 31.39768628210144641, -2.660918448318280838 ) ) ;
#15076=CARTESIAN_POINT ( 'NONE',  ( -3.474262827703527901, 142.7648137178985621, 8.843639120294245259 ) ) ;
#15086=CARTESIAN_POINT ( 'NONE',  ( 10.49813415415989581, 54.97268628210144925, 7.228626920339069173 ) ) ;
#15095=CARTESIAN_POINT ( 'NONE',  ( -2.660918448318275509, 102.6976862821014720, 12.46528703574805874 ) ) ;
#15096=CARTESIAN_POINT ( 'NONE',  ( -8.927990412390371944, 26.32731371789854791, -13.04141134922778988 ) ) ;
#15102=CARTESIAN_POINT ( 'NONE',  ( 10.49813415416005213, 139.0273137178985507, -7.228626920338837358 ) ) ;
#15108=CARTESIAN_POINT ( 'NONE',  ( -15.46528703574811736, 135.0023137178985166, 3.257655550456946436 ) ) ;
#15111=CARTESIAN_POINT ( 'NONE',  ( -10.69584247140444866, 48.64768628210144641, 6.932735513423972762 ) ) ;
#15115=CARTESIAN_POINT ( 'NONE',  ( -6.092822981423970496, 102.9851862821014805, 14.25334919248782661 ) ) ;
#15118=CARTESIAN_POINT ( 'NONE',  ( 8.152565276336714462, 62.44768628210144357, -5.233372021372432847 ) ) ;
#15121=CARTESIAN_POINT ( 'NONE',  ( -8.962234695871760692, 94.36018628210145209, 8.715434833791933400 ) ) ;
#15133=CARTESIAN_POINT ( 'NONE',  ( -10.69584247140429412, 108.5523137178985564, -6.932735513424201024 ) ) ;
#15134=CARTESIAN_POINT ( 'NONE',  ( 2.311890736173175753, 111.3226862821014578, 12.53471296425194659 ) ) ;
#15138=CARTESIAN_POINT ( 'NONE',  ( -11.08355503943118592, 72.03981371789855359, -10.83675517735179383 ) ) ;
#15144=CARTESIAN_POINT ( 'NONE',  ( -6.840914352312096547, 103.5601862821014407, 6.594114490232313663 ) ) ;
#15146=CARTESIAN_POINT ( 'NONE',  ( -8.152565276336593669, 71.75231371789854506, -5.233372021372610483 ) ) ;
#15148=CARTESIAN_POINT ( 'NONE',  ( -5.233372021372612259, 115.4523137178985479, 8.152565276336593669 ) ) ;
#15150=CARTESIAN_POINT ( 'NONE',  ( -12.46528703574811558, 52.20231371789855501, 2.660918448318003726 ) ) ;
#15152=CARTESIAN_POINT ( 'NONE',  ( 12.53471296425194836, 99.82268628210144357, -2.311890736173178418 ) ) ;
#15157=CARTESIAN_POINT ( 'NONE',  ( 12.53471296425194836, 136.6226862821014834, -2.311890736173178418 ) ) ;
#15159=CARTESIAN_POINT ( 'NONE',  ( 14.38691631536207538, 90.33518628210144641, -5.770363421893813793 ) ) ;
#15164=CARTESIAN_POINT ( 'NONE',  ( -8.152565276336710909, 122.2476862821014691, 5.233372021372435512 ) ) ;
#15167=CARTESIAN_POINT ( 'NONE',  ( 3.257655550457285720, 6.097686282101443922, -15.46528703574804986 ) ) ;
#15179=CARTESIAN_POINT ( 'NONE',  ( -2.064181346179062349, 26.90231371789854364, -9.465287035748106703 ) ) ;
#15184=CARTESIAN_POINT ( 'NONE',  ( 12.46528703574811558, 20.00231371789855217, -2.660918448318005947 ) ) ;
#15186=CARTESIAN_POINT ( 'NONE',  ( 14.38691631536194393, 131.2648137178985621, 5.770363421894124656 ) ) ;
#15205=CARTESIAN_POINT ( 'NONE',  ( 8.927990412390657937, 135.4726862821014777, -13.04141134922759804 ) ) ;
#15208=CARTESIAN_POINT ( 'NONE',  ( 6.840914352312096547, 126.5601862821014834, -6.594114490232313663 ) ) ;
#15210=CARTESIAN_POINT ( 'NONE',  ( 11.61527771782819940, 25.93518628210143717, -4.622313124798573369 ) ) ;
#15214=CARTESIAN_POINT ( 'NONE',  ( 5.770363421893814682, 120.2351862821014521, 14.38691631536207183 ) ) ;
#15216=CARTESIAN_POINT ( 'NONE',  ( 5.233372021372432847, 9.547686282101452093, 8.152565276336710909 ) ) ;
#15223=CARTESIAN_POINT ( 'NONE',  ( -1.715153634034442431, 78.07731371789854791, 9.534712964251900402 ) ) ;
#15227=CARTESIAN_POINT ( 'NONE',  ( 6.932735513424201024, 101.6523137178985650, -10.69584247140429412 ) ) ;
#15231=CARTESIAN_POINT ( 'NONE',  ( 10.49813415416005213, 56.22731371789854649, -7.228626920338837358 ) ) ;
#15238=CARTESIAN_POINT ( 'NONE',  ( 6.932735513423970097, 46.34768628210145636, 10.69584247140445044 ) ) ;
#15244=CARTESIAN_POINT ( 'NONE',  ( 8.962234695871567070, 76.63981371789856212, 8.715434833792127023 ) ) ;
#15249=CARTESIAN_POINT ( 'NONE',  ( 15.50000000000000533, 66.28981371789855359, -0.1745138560722452326 ) ) ;
#15252=CARTESIAN_POINT ( 'NONE',  ( 2.660918448318279950, 88.89768628210146062, -12.46528703574805697 ) ) ;
#15253=CARTESIAN_POINT ( 'NONE',  ( 15.53471296425195369, 26.22268628210144925, -2.908627838312120684 ) ) ;
#15256=CARTESIAN_POINT ( 'NONE',  ( 15.53471296425195369, 44.62268628210144783, -2.908627838312120684 ) ) ;
#15262=CARTESIAN_POINT ( 'NONE',  ( -2.311890736173176641, 14.72268628210143859, -12.53471296425194836 ) ) ;
#15264=CARTESIAN_POINT ( 'NONE',  ( 6.840914352311949109, 122.6398137178985479, 6.594114490232462877 ) ) ;
#15275=CARTESIAN_POINT ( 'NONE',  ( 12.53471296425194659, 53.82268628210145067, -2.311890736173178418 ) ) ;
#15280=LINE ( 'NONE', #35549, #7022 ) ;
#15283=CARTESIAN_POINT ( 'NONE',  ( 12.50000000000000355, 100.1101862821014521, 0.1745138560725507937 ) ) ;
#15284=CARTESIAN_POINT ( 'NONE',  ( 10.83675517735179206, 19.13981371789855146, -11.08355503943118769 ) ) ;
#15292=CARTESIAN_POINT ( 'NONE',  ( 8.962234695871567070, 131.8398137178985792, 8.715434833792127023 ) ) ;
#15298=CARTESIAN_POINT ( 'NONE',  ( -2.908627838312453306, 114.8773137178985735, 15.53471296425188797 ) ) ;
#15301=CARTESIAN_POINT ( 'NONE',  ( -11.48171059495397373, 31.68518628210144428, -4.944772684328680334 ) ) ;
#15306=CARTESIAN_POINT ( 'NONE',  ( -10.83675517735155047, 96.66018628210144925, -11.08355503943142750 ) ) ;
#15309=CARTESIAN_POINT ( 'NONE',  ( -9.465287035748065847, 49.79768628210144499, -2.064181346179273735 ) ) ;
#15312=CARTESIAN_POINT ( 'NONE',  ( -10.69584247140444866, 85.44768628210144357, 6.932735513423972762 ) ) ;
#15326=CARTESIAN_POINT ( 'NONE',  ( 2.311890736173452865, 101.0773137178985621, -12.53471296425189152 ) ) ;
#15327=CARTESIAN_POINT ( 'NONE',  ( -11.48171059495397373, 96.08518628210146062, -4.944772684328680334 ) ) ;
#15332=CARTESIAN_POINT ( 'NONE',  ( -13.04141134922778456, 70.02731371789855075, 8.927990412390377273 ) ) ;
#15335=CARTESIAN_POINT ( 'NONE',  ( -7.954856959092191815, 96.37268628210144072, -5.529263428287477744 ) ) ;
#15338=CARTESIAN_POINT ( 'NONE',  ( 3.474262827703532341, 55.36481371789856354, -8.843639120294245259 ) ) ;
#15341=CARTESIAN_POINT ( 'NONE',  ( 7.954856959092311719, 111.4273137178985422, -5.529263428287300108 ) ) ;
#15342=CARTESIAN_POINT ( 'NONE',  ( 6.932735513424201024, 28.05231371789855643, -10.69584247140429412 ) ) ;
#15344=CARTESIAN_POINT ( 'NONE',  ( -8.715434833791929847, 96.66018628210146346, -8.962234695871762469 ) ) ;
#15349=CARTESIAN_POINT ( 'NONE',  ( 5.770363421893814682, 83.43518628210145494, 14.38691631536207183 ) ) ;
#15353=CARTESIAN_POINT ( 'NONE',  ( 6.840914352312096547, 108.1601862821014635, -6.594114490232313663 ) ) ;
#15355=CARTESIAN_POINT ( 'NONE',  ( 0.1745138560725515708, 134.6101862821014663, -12.50000000000000355 ) ) ;
#15369=CARTESIAN_POINT ( 'NONE',  ( -9.465287035748106703, 24.60231371789854649, 2.064181346179061460 ) ) ;
#15372=VERTEX_POINT ( 'NONE', #7753 ) ;
#15375=CARTESIAN_POINT ( 'NONE',  ( 11.48171059495408208, 19.71481371789854364, -4.944772684328420986 ) ) ;
#15377=CARTESIAN_POINT ( 'NONE',  ( -6.092822981423666739, 137.0148137178985621, -14.25334919248795096 ) ) ;
#15383=CARTESIAN_POINT ( 'NONE',  ( 12.50000000000000355, 136.9101862821014777, 0.1745138560725507937 ) ) ;
#15389=SHAPE_REPRESENTATION_RELATIONSHIP ( 'NONE' , 'NONE' ,  #36285, #18760 ) ;
#15396=CARTESIAN_POINT ( 'NONE',  ( 2.908627838312118019, 138.9226862821014663, 15.53471296425195369 ) ) ;
#15400=CARTESIAN_POINT ( 'NONE',  ( -8.710071997420127943, 123.6851862821014549, -3.796722387233380402 ) ) ;
#15403=CARTESIAN_POINT ( 'NONE',  ( 12.46528703574805874, 35.99768628210144072, 2.660918448318279950 ) ) ;
#15408=CARTESIAN_POINT ( 'NONE',  ( -11.08355503943142573, 121.9601862821014606, 10.83675517735155402 ) ) ;
#15410=CARTESIAN_POINT ( 'NONE',  ( 2.064181346179272847, 6.097686282101443922, -9.465287035748065847 ) ) ;
#15416=CARTESIAN_POINT ( 'NONE',  ( -5.233372021372612259, 78.65231371789856496, 8.152565276336593669 ) ) ;
#15420=CARTESIAN_POINT ( 'NONE',  ( -0.1745138560722763466, 73.18981371789855928, -12.50000000000000355 ) ) ;
#15422=CARTESIAN_POINT ( 'NONE',  ( -10.08800066309955490, 142.9999999999999147, 9.061245623615871381 ) ) ;
#15424=CARTESIAN_POINT ( 'NONE',  ( 8.962234695871567070, 39.83981371789855075, 8.715434833792127023 ) ) ;
#15430=CARTESIAN_POINT ( 'NONE',  ( 2.311890736173175753, 28.52268628210144641, 12.53471296425194836 ) ) ;
#15435=CARTESIAN_POINT ( 'NONE',  ( -2.660918448318004614, 91.30231371789857064, -12.46528703574811558 ) ) ;
#15440=CARTESIAN_POINT ( 'NONE',  ( -5.770363421894122880, 59.96481371789855075, 14.38691631536194393 ) ) ;
#15443=CARTESIAN_POINT ( 'NONE',  ( -11.61527771782819940, 85.73518628210143788, 4.622313124798574258 ) ) ;
#15444=CARTESIAN_POINT ( 'NONE',  ( -15.50000000000000533, 21.91018628210143859, -0.1745138560725808530 ) ) ;
#15448=CARTESIAN_POINT ( 'NONE',  ( 14.38691631536207538, 44.33518628210144641, -5.770363421893813793 ) ) ;
#15453=CARTESIAN_POINT ( 'NONE',  ( 12.50000000000000355, 26.51018628210144357, 0.1745138560725507937 ) ) ;
#15456=CARTESIAN_POINT ( 'NONE',  ( 9.465287035748106703, 139.6023137178985394, -2.064181346179063237 ) ) ;
#15461=CARTESIAN_POINT ( 'NONE',  ( -10.49813415416004858, 134.4273137178985564, 7.228626920338840023 ) ) ;
#15466=CARTESIAN_POINT ( 'NONE',  ( -10.69584247140444866, 48.64768628210144641, 6.932735513423972762 ) ) ;
#15474=CARTESIAN_POINT ( 'NONE',  ( 8.715434833791931624, 101.2601862821014578, 8.962234695871760692 ) ) ;
#15475=CARTESIAN_POINT ( 'NONE',  ( 15.53471296425188797, 29.77731371789854364, 2.908627838312457747 ) ) ;
#15481=CARTESIAN_POINT ( 'NONE',  ( 9.534712964251900402, 11.37731371789854506, 1.715153634034445540 ) ) ;
#15488=CARTESIAN_POINT ( 'NONE',  ( -15.46528703574811736, 107.4023137178985650, 3.257655550456946436 ) ) ;
#15491=CARTESIAN_POINT ( 'NONE',  ( -4.944772684328673229, 29.38518628210144712, 11.48171059495397728 ) ) ;
#15495=CARTESIAN_POINT ( 'NONE',  ( 14.38691631536207538, 108.7351862821014663, -5.770363421893813793 ) ) ;
#15499=CARTESIAN_POINT ( 'NONE',  ( -3.796722387233375073, 66.18518628210145494, 8.710071997420127943 ) ) ;
#15504=CARTESIAN_POINT ( 'NONE',  ( 11.48171059495397728, 73.08518628210144641, 4.944772684328674117 ) ) ;
#15507=CARTESIAN_POINT ( 'NONE',  ( 8.152565276336714462, 44.04768628210143788, -5.233372021372432847 ) ) ;
#15518=CARTESIAN_POINT ( 'NONE',  ( -12.46528703574811558, 98.20231371789856212, 2.660918448318003726 ) ) ;
#15519=CARTESIAN_POINT ( 'NONE',  ( 10.49813415415989581, 100.9726862821014635, 7.228626920339069173 ) ) ;
#15524=CARTESIAN_POINT ( 'NONE',  ( 5.770363421894130873, 73.76481371789856212, -14.38691631536193860 ) ) ;
#15527=CARTESIAN_POINT ( 'NONE',  ( 0.1745138560725194299, 107.0101862821014578, -9.500000000000005329 ) ) ;
#15529=CARTESIAN_POINT ( 'NONE',  ( -8.710071997420207879, 51.91481371789856070, 3.796722387233182339 ) ) ;
#15531=CARTESIAN_POINT ( 'NONE',  ( -3.474262827703527901, 115.1648137178985678, 8.843639120294245259 ) ) ;
#15533=CARTESIAN_POINT ( 'NONE',  ( -11.48171059495408208, 24.31481371789855217, 4.944772684328421875 ) ) ;
#15535=CARTESIAN_POINT ( 'NONE',  ( 8.715434833791931624, 73.66018628210144925, 8.962234695871760692 ) ) ;
#15543=CARTESIAN_POINT ( 'NONE',  ( -6.840914352312096547, 112.7601862821014720, 6.594114490232313663 ) ) ;
#15545=CARTESIAN_POINT ( 'NONE',  ( -12.46528703574805697, 132.5976862821014777, -2.660918448318280838 ) ) ;
#15557=CARTESIAN_POINT ( 'NONE',  ( -9.534712964251895073, 15.97731371789853405, -1.715153634034446428 ) ) ;
#15562=CARTESIAN_POINT ( 'NONE',  ( -4.944772684328424539, 26.61481371789854578, -11.48171059495408031 ) ) ;
#15564=CARTESIAN_POINT ( 'NONE',  ( -3.257655550456946880, 137.3023137178985564, -15.46528703574811736 ) ) ;
#15571=CARTESIAN_POINT ( 'NONE',  ( -2.311890736173176641, 134.3226862821014436, -12.53471296425194836 ) ) ;
#15579=CARTESIAN_POINT ( 'NONE',  ( 4.622313124798573369, 129.4351862821014549, 11.61527771782819940 ) ) ;
#15583=CARTESIAN_POINT ( 'NONE',  ( 15.53471296425188797, 11.37731371789854506, 2.908627838312457747 ) ) ;
#15585=CARTESIAN_POINT ( 'NONE',  ( 5.233372021372432847, 119.9476862821014294, 8.152565276336710909 ) ) ;
#15588=CARTESIAN_POINT ( 'NONE',  ( 4.622313124798573369, 37.43518628210144783, 11.61527771782819940 ) ) ;
#15592=CARTESIAN_POINT ( 'NONE',  ( -10.83675517735155047, 124.2601862821014578, -11.08355503943142750 ) ) ;
#15594=CARTESIAN_POINT ( 'NONE',  ( 1.715153634034233487, 10.12268628210144428, 9.534712964251941258 ) ) ;
#15601=CARTESIAN_POINT ( 'NONE',  ( -0.1745138560723084320, 82.38981371789856212, -9.500000000000005329 ) ) ;
#15604=CARTESIAN_POINT ( 'NONE',  ( 12.50000000000000355, 75.48981371789855643, -0.1745138560722771515 ) ) ;
#15608=CARTESIAN_POINT ( 'NONE',  ( -10.49813415416004858, 42.42731371789855643, 7.228626920338839135 ) ) ;
#15613=CARTESIAN_POINT ( 'NONE',  ( 0.1745138560725515708, 15.01018628210143468, -12.50000000000000355 ) ) ;
#15619=CARTESIAN_POINT ( 'NONE',  ( 11.48171059495408208, 84.11481371789855643, -4.944772684328420986 ) ) ;
#15625=CARTESIAN_POINT ( 'NONE',  ( -10.83675517735179028, 51.33981371789855785, 11.08355503943118947 ) ) ;
#15628=CARTESIAN_POINT ( 'NONE',  ( 11.48171059495397728, 91.48518628210145209, 4.944772684328674117 ) ) ;
#15629=CARTESIAN_POINT ( 'NONE',  ( -15.46528703574804986, 22.19768628210144001, -3.257655550457287497 ) ) ;
#15635=CARTESIAN_POINT ( 'NONE',  ( -2.908627838312119351, 42.32268628210145067, -15.53471296425195369 ) ) ;
#15642=CARTESIAN_POINT ( 'NONE',  ( -8.715434833791929847, 23.06018628210145138, -8.962234695871762469 ) ) ;
#15644=CARTESIAN_POINT ( 'NONE',  ( 3.474262827703532341, 138.1648137178985678, -8.843639120294245259 ) ) ;
#15650=CARTESIAN_POINT ( 'NONE',  ( 12.46528703574811558, 130.4023137178985792, -2.660918448318005947 ) ) ;
#15656=CARTESIAN_POINT ( 'NONE',  ( -10.49813415415989404, 50.37268628210145494, -7.228626920339069173 ) ) ;
#15664=CARTESIAN_POINT ( 'NONE',  ( 8.715434833791931624, 73.66018628210144925, 8.962234695871760692 ) ) ;
#15665=CARTESIAN_POINT ( 'NONE',  ( -5.770363421894122880, 13.96481371789853831, 14.38691631536194393 ) ) ;
#15671=CARTESIAN_POINT ( 'NONE',  ( 8.710071997420211432, 10.51481371789855679, -3.796722387233181895 ) ) ;
#15678=CARTESIAN_POINT ( 'NONE',  ( -0.1745138560722442889, 109.9898137178985706, -15.50000000000000533 ) ) ;
#15682=CARTESIAN_POINT ( 'NONE',  ( -11.61527771782819940, 21.33518628210144641, 4.622313124798574258 ) ) ;
#15686=CARTESIAN_POINT ( 'NONE',  ( -13.04141134922759804, 105.5726862821014294, -8.927990412390657937 ) ) ;
#15690=CARTESIAN_POINT ( 'NONE',  ( -2.064181346179269738, 38.29768628210144499, 9.465287035748067623 ) ) ;
#15694=CARTESIAN_POINT ( 'NONE',  ( 2.660918448318279950, 79.69768628210144357, -12.46528703574805697 ) ) ;
#15697=CARTESIAN_POINT ( 'NONE',  ( -6.594114490232312775, 50.66018628210144925, -6.840914352312096547 ) ) ;
#15707=CARTESIAN_POINT ( 'NONE',  ( 12.53471296425189330, 94.17731371789857064, 2.311890736173451977 ) ) ;
#15708=CARTESIAN_POINT ( 'NONE',  ( -6.932735513423968321, 106.1476862821014606, -10.69584247140445221 ) ) ;
#15713=CARTESIAN_POINT ( 'NONE',  ( -3.257655550456946880, 72.90231371789855075, -15.46528703574811736 ) ) ;
#15716=CARTESIAN_POINT ( 'NONE',  ( -3.796722387233375073, 93.78518628210144925, 8.710071997420127943 ) ) ;
#15719=CARTESIAN_POINT ( 'NONE',  ( -6.594114490232462877, 51.33981371789855785, 6.840914352311949109 ) ) ;
#15721=CARTESIAN_POINT ( 'NONE',  ( 6.594114490232462877, 111.1398137178985621, -6.840914352311949109 ) ) ;
#15723=CARTESIAN_POINT ( 'NONE',  ( 8.962234695871567070, 21.43981371789854862, 8.715434833792127023 ) ) ;
#15724=CARTESIAN_POINT ( 'NONE',  ( -10.49813415415989581, 87.17268628210143788, -7.228626920339068285 ) ) ;
#15730=FACE_OUTER_BOUND ( 'NONE', #28677, .T. ) ;
#15732=CARTESIAN_POINT ( 'NONE',  ( -7.954856959092191815, 96.37268628210144072, -5.529263428287477744 ) ) ;
#15734=CARTESIAN_POINT ( 'NONE',  ( 12.50000000000000355, 136.9101862821014777, 0.1745138560725507937 ) ) ;
#15735=CARTESIAN_POINT ( 'NONE',  ( -6.589905998207248317, 143.0000000000000284, 10.14935392281090287 ) ) ;
#15746=CARTESIAN_POINT ( 'NONE',  ( 3.474262827703532341, 18.56481371789855928, -8.843639120294245259 ) ) ;
#15752=CARTESIAN_POINT ( 'NONE',  ( -0.1745138560722763466, 27.18981371789855217, -12.50000000000000355 ) ) ;
#15754=CARTESIAN_POINT ( 'NONE',  ( -8.927990412390371944, 127.5273137178985792, -13.04141134922778988 ) ) ;
#15763=CARTESIAN_POINT ( 'NONE',  ( 11.48171059495397728, 137.4851862821014663, 4.944772684328674117 ) ) ;
#15771=CARTESIAN_POINT ( 'NONE',  ( -2.311890736173176641, 134.3226862821014436, -12.53471296425194836 ) ) ;
#15776=CARTESIAN_POINT ( 'NONE',  ( 10.83675517735155225, 138.0601862821014549, 11.08355503943142573 ) ) ;
#15778=CARTESIAN_POINT ( 'NONE',  ( -8.152565276336710909, 113.0476862821014663, 5.233372021372435512 ) ) ;
#15780=CARTESIAN_POINT ( 'NONE',  ( 8.962234695871762469, 25.36018628210144499, -8.715434833791931624 ) ) ;
#15785=CARTESIAN_POINT ( 'NONE',  ( 13.23911966647218996, 126.8476862821014635, -8.632099005475504683 ) ) ;
#15787=CARTESIAN_POINT ( 'NONE',  ( -7.954856959092309943, 143.6273137178985451, 5.529263428287300108 ) ) ;
#15793=CARTESIAN_POINT ( 'NONE',  ( -5.233372021372612259, 69.45231371789853370, 8.152565276336593669 ) ) ;
#15796=CARTESIAN_POINT ( 'NONE',  ( -12.46528703574811558, 79.80231371789855643, 2.660918448318004170 ) ) ;
#15798=CARTESIAN_POINT ( 'NONE',  ( -6.543039160116403075, 143.0000000000000284, 10.81689977700826866 ) ) ;
#15800=CARTESIAN_POINT ( 'NONE',  ( 4.622313124798831829, 55.36481371789855643, -11.61527771782809282 ) ) ;
#15804=CARTESIAN_POINT ( 'NONE',  ( 8.962234695871762469, 16.16018628210144570, -8.715434833791931624 ) ) ;
#15809=CARTESIAN_POINT ( 'NONE',  ( -2.311890736173448424, 78.07731371789856212, 12.53471296425189330 ) ) ;
#15814=CARTESIAN_POINT ( 'NONE',  ( -6.092822981423666739, 63.41481371789855359, -14.25334919248795096 ) ) ;
#15817=CARTESIAN_POINT ( 'NONE',  ( 2.311890736173175753, 92.92268628210145209, 12.53471296425194836 ) ) ;
#15818=CARTESIAN_POINT ( 'NONE',  ( 15.50000000000000533, 26.51018628210144001, 0.1745138560725827404 ) ) ;
#15822=CARTESIAN_POINT ( 'NONE',  ( 10.83675517735155225, 46.06018628210144072, 11.08355503943142573 ) ) ;
#15829=CARTESIAN_POINT ( 'NONE',  ( -2.660918448318275509, 19.89768628210143575, 12.46528703574805874 ) ) ;
#15832=CARTESIAN_POINT ( 'NONE',  ( 8.152565276336593669, 131.5523137178985564, 5.233372021372610483 ) ) ;
#15836=CARTESIAN_POINT ( 'NONE',  ( -4.944772684328424539, 127.8148137178985735, -11.48171059495408031 ) ) ;
#15842=CARTESIAN_POINT ( 'NONE',  ( -4.944772684328673229, 38.58518628210144641, 11.48171059495397728 ) ) ;
#15851=CARTESIAN_POINT ( 'NONE',  ( -12.50000000000000355, 77.11018628210145209, -0.1745138560725492671 ) ) ;
#15852=CARTESIAN_POINT ( 'NONE',  ( 15.50000000000000533, 11.08981371789854897, -0.1745138560722452326 ) ) ;
#15860=CARTESIAN_POINT ( 'NONE',  ( -12.50000000000000355, 144.4898137178985564, 0.1745138560722786503 ) ) ;
#15868=CARTESIAN_POINT ( 'NONE',  ( -13.23911966647199812, 108.5523137178985422, -8.632099005475788900 ) ) ;
#15874=CARTESIAN_POINT ( 'NONE',  ( 6.092822981423978490, 98.38518628210145778, -14.25334919248782306 ) ) ;
#15879=CARTESIAN_POINT ( 'NONE',  ( 0.1745138560725194299, 42.61018628210144499, -9.500000000000005329 ) ) ;
#15883=CARTESIAN_POINT ( 'NONE',  ( 10.49813415415989581, 82.57268628210145778, 7.228626920339068285 ) ) ;
#15886=CARTESIAN_POINT ( 'NONE',  ( -5.233372021372430183, 41.74768628210143362, -8.152565276336710909 ) ) ;
#15896=CARTESIAN_POINT ( 'NONE',  ( -11.61527771782809282, 89.86481371789855643, -4.622313124798832717 ) ) ;
#15897=CARTESIAN_POINT ( 'NONE',  ( -12.46528703574805874, 104.9976862821014549, -2.660918448318280838 ) ) ;
#15903=CARTESIAN_POINT ( 'NONE',  ( -13.04141134922778456, 51.62731371789855928, 8.927990412390377273 ) ) ;
#15909=CARTESIAN_POINT ( 'NONE',  ( 6.840914352311949109, 49.03981371789855359, 6.594114490232462877 ) ) ;
#15911=CARTESIAN_POINT ( 'NONE',  ( -7.954856959092309943, 116.0273137178985792, 5.529263428287300108 ) ) ;
#15913=CARTESIAN_POINT ( 'NONE',  ( -7.228626920338836470, 35.52731371789855075, -10.49813415416005213 ) ) ;
#15914=CARTESIAN_POINT ( 'NONE',  ( -2.311890736173176641, 88.32268628210144357, -12.53471296425194836 ) ) ;
#15923=CARTESIAN_POINT ( 'NONE',  ( 5.529263428287477744, 89.47268628210143504, -7.954856959092191815 ) ) ;
#15925=CARTESIAN_POINT ( 'NONE',  ( -7.228626920339069173, 140.0726862821014720, 10.49813415415989581 ) ) ;
#15938=CARTESIAN_POINT ( 'NONE',  ( 8.710071997420211432, 10.51481371789855679, -3.796722387233181895 ) ) ;
#15943=CARTESIAN_POINT ( 'NONE',  ( -2.311890736173447980, 32.07731371789855501, 12.53471296425189330 ) ) ;
#15945=CARTESIAN_POINT ( 'NONE',  ( 6.092822981423662299, 123.2148137178985792, 14.25334919248795096 ) ) ;
#15952=CARTESIAN_POINT ( 'NONE',  ( -10.69584247140444866, 140.6476862821014890, 6.932735513423972762 ) ) ;
#15963=CARTESIAN_POINT ( 'NONE',  ( 15.50000000000000533, 127.7101862821014606, 0.1745138560725827404 ) ) ;
#15965=CARTESIAN_POINT ( 'NONE',  ( -6.594114490232312775, 115.0601862821014691, -6.840914352312096547 ) ) ;
#15968=CARTESIAN_POINT ( 'NONE',  ( 11.61527771782819940, 16.73518628210143788, -4.622313124798573369 ) ) ;
#15972=CARTESIAN_POINT ( 'NONE',  ( -3.796722387233375073, 84.58518628210146062, 8.710071997420127943 ) ) ;
#15975=CARTESIAN_POINT ( 'NONE',  ( 3.796722387233182339, 132.4148137178985678, 8.710071997420207879 ) ) ;
#15984=CARTESIAN_POINT ( 'NONE',  ( -0.1745138560723084320, 73.18981371789854506, -9.500000000000005329 ) ) ;
#15987=CARTESIAN_POINT ( 'NONE',  ( -8.715434833792127023, 88.13981371789856212, 8.962234695871568846 ) ) ;
#15989=CARTESIAN_POINT ( 'NONE',  ( -11.68933346642354998, 143.0000000000000000, 7.290916064140882114 ) ) ;
#15991=CARTESIAN_POINT ( 'NONE',  ( 12.46528703574811558, 47.60231371789855359, -2.660918448318005503 ) ) ;
#15996=CARTESIAN_POINT ( 'NONE',  ( 11.61527771782819940, 25.93518628210143717, -4.622313124798573369 ) ) ;
#16001=CARTESIAN_POINT ( 'NONE',  ( -10.69584247140429412, 62.55231371789856354, -6.932735513424201024 ) ) ;
#16007=CARTESIAN_POINT ( 'NONE',  ( 0.1745138560722461762, 40.98981371789854933, 15.50000000000000533 ) ) ;
#16010=CARTESIAN_POINT ( 'NONE',  ( -0.1745138560725500443, 74.81018628210145494, 12.50000000000000355 ) ) ;
#16011=CARTESIAN_POINT ( 'NONE',  ( -5.770363421893818234, 32.83518628210143930, -14.38691631536207005 ) ) ;
#16015=CARTESIAN_POINT ( 'NONE',  ( 14.25334919248782661, 27.08518628210144996, 6.092822981423971385 ) ) ;
#16022=CARTESIAN_POINT ( 'NONE',  ( 9.534712964251900402, 130.9773137178985394, 1.715153634034445540 ) ) ;
#16027=CARTESIAN_POINT ( 'NONE',  ( 12.46528703574811558, 139.6023137178985678, -2.660918448318005947 ) ) ;
#16033=CARTESIAN_POINT ( 'NONE',  ( -2.660918448318275509, 29.09768628210144925, 12.46528703574805874 ) ) ;
#16041=CARTESIAN_POINT ( 'NONE',  ( 12.46528703574805874, 81.99768628210146915, 2.660918448318279950 ) ) ;
#16042=CARTESIAN_POINT ( 'NONE',  ( -11.08355503943118592, 7.639813717898540801, -10.83675517735179383 ) ) ;
#16047=CARTESIAN_POINT ( 'NONE',  ( 0.000000000000000000, 0.000000000000000000, 0.000000000000000000 ) ) ;
#16049=CARTESIAN_POINT ( 'NONE',  ( -2.660918448318004614, 128.1023137178985678, -12.46528703574811558 ) ) ;
#16055=CARTESIAN_POINT ( 'NONE',  ( -14.38691631536193860, 108.2648137178985621, -5.770363421894132649 ) ) ;
#16059=CARTESIAN_POINT ( 'NONE',  ( 8.715434833791931624, 128.8601862821014663, 8.962234695871760692 ) ) ;
#16060=CARTESIAN_POINT ( 'NONE',  ( 3.257655550457285720, 79.69768628210141515, -15.46528703574804986 ) ) ;
#16064=CARTESIAN_POINT ( 'NONE',  ( -14.38691631536207183, 85.73518628210145209, 5.770363421893814682 ) ) ;
#16067=CARTESIAN_POINT ( 'NONE',  ( -2.064181346179269738, 47.49768628210145494, 9.465287035748067623 ) ) ;
#16071=CARTESIAN_POINT ( 'NONE',  ( -12.50000000000000355, 67.91018628210144925, -0.1745138560725492671 ) ) ;
#16074=CARTESIAN_POINT ( 'NONE',  ( 5.233372021372432847, 37.14768628210143220, 8.152565276336710909 ) ) ;
#16083=CARTESIAN_POINT ( 'NONE',  ( 6.932735513424201024, 92.45231371789856212, -10.69584247140429412 ) ) ;
#16084=CARTESIAN_POINT ( 'NONE',  ( -8.715434833791929847, 78.26018628210144357, -8.962234695871762469 ) ) ;
#16088=CARTESIAN_POINT ( 'NONE',  ( 13.04141134922778988, 56.22731371789854649, -8.927990412390371944 ) ) ;
#16094=CARTESIAN_POINT ( 'NONE',  ( 9.534712964251900402, 66.57731371789853370, 1.715153634034445540 ) ) ;
#16097=CARTESIAN_POINT ( 'NONE',  ( -6.594114490232462877, 97.33981371789856496, 6.840914352311949109 ) ) ;
#16099=CARTESIAN_POINT ( 'NONE',  ( 4.622313124798831829, 27.76481371789854435, -11.61527771782809282 ) ) ;
#16101=CARTESIAN_POINT ( 'NONE',  ( -11.61527771782819940, 76.53518628210146346, 4.622313124798574258 ) ) ;
#16109=CARTESIAN_POINT ( 'NONE',  ( 6.594114490232313663, 92.06018628210145494, 6.840914352312096547 ) ) ;
#16111=CARTESIAN_POINT ( 'NONE',  ( -10.69584247140444866, 140.6476862821014890, 6.932735513423972762 ) ) ;
#16123=CARTESIAN_POINT ( 'NONE',  ( 8.962234695871567070, 141.0398137178985678, 8.715434833792127023 ) ) ;
#16129=CARTESIAN_POINT ( 'NONE',  ( 12.50000000000000355, 11.08981371789855075, -0.1745138560722771515 ) ) ;
#16131=CARTESIAN_POINT ( 'NONE',  ( -3.257655550456946880, 109.7023137178985479, -15.46528703574811736 ) ) ;
#16136=CARTESIAN_POINT ( 'NONE',  ( -2.311890736173176641, 125.1226862821014549, -12.53471296425194836 ) ) ;
#16146=CARTESIAN_POINT ( 'NONE',  ( 12.46528703574805874, 137.1976862821014720, 2.660918448318279950 ) ) ;
#16151=CARTESIAN_POINT ( 'NONE',  ( 8.927990412390657937, 117.0726862821014294, -13.04141134922759804 ) ) ;
#16153=CARTESIAN_POINT ( 'NONE',  ( 1.715153634034233487, 111.3226862821014578, 9.534712964251941258 ) ) ;
#16155=CARTESIAN_POINT ( 'NONE',  ( -4.622313124798576922, 14.43518628210144250, -11.61527771782819762 ) ) ;
#16159=CARTESIAN_POINT ( 'NONE',  ( -9.534712964251941258, 76.82268628210144357, 1.715153634034234154 ) ) ;
#16161=CARTESIAN_POINT ( 'NONE',  ( 0.1745138560723095977, 123.7898137178985678, 9.500000000000005329 ) ) ;
#16168=CARTESIAN_POINT ( 'NONE',  ( 9.534712964251900402, 57.37731371789855928, 1.715153634034445540 ) ) ;
#16169=ORIENTED_EDGE ( 'NONE', *, *, #6580, .T. ) ;
#16171=CARTESIAN_POINT ( 'NONE',  ( 12.53471296425189330, 75.77731371789856496, 2.311890736173451533 ) ) ;
#16175=CARTESIAN_POINT ( 'NONE',  ( -2.311890736173448424, 22.87731371789854151, 12.53471296425189330 ) ) ;
#16180=CARTESIAN_POINT ( 'NONE',  ( -4.944772684328673229, 20.18518628210144783, 11.48171059495397728 ) ) ;
#16184=CARTESIAN_POINT ( 'NONE',  ( 8.962234695871567070, 58.23981371789854933, 8.715434833792127023 ) ) ;
#16191=CARTESIAN_POINT ( 'NONE',  ( -15.46528703574811736, 33.80231371789854222, 3.257655550456946436 ) ) ;
#16194=CARTESIAN_POINT ( 'NONE',  ( 8.715434833791931624, 64.46018628210146062, 8.962234695871760692 ) ) ;
#16195=CARTESIAN_POINT ( 'NONE',  ( 10.83675517735155225, 9.260186282101427580, 11.08355503943142573 ) ) ;
#16199=CARTESIAN_POINT ( 'NONE',  ( -15.50000000000000533, 21.91018628210143859, -0.1745138560725808530 ) ) ;
#16206=CARTESIAN_POINT ( 'NONE',  ( 2.660918448318279950, 6.097686282101443922, -12.46528703574805697 ) ) ;
#16208=CARTESIAN_POINT ( 'NONE',  ( 9.534712964251900402, 103.3773137178985451, 1.715153634034445540 ) ) ;
#16212=CARTESIAN_POINT ( 'NONE',  ( 8.962234695871567070, 141.0398137178985678, 8.715434833792127023 ) ) ;
#16218=CARTESIAN_POINT ( 'NONE',  ( -11.61527771782819940, 30.53518628210144570, 4.622313124798574258 ) ) ;
#16226=CARTESIAN_POINT ( 'NONE',  ( -4.622313124798576922, 69.63518628210145778, -11.61527771782819762 ) ) ;
#16227=CARTESIAN_POINT ( 'NONE',  ( 15.46528703574811736, 10.80231371789855466, -3.257655550456947768 ) ) ;
#16235=CARTESIAN_POINT ( 'NONE',  ( -12.53471296425189152, 126.3773137178985593, -2.311890736173453753 ) ) ;
#16242=CARTESIAN_POINT ( 'NONE',  ( 0.1745138560722461762, 96.18981371789855928, 15.50000000000000533 ) ) ;
#16246=CARTESIAN_POINT ( 'NONE',  ( 12.46528703574805874, 127.9976862821014407, 2.660918448318279950 ) ) ;
#16247=CARTESIAN_POINT ( 'NONE',  ( -6.092822981423970496, 75.38518628210142936, 14.25334919248782661 ) ) ;
#16250=CARTESIAN_POINT ( 'NONE',  ( 2.908627838312118019, 92.92268628210145209, 15.53471296425195369 ) ) ;
#16253=CARTESIAN_POINT ( 'NONE',  ( -8.710071997420127943, 31.68518628210144428, -3.796722387233380402 ) ) ;
#16256=CARTESIAN_POINT ( 'NONE',  ( -12.46528703574805697, 49.79768628210145209, -2.660918448318280838 ) ) ;
#16260=CARTESIAN_POINT ( 'NONE',  ( 8.152565276336714462, 53.24768628210144783, -5.233372021372432847 ) ) ;
#16270=CARTESIAN_POINT ( 'NONE',  ( 8.962234695871567070, 85.83981371789856496, 8.715434833792127023 ) ) ;
#16271=CARTESIAN_POINT ( 'NONE',  ( 2.660918448318279950, 88.89768628210146062, -12.46528703574805874 ) ) ;
#16277=CARTESIAN_POINT ( 'NONE',  ( -2.908627838312453306, 59.67731371789855643, 15.53471296425188797 ) ) ;
#16281=CARTESIAN_POINT ( 'NONE',  ( -8.710071997420207879, 42.71481371789855075, 3.796722387233182339 ) ) ;
#16284=CARTESIAN_POINT ( 'NONE',  ( 8.152565276336593669, 94.75231371789854506, 5.233372021372610483 ) ) ;
#16286=CARTESIAN_POINT ( 'NONE',  ( 12.50000000000000355, 11.08981371789855075, -0.1745138560722771515 ) ) ;
#16287=CARTESIAN_POINT ( 'NONE',  ( -0.1745138560725500443, 74.81018628210145494, 12.50000000000000355 ) ) ;
#16294=CARTESIAN_POINT ( 'NONE',  ( 8.152565276336714462, 99.24768628210145494, -5.233372021372432847 ) ) ;
#16296=CARTESIAN_POINT ( 'NONE',  ( -12.50000000000000355, 104.7101862821014606, -0.1745138560725492671 ) ) ;
#16297=CARTESIAN_POINT ( 'NONE',  ( -8.655134159629936264, 143.0000000000000284, 7.486361052592569010 ) ) ;
#16309=CARTESIAN_POINT ( 'NONE',  ( -11.48171059495408208, 143.9148137178985678, 4.944772684328421875 ) ) ;
#16310=CARTESIAN_POINT ( 'NONE',  ( -8.962234695871760692, 140.3601862821014379, 8.715434833791933400 ) ) ;
#16316=CARTESIAN_POINT ( 'NONE',  ( -10.83675517735179028, 106.5398137178985536, 11.08355503943118947 ) ) ;
#16322=CARTESIAN_POINT ( 'NONE',  ( 8.715434833791931624, 119.6601862821014493, 8.962234695871760692 ) ) ;
#16329=CARTESIAN_POINT ( 'NONE',  ( -11.61527771782819940, 140.9351862821014834, 4.622313124798574258 ) ) ;
#16335=CARTESIAN_POINT ( 'NONE',  ( 8.632099005475504683, 119.9476862821014294, 13.23911966647218996 ) ) ;
#16337=CARTESIAN_POINT ( 'NONE',  ( -4.622313124798576922, 5.235186282101428112, -11.61527771782819762 ) ) ;
#16341=CARTESIAN_POINT ( 'NONE',  ( 9.465287035748067623, 81.99768628210142651, 2.064181346179272847 ) ) ;
#16343=CARTESIAN_POINT ( 'NONE',  ( -3.474262827703527901, 133.5648137178985735, 8.843639120294245259 ) ) ;
#16349=CARTESIAN_POINT ( 'NONE',  ( 6.594114490232462877, 55.93981371789855217, -6.840914352311949109 ) ) ;
#16353=CARTESIAN_POINT ( 'NONE',  ( -12.46528703574811558, 70.60231371789855359, 2.660918448318004170 ) ) ;
#16358=CARTESIAN_POINT ( 'NONE',  ( 10.49813415416005213, 37.82731371789854791, -7.228626920338837358 ) ) ;
#16361=CARTESIAN_POINT ( 'NONE',  ( 10.49813415415989581, 8.972686282101431487, 7.228626920339068285 ) ) ;
#16370=CARTESIAN_POINT ( 'NONE',  ( 8.715434833792128799, 65.13981371789854791, -8.962234695871567070 ) ) ;
#16375=CARTESIAN_POINT ( 'NONE',  ( -8.632099005475794229, 32.65231371789855075, 13.23911966647199812 ) ) ;
#16377=CARTESIAN_POINT ( 'NONE',  ( 10.49813415415989581, 27.37268628210144783, 7.228626920339068285 ) ) ;
#16379=CARTESIAN_POINT ( 'NONE',  ( 2.660918448318279950, 61.29768628210143788, -12.46528703574805697 ) ) ;
#16380=CARTESIAN_POINT ( 'NONE',  ( 10.83675517735155225, 18.46018628210144286, 11.08355503943142573 ) ) ;
#16386=CARTESIAN_POINT ( 'NONE',  ( -6.092822981423970496, 29.38518628210144712, 14.25334919248782661 ) ) ;
#16392=CARTESIAN_POINT ( 'NONE',  ( 4.622313124798573369, 9.835186282101449962, 11.61527771782819940 ) ) ;
#16394=CARTESIAN_POINT ( 'NONE',  ( 2.064181346179061460, 105.1023137178985678, 9.465287035748106703 ) ) ;
#16399=CARTESIAN_POINT ( 'NONE',  ( -12.46528703574811558, 125.8023137178985706, 2.660918448318004170 ) ) ;
#16405=CARTESIAN_POINT ( 'NONE',  ( 10.49813415415989581, 27.37268628210144783, 7.228626920339069173 ) ) ;
#16412=CARTESIAN_POINT ( 'NONE',  ( -4.944772684328673229, 84.58518628210146062, 11.48171059495397728 ) ) ;
#16413=CARTESIAN_POINT ( 'NONE',  ( 14.25334919248782661, 137.4851862821014379, 6.092822981423971385 ) ) ;
#16420=CARTESIAN_POINT ( 'NONE',  ( 8.715434833792128799, 120.3398137178985650, -8.962234695871567070 ) ) ;
#16426=CARTESIAN_POINT ( 'NONE',  ( -3.257655550456946880, 91.30231371789854222, -15.46528703574811736 ) ) ;
#16430=CARTESIAN_POINT ( 'NONE',  ( 12.46528703574805874, 118.7976862821014663, 2.660918448318279950 ) ) ;
#16431=CARTESIAN_POINT ( 'NONE',  ( 13.23911966647218996, 71.64768628210146062, -8.632099005475504683 ) ) ;
#16434=CARTESIAN_POINT ( 'NONE',  ( -11.08355503943142573, 85.16018628210146346, 10.83675517735155402 ) ) ;
#16438=CARTESIAN_POINT ( 'NONE',  ( -8.843639120294326972, 39.73518628210145209, 3.474262827703335166 ) ) ;
#16443=CARTESIAN_POINT ( 'NONE',  ( -2.660918448318275509, 65.89768628210146062, 12.46528703574805874 ) ) ;
#16446=CARTESIAN_POINT ( 'NONE',  ( -9.465287035748065847, 31.39768628210144286, -2.064181346179273735 ) ) ;
#16457=CARTESIAN_POINT ( 'NONE',  ( 12.46528703574811558, 84.40231371789853654, -2.660918448318005503 ) ) ;
#16458=CARTESIAN_POINT ( 'NONE',  ( 4.622313124798573369, 83.43518628210145494, 11.61527771782819940 ) ) ;
#16463=CARTESIAN_POINT ( 'NONE',  ( 3.257655550456945548, 59.10231371789854649, 15.46528703574811736 ) ) ;
#16468=CARTESIAN_POINT ( 'NONE',  ( -9.500000000000005329, 34.08981371789853654, 0.1745138560723101806 ) ) ;
#16470=CARTESIAN_POINT ( 'NONE',  ( -8.710071997420207879, 97.91481371789856780, 3.796722387233182339 ) ) ;
#16472=CARTESIAN_POINT ( 'NONE',  ( -8.715434833792127023, 14.53981371789855892, 8.962234695871568846 ) ) ;
#16474=CARTESIAN_POINT ( 'NONE',  ( -2.311890736173176641, 60.72268628210144925, -12.53471296425194836 ) ) ;
#16482=CARTESIAN_POINT ( 'NONE',  ( -6.594114490232312775, 96.66018628210144925, -6.840914352312096547 ) ) ;
#16484=CARTESIAN_POINT ( 'NONE',  ( -12.53471296425194836, 113.6226862821014407, 2.311890736173176641 ) ) ;
#16496=CARTESIAN_POINT ( 'NONE',  ( 9.465287035748106703, 10.80231371789855466, -2.064181346179063237 ) ) ;
#16497=CARTESIAN_POINT ( 'NONE',  ( 10.49813415415989581, 137.7726862821014606, 7.228626920339069173 ) ) ;
#16501=CARTESIAN_POINT ( 'NONE',  ( -12.50000000000000355, 6.489813717898557321, 0.1745138560722785670 ) ) ;
#16503=CARTESIAN_POINT ( 'NONE',  ( -5.770363421894122880, 115.1648137178985678, 14.38691631536194393 ) ) ;
#16510=CARTESIAN_POINT ( 'NONE',  ( 12.53471296425194836, 109.0226862821014606, -2.311890736173178418 ) ) ;
#16516=CARTESIAN_POINT ( 'NONE',  ( 12.50000000000000355, 127.7101862821014606, 0.1745138560725507937 ) ) ;
#16521=CARTESIAN_POINT ( 'NONE',  ( 0.1745138560725837118, 125.4101862821014635, -15.50000000000000533 ) ) ;
#16523=CARTESIAN_POINT ( 'NONE',  ( -12.46528703574805697, 12.99768628210143362, -2.660918448318280838 ) ) ;
#16528=CARTESIAN_POINT ( 'NONE',  ( -1.715153634034234598, 88.32268628210142936, -9.534712964251941258 ) ) ;
#16530=CARTESIAN_POINT ( 'NONE',  ( -8.152565276336593669, 126.9523137178985621, -5.233372021372610483 ) ) ;
#16537=CARTESIAN_POINT ( 'NONE',  ( -8.152565276336593669, 53.35231371789856780, -5.233372021372610483 ) ) ;
#16542=CARTESIAN_POINT ( 'NONE',  ( -10.49813415416004858, 70.02731371789855075, 7.228626920338840023 ) ) ;
#16546=CARTESIAN_POINT ( 'NONE',  ( -7.228626920338836470, 35.52731371789855075, -10.49813415416005213 ) ) ;
#16556=CARTESIAN_POINT ( 'NONE',  ( 4.944772684328420986, 58.81481371789855217, 11.48171059495408208 ) ) ;
#16562=CARTESIAN_POINT ( 'NONE',  ( 14.38691631536194393, 48.46481371789856496, 5.770363421894124656 ) ) ;
#16565=CARTESIAN_POINT ( 'NONE',  ( 10.69584247140445221, 25.64768628210143930, -6.932735513423970097 ) ) ;
#16566=CARTESIAN_POINT ( 'NONE',  ( -11.48171059495397373, 68.48518628210145209, -4.944772684328680334 ) ) ;
#16567=CARTESIAN_POINT ( 'NONE',  ( -8.632099005475501130, 4.947686282101431132, -13.23911966647218996 ) ) ;
#16571=CARTESIAN_POINT ( 'NONE',  ( -8.632099005475501130, 32.54768628210143788, -13.23911966647218996 ) ) ;
#16577=CARTESIAN_POINT ( 'NONE',  ( 0.1745138560725515708, 5.810186282101447830, -12.50000000000000355 ) ) ;
#16580=CARTESIAN_POINT ( 'NONE',  ( 7.954856959092311719, 111.4273137178985422, -5.529263428287300108 ) ) ;
#16586=CARTESIAN_POINT ( 'NONE',  ( -4.944772684328424539, 118.6148137178985564, -11.48171059495408031 ) ) ;
#16601=CARTESIAN_POINT ( 'NONE',  ( -0.1745138560725500443, 56.41018628210145636, 12.50000000000000355 ) ) ;
#16607=CARTESIAN_POINT ( 'NONE',  ( 12.50000000000000355, 121.4898137178985564, -0.1745138560722771515 ) ) ;
#16613=CARTESIAN_POINT ( 'NONE',  ( -8.632099005475794229, 87.85231371789855359, 13.23911966647199812 ) ) ;
#16617=CARTESIAN_POINT ( 'NONE',  ( 12.50000000000000355, 118.5101862821014578, 0.1745138560725507937 ) ) ;
#16618=CARTESIAN_POINT ( 'NONE',  ( 5.770363421893814682, 65.03518628210144925, 14.38691631536207183 ) ) ;
#16622=CARTESIAN_POINT ( 'NONE',  ( -10.83675517735155047, 87.46018628210146062, -11.08355503943142750 ) ) ;
#16627=CARTESIAN_POINT ( 'NONE',  ( -8.843639120294326972, 30.53518628210144570, 3.474262827703335166 ) ) ;
#16631=CARTESIAN_POINT ( 'NONE',  ( 8.962234695871762469, 62.16018628210144215, -8.715434833791931624 ) ) ;
#16634=CARTESIAN_POINT ( 'NONE',  ( -3.796722387233375073, 29.38518628210144712, 8.710071997420127943 ) ) ;
#16645=CARTESIAN_POINT ( 'NONE',  ( 11.61527771782819940, 81.13518628210145778, -4.622313124798573369 ) ) ;
#16650=CARTESIAN_POINT ( 'NONE',  ( 8.927990412390371944, 49.32731371789854791, 13.04141134922778811 ) ) ;
#16655=CARTESIAN_POINT ( 'NONE',  ( -7.954856959092309943, 33.22731371789855359, 5.529263428287300108 ) ) ;
#16657=CARTESIAN_POINT ( 'NONE',  ( 1.715153634034445762, 101.0773137178985479, -9.534712964251895073 ) ) ;
#16659=CARTESIAN_POINT ( 'NONE',  ( 11.48171059495408208, 10.51481371789855856, -4.944772684328420986 ) ) ;
#16661=CARTESIAN_POINT ( 'NONE',  ( 12.50000000000000355, 72.51018628210145778, 0.1745138560725507937 ) ) ;
#16669=CARTESIAN_POINT ( 'NONE',  ( -3.474262827703337830, 69.63518628210144357, -8.843639120294326972 ) ) ;
#16672=CARTESIAN_POINT ( 'NONE',  ( 11.61527771782819940, 117.9351862821014549, -4.622313124798573369 ) ) ;
#16685=CARTESIAN_POINT ( 'NONE',  ( 7.228626920338837358, 132.1273137178986019, 10.49813415416005036 ) ) ;
#16686=CARTESIAN_POINT ( 'NONE',  ( 4.944772684328679446, 135.1851862821014549, -11.48171059495397373 ) ) ;
#16690=CARTESIAN_POINT ( 'NONE',  ( -4.944772684328424539, 8.214813717898532985, -11.48171059495408031 ) ) ;
#16692=CARTESIAN_POINT ( 'NONE',  ( 15.53471296425188797, 112.5773137178985479, 2.908627838312457747 ) ) ;
#16697=CARTESIAN_POINT ( 'NONE',  ( -8.962234695871760692, 112.7601862821014720, 8.715434833791933400 ) ) ;
#16704=CARTESIAN_POINT ( 'NONE',  ( 8.962234695871762469, 126.5601862821014691, -8.715434833791931624 ) ) ;
#16710=CARTESIAN_POINT ( 'NONE',  ( -14.25334919248782306, 123.6851862821014549, -6.092822981423979378 ) ) ;
#16712=CARTESIAN_POINT ( 'NONE',  ( -8.710071997420127943, 132.8851862821014436, -3.796722387233380402 ) ) ;
#16717=CARTESIAN_POINT ( 'NONE',  ( -0.1745138560725182642, 74.81018628210145494, 9.500000000000005329 ) ) ;
#16724=CARTESIAN_POINT ( 'NONE',  ( 5.233372021372610483, 64.85231371789855359, -8.152565276336593669 ) ) ;
#16728=CARTESIAN_POINT ( 'NONE',  ( -7.228626920338836470, 53.92731371789854933, -10.49813415416005213 ) ) ;
#16731=CARTESIAN_POINT ( 'NONE',  ( -10.69584247140429412, 25.75231371789854506, -6.932735513424201024 ) ) ;
#16734=CARTESIAN_POINT ( 'NONE',  ( -4.944772684328673229, 10.98518628210143433, 11.48171059495397728 ) ) ;
#16745=CARTESIAN_POINT ( 'NONE',  ( 3.257655550456945548, 40.70231371789854791, 15.46528703574811736 ) ) ;
#16747=CARTESIAN_POINT ( 'NONE',  ( -9.534712964251941258, 141.2226862821014493, 1.715153634034234154 ) ) ;
#16748=CARTESIAN_POINT ( 'NONE',  ( 11.61527771782819940, 62.73518628210145209, -4.622313124798573369 ) ) ;
#16749=CARTESIAN_POINT ( 'NONE',  ( -5.770363421893818234, 14.43518628210144072, -14.38691631536207005 ) ) ;
#16753=CARTESIAN_POINT ( 'NONE',  ( -14.38691631536207183, 30.53518628210144570, 5.770363421893814682 ) ) ;
#16761=CARTESIAN_POINT ( 'NONE',  ( 3.474262827703532341, 119.7648137178985905, -8.843639120294245259 ) ) ;
#16768=CARTESIAN_POINT ( 'NONE',  ( 0.1745138560722779009, 123.7898137178985678, 12.50000000000000355 ) ) ;
#16782=CARTESIAN_POINT ( 'NONE',  ( -6.932735513423968321, 60.14768628210144641, -10.69584247140445221 ) ) ;
#16789=CARTESIAN_POINT ( 'NONE',  ( 2.660918448318002838, 123.5023137178985735, 12.46528703574811558 ) ) ;
#16795=CARTESIAN_POINT ( 'NONE',  ( -15.53471296425188442, 89.57731371789856212, -2.908627838312459080 ) ) ;
#16801=CARTESIAN_POINT ( 'NONE',  ( 10.49813415415989581, 128.5726862821014720, 7.228626920339068285 ) ) ;
#16802=CARTESIAN_POINT ( 'NONE',  ( -8.927990412390661490, 57.27268628210143220, 13.04141134922759804 ) ) ;
#16806=CARTESIAN_POINT ( 'NONE',  ( 11.08355503943142750, 80.56018628210146915, -10.83675517735155225 ) ) ;
#16809=CARTESIAN_POINT ( 'NONE',  ( -5.529263428287477744, 29.67268628210143788, 7.954856959092191815 ) ) ;
#16813=CARTESIAN_POINT ( 'NONE',  ( -6.932735513423968321, 60.14768628210144641, -10.69584247140445221 ) ) ;
#16816=CARTESIAN_POINT ( 'NONE',  ( -5.233372021372430183, 32.54768628210143788, -8.152565276336710909 ) ) ;
#16827=CARTESIAN_POINT ( 'NONE',  ( -4.944772684328673229, 93.78518628210144925, 11.48171059495397728 ) ) ;
#16833=CARTESIAN_POINT ( 'NONE',  ( 14.38691631536194393, 39.26481371789855501, 5.770363421894124656 ) ) ;
#16841=CARTESIAN_POINT ( 'NONE',  ( -6.840914352311947333, 35.23981371789855643, -6.594114490232462877 ) ) ;
#16844=CARTESIAN_POINT ( 'NONE',  ( -1.715153634034442431, 87.27731371789855075, 9.534712964251900402 ) ) ;
#16846=CARTESIAN_POINT ( 'NONE',  ( 11.61527771782809637, 20.86481371789854222, 4.622313124798827388 ) ) ;
#16848=CARTESIAN_POINT ( 'NONE',  ( 11.48171059495397728, 73.08518628210144641, 4.944772684328674117 ) ) ;
#16850=PLANE ( 'NONE',  #3551 ) ;
#16856=CARTESIAN_POINT ( 'NONE',  ( 2.064181346179272847, 79.69768628210141515, -9.465287035748065847 ) ) ;
#16858=CARTESIAN_POINT ( 'NONE',  ( -0.1745138560725500443, 111.6101862821014521, 12.50000000000000355 ) ) ;
#16870=CARTESIAN_POINT ( 'NONE',  ( -12.53471296425189152, 117.1773137178985564, -2.311890736173453753 ) ) ;
#16878=CARTESIAN_POINT ( 'NONE',  ( -15.50000000000000533, 107.6898137178985735, 0.1745138560722471477 ) ) ;
#16883=CARTESIAN_POINT ( 'NONE',  ( -12.50000000000000355, 104.7101862821014606, -0.1745138560725492671 ) ) ;
#16889=CARTESIAN_POINT ( 'NONE',  ( 4.944772684328679446, 116.7851862821014635, -11.48171059495397373 ) ) ;
#16893=CARTESIAN_POINT ( 'NONE',  ( 14.25334919248782661, 109.8851862821014720, 6.092822981423971385 ) ) ;
#16894=CARTESIAN_POINT ( 'NONE',  ( -0.1745138560725500443, 19.61018628210144144, 12.50000000000000355 ) ) ;
#16896=CARTESIAN_POINT ( 'NONE',  ( -6.594114490232312775, 124.2601862821014578, -6.840914352312096547 ) ) ;
#16901=CARTESIAN_POINT ( 'NONE',  ( -5.529263428287477744, 57.27268628210143220, 7.954856959092191815 ) ) ;
#16909=CARTESIAN_POINT ( 'NONE',  ( 7.954856959092311719, 65.42731371789857064, -5.529263428287300108 ) ) ;
#16914=CARTESIAN_POINT ( 'NONE',  ( -6.932735513424201912, 69.45231371789856212, 10.69584247140429412 ) ) ;
#16917=CARTESIAN_POINT ( 'NONE',  ( 12.50000000000000355, 29.48981371789854933, -0.1745138560722771515 ) ) ;
#16921=CARTESIAN_POINT ( 'NONE',  ( 2.311890736173175753, 10.12268628210144428, 12.53471296425194836 ) ) ;
#16932=CARTESIAN_POINT ( 'NONE',  ( 8.632099005475788900, 28.05231371789855643, -13.23911966647199812 ) ) ;
#16934=CARTESIAN_POINT ( 'NONE',  ( -2.064181346179269738, 139.4976862821014549, 9.465287035748067623 ) ) ;
#16935=CARTESIAN_POINT ( 'NONE',  ( 10.49813415415989581, 54.97268628210144925, 7.228626920339068285 ) ) ;
#16939=CARTESIAN_POINT ( 'NONE',  ( 14.38691631536207538, 7.535186282101451916, -5.770363421893813793 ) ) ;
#16947=CARTESIAN_POINT ( 'NONE',  ( -0.1745138560723084320, 119.1898137178985593, -9.500000000000005329 ) ) ;
#16953=CARTESIAN_POINT ( 'NONE',  ( -7.228626920338836470, 118.3273137178985621, -10.49813415416005213 ) ) ;
#16966=CARTESIAN_POINT ( 'NONE',  ( -8.715434833791929847, 59.86018628210145209, -8.962234695871762469 ) ) ;
#16972=CARTESIAN_POINT ( 'NONE',  ( 12.53471296425189330, 112.5773137178985621, 2.311890736173451977 ) ) ;
#16977=CARTESIAN_POINT ( 'NONE',  ( 0.1745138560722461762, 86.98981371789857064, 15.50000000000000533 ) ) ;
#16981=CARTESIAN_POINT ( 'NONE',  ( 8.962234695871762469, 108.1601862821014635, -8.715434833791931624 ) ) ;
#16983=CARTESIAN_POINT ( 'NONE',  ( -6.092822981423970496, 66.18518628210145494, 14.25334919248782661 ) ) ;
#16988=CARTESIAN_POINT ( 'NONE',  ( 0.1745138560725837118, 61.01018628210145067, -15.50000000000000533 ) ) ;
#16990=CARTESIAN_POINT ( 'NONE',  ( 8.710071997420127943, 27.08518628210144996, 3.796722387233375073 ) ) ;
#16993=CARTESIAN_POINT ( 'NONE',  ( 0.1745138560725515708, 51.81018628210144783, -12.50000000000000355 ) ) ;
#16996=CARTESIAN_POINT ( 'NONE',  ( -5.529263428287477744, 29.67268628210143788, 7.954856959092191815 ) ) ;
#17008=CARTESIAN_POINT ( 'NONE',  ( -0.1745138560725500443, 74.81018628210145494, 12.50000000000000355 ) ) ;
#17013=CARTESIAN_POINT ( 'NONE',  ( -6.092822981423666739, 35.81481371789853796, -14.25334919248795096 ) ) ;
#17021=CARTESIAN_POINT ( 'NONE',  ( -1.715153634034442431, 32.07731371789855501, 9.534712964251900402 ) ) ;
#17026=CARTESIAN_POINT ( 'NONE',  ( 12.50000000000000355, 20.28981371789855004, -0.1745138560722771515 ) ) ;
#17029=CARTESIAN_POINT ( 'NONE',  ( 10.69584247140445221, 62.44768628210145778, -6.932735513423970097 ) ) ;
#17037=CARTESIAN_POINT ( 'NONE',  ( -7.954856959092191815, 77.97268628210142083, -5.529263428287477744 ) ) ;
#17039=CARTESIAN_POINT ( 'NONE',  ( -4.622313124798576922, 106.4351862821014549, -11.61527771782819762 ) ) ;
#17053=CARTESIAN_POINT ( 'NONE',  ( -8.715434833792127023, 115.7398137178985706, 8.962234695871568846 ) ) ;
#17054=CARTESIAN_POINT ( 'NONE',  ( -12.53471296425194659, 122.8226862821014720, 2.311890736173176641 ) ) ;
#17060=CARTESIAN_POINT ( 'NONE',  ( 13.23911966647199812, 94.75231371789854506, 8.632099005475788900 ) ) ;
#17061=CARTESIAN_POINT ( 'NONE',  ( 12.46528703574805874, 100.3976862821014464, 2.660918448318279950 ) ) ;
#17065=CARTESIAN_POINT ( 'NONE',  ( -10.49813415415989581, 114.7726862821014606, -7.228626920339068285 ) ) ;
#17069=CARTESIAN_POINT ( 'NONE',  ( -12.46528703574805697, 114.1976862821014720, -2.660918448318280838 ) ) ;
#17075=CARTESIAN_POINT ( 'NONE',  ( 3.257655550457285720, 98.09768628210146346, -15.46528703574804986 ) ) ;
#17076=CARTESIAN_POINT ( 'NONE',  ( -8.962234695871760692, 20.76018628210144001, 8.715434833791933400 ) ) ;
#17080=CARTESIAN_POINT ( 'NONE',  ( 5.529263428287477744, 126.2726862821014464, -7.954856959092191815 ) ) ;
#17085=CARTESIAN_POINT ( 'NONE',  ( 9.465287035748067623, 54.39768628210144641, 2.064181346179272847 ) ) ;
#17094=CARTESIAN_POINT ( 'NONE',  ( 8.710071997420211432, 47.31481371789856638, -3.796722387233181895 ) ) ;
#17099=CARTESIAN_POINT ( 'NONE',  ( -4.622313124798826500, 59.96481371789855075, 11.61527771782809637 ) ) ;
#17102=CARTESIAN_POINT ( 'NONE',  ( -13.04141134922778456, 143.6273137178985451, 8.927990412390377273 ) ) ;
#17119=CARTESIAN_POINT ( 'NONE',  ( -13.04141134922778456, 24.02731371789854364, 8.927990412390377273 ) ) ;
#17121=CARTESIAN_POINT ( 'NONE',  ( 4.944772684328679446, 6.385186282101440014, -11.48171059495397373 ) ) ;
#17123=CARTESIAN_POINT ( 'NONE',  ( 12.46528703574805874, 54.39768628210146062, 2.660918448318279950 ) ) ;
#17127=CARTESIAN_POINT ( 'NONE',  ( -6.092822981423970496, 10.98518628210143433, 14.25334919248782661 ) ) ;
#17135=CARTESIAN_POINT ( 'NONE',  ( 1.715153634034445762, 101.0773137178985479, -9.534712964251895073 ) ) ;
#17142=CARTESIAN_POINT ( 'NONE',  ( 11.48171059495408208, 120.9148137178985536, -4.944772684328420986 ) ) ;
#17146=CARTESIAN_POINT ( 'NONE',  ( -12.50000000000000355, 80.08981371789855075, 0.1745138560722786503 ) ) ;
#17155=CARTESIAN_POINT ( 'NONE',  ( -2.660918448318275509, 65.89768628210146062, 12.46528703574805874 ) ) ;
#17162=CARTESIAN_POINT ( 'NONE',  ( 12.50000000000000355, 103.0898137178985650, -0.1745138560722771515 ) ) ;
#17167=CARTESIAN_POINT ( 'NONE',  ( 2.908627838312458636, 73.47731371789855359, -15.53471296425188442 ) ) ;
#17171=CARTESIAN_POINT ( 'NONE',  ( -11.61527771782819940, 104.1351862821014578, 4.622313124798574258 ) ) ;
#17172=CARTESIAN_POINT ( 'NONE',  ( 2.908627838312118019, 46.92268628210143788, 15.53471296425195369 ) ) ;
#17176=CARTESIAN_POINT ( 'NONE',  ( -15.50000000000000533, 58.71018628210145351, -0.1745138560725808530 ) ) ;
#17181=CARTESIAN_POINT ( 'NONE',  ( -0.1745138560725500443, 38.01018628210144357, 12.50000000000000355 ) ) ;
#17184=CARTESIAN_POINT ( 'NONE',  ( 2.064181346179272847, 15.29768628210142722, -9.465287035748065847 ) ) ;
#17195=CARTESIAN_POINT ( 'NONE',  ( 2.311890736173175753, 74.52268628210146062, 12.53471296425194659 ) ) ;
#17201=CARTESIAN_POINT ( 'NONE',  ( 15.53471296425188797, 48.17731371789854222, 2.908627838312457747 ) ) ;
#17207=CARTESIAN_POINT ( 'NONE',  ( 9.534712964251900402, 29.77731371789854364, 1.715153634034445540 ) ) ;
#17213=CARTESIAN_POINT ( 'NONE',  ( 15.50000000000000533, 130.6898137178985451, -0.1745138560722452326 ) ) ;
#17215=AXIS2_PLACEMENT_3D ( 'NONE', #16047, #4651, #19645 ) ;
#17217=CARTESIAN_POINT ( 'NONE',  ( -2.660918448318275509, 38.29768628210145920, 12.46528703574805874 ) ) ;
#17225=CARTESIAN_POINT ( 'NONE',  ( -5.529263428287477744, 75.67268628210143788, 7.954856959092191815 ) ) ;
#17227=CARTESIAN_POINT ( 'NONE',  ( -6.932735513423968321, 87.74768628210145494, -10.69584247140445221 ) ) ;
#17238=CARTESIAN_POINT ( 'NONE',  ( -8.962234695871565293, 127.2398137178985564, -8.715434833792128799 ) ) ;
#17239=CARTESIAN_POINT ( 'NONE',  ( 12.53471296425194659, 118.2226862821014635, -2.311890736173178418 ) ) ;
#17245=CARTESIAN_POINT ( 'NONE',  ( 8.927990412390371944, 95.32731371789854791, 13.04141134922778811 ) ) ;
#17249=CARTESIAN_POINT ( 'NONE',  ( -8.710071997420207879, 79.51481371789856212, 3.796722387233182339 ) ) ;
#17254=CARTESIAN_POINT ( 'NONE',  ( 2.311890736173452865, 73.47731371789856780, -12.53471296425189152 ) ) ;
#17256=CARTESIAN_POINT ( 'NONE',  ( -4.944772684328673229, 112.1851862821014549, 11.48171059495397728 ) ) ;
#17261=CARTESIAN_POINT ( 'NONE',  ( 14.38691631536207538, 99.53518628210146346, -5.770363421893813793 ) ) ;
#17263=CARTESIAN_POINT ( 'NONE',  ( -10.49813415415989404, 13.57268628210145422, -7.228626920339069173 ) ) ;
#17266=CARTESIAN_POINT ( 'NONE',  ( -6.840914352312096547, 140.3601862821014663, 6.594114490232313663 ) ) ;
#17272=CARTESIAN_POINT ( 'NONE',  ( -1.715153634034234598, 60.72268628210144925, -9.534712964251941258 ) ) ;
#17278=CARTESIAN_POINT ( 'NONE',  ( -3.474262827703527901, 41.56481371789855217, 8.843639120294245259 ) ) ;
#17283=CARTESIAN_POINT ( 'NONE',  ( 0.1745138560722779009, 40.98981371789854933, 12.50000000000000355 ) ) ;
#17286=CARTESIAN_POINT ( 'NONE',  ( -10.69584247140429412, 16.55231371789855999, -6.932735513424201024 ) ) ;
#17303=CARTESIAN_POINT ( 'NONE',  ( -8.632099005475794229, 23.45231371789854435, 13.23911966647199812 ) ) ;
#17306=CARTESIAN_POINT ( 'NONE',  ( -2.311890736173176641, 14.72268628210143859, -12.53471296425194836 ) ) ;
#17307=CARTESIAN_POINT ( 'NONE',  ( 2.660918448318279950, 52.09768628210144215, -12.46528703574805697 ) ) ;
#17318=CARTESIAN_POINT ( 'NONE',  ( 6.840914352311949109, 95.03981371789855359, 6.594114490232462877 ) ) ;
#17325=CARTESIAN_POINT ( 'NONE',  ( 2.660918448318003282, 105.1023137178985678, 12.46528703574811558 ) ) ;
#17329=CARTESIAN_POINT ( 'NONE',  ( -11.61527771782809282, 71.46481371789856496, -4.622313124798832717 ) ) ;
#17339=CARTESIAN_POINT ( 'NONE',  ( -7.228626920339069173, 48.07268628210143646, 10.49813415415989581 ) ) ;
#17346=CARTESIAN_POINT ( 'NONE',  ( -10.49813415416004858, 106.8273137178985479, 7.228626920338839135 ) ) ;
#17352=CARTESIAN_POINT ( 'NONE',  ( -8.632099005475794229, 78.65231371789856496, 13.23911966647199812 ) ) ;
#17356=CARTESIAN_POINT ( 'NONE',  ( 7.228626920339068285, 107.8726862821014549, -10.49813415415989581 ) ) ;
#17357=CARTESIAN_POINT ( 'NONE',  ( -3.257655550457281723, 38.29768628210144499, 15.46528703574804986 ) ) ;
#17360=CARTESIAN_POINT ( 'NONE',  ( -5.770363421893818234, 69.63518628210144357, -14.38691631536207005 ) ) ;
#17367=CARTESIAN_POINT ( 'NONE',  ( 8.962234695871762469, 43.76018628210144357, -8.715434833791931624 ) ) ;
#17370=CARTESIAN_POINT ( 'NONE',  ( -9.465287035748065847, 12.99768628210143362, -2.064181346179273735 ) ) ;
#17382=CARTESIAN_POINT ( 'NONE',  ( -2.311890736173176641, 69.92268628210145209, -12.53471296425194659 ) ) ;
#17389=CARTESIAN_POINT ( 'NONE',  ( 15.53471296425188797, 38.97731371789853938, 2.908627838312457747 ) ) ;
#17397=CARTESIAN_POINT ( 'NONE',  ( -2.064181346179062349, 17.70231371789854435, -9.465287035748106703 ) ) ;
#17402=CARTESIAN_POINT ( 'NONE',  ( 11.08355503943118769, 122.6398137178985479, 10.83675517735179028 ) ) ;
#17404=CARTESIAN_POINT ( 'NONE',  ( 11.48171059495397728, 45.48518628210145209, 4.944772684328674117 ) ) ;
#17411=CARTESIAN_POINT ( 'NONE',  ( 9.465287035748067623, 81.99768628210142651, 2.064181346179272847 ) ) ;
#17414=CARTESIAN_POINT ( 'NONE',  ( 4.944772684328679446, 89.18518628210145494, -11.48171059495397373 ) ) ;
#17426=CARTESIAN_POINT ( 'NONE',  ( -2.311890736173448424, 114.8773137178985735, 12.53471296425189330 ) ) ;
#17427=CARTESIAN_POINT ( 'NONE',  ( 2.660918448318279950, 125.6976862821014578, -12.46528703574805874 ) ) ;
#17432=CARTESIAN_POINT ( 'NONE',  ( 8.632099005475788900, 92.45231371789854791, -13.23911966647199812 ) ) ;
#17437=CARTESIAN_POINT ( 'NONE',  ( -1.715153634034442431, 68.87731371789855928, 9.534712964251900402 ) ) ;
#17440=CARTESIAN_POINT ( 'NONE',  ( -6.932735513424201912, 51.05231371789854933, 10.69584247140429412 ) ) ;
#17442=CARTESIAN_POINT ( 'NONE',  ( -7.228626920339069173, 94.07268628210145778, 10.49813415415989581 ) ) ;
#17448=CARTESIAN_POINT ( 'NONE',  ( 13.04141134922759804, 110.1726862821014663, 8.927990412390657937 ) ) ;
#17449=CARTESIAN_POINT ( 'NONE',  ( 11.61527771782819940, 7.535186282101452804, -4.622313124798573369 ) ) ;
#17452=CARTESIAN_POINT ( 'NONE',  ( -9.465287035748065847, 132.5976862821014493, -2.064181346179273735 ) ) ;
#17458=CARTESIAN_POINT ( 'NONE',  ( -9.465287035748065847, 58.99768628210144783, -2.064181346179273735 ) ) ;
#17465=CARTESIAN_POINT ( 'NONE',  ( 5.233372021372610483, 46.45231371789854791, -8.152565276336593669 ) ) ;
#17471=CARTESIAN_POINT ( 'NONE',  ( 6.932735513424201024, 46.45231371789855501, -10.69584247140429412 ) ) ;
#17474=CARTESIAN_POINT ( 'NONE',  ( 12.46528703574811558, 10.80231371789855466, -2.660918448318005503 ) ) ;
#17490=CARTESIAN_POINT ( 'NONE',  ( 13.23911966647199812, 21.15231371789855430, 8.632099005475788900 ) ) ;
#17492=CARTESIAN_POINT ( 'NONE',  ( -6.932735513423968321, 14.14768628210144463, -10.69584247140445221 ) ) ;
#17493=CARTESIAN_POINT ( 'NONE',  ( 6.932735513423970097, 46.34768628210145636, 10.69584247140445044 ) ) ;
#17505=CARTESIAN_POINT ( 'NONE',  ( -2.064181346179062349, 91.30231371789854222, -9.465287035748106703 ) ) ;
#17512=CARTESIAN_POINT ( 'NONE',  ( -10.69584247140429412, 99.35231371789855359, -6.932735513424201024 ) ) ;
#17517=CARTESIAN_POINT ( 'NONE',  ( -7.228626920338836470, 72.32731371789854791, -10.49813415416005213 ) ) ;
#17526=CARTESIAN_POINT ( 'NONE',  ( 8.962234695871762469, 34.56018628210144783, -8.715434833791931624 ) ) ;
#17532=CARTESIAN_POINT ( 'NONE',  ( 7.228626920338837358, 95.32731371789856212, 10.49813415416005036 ) ) ;
#17538=CARTESIAN_POINT ( 'NONE',  ( 6.092822981423662299, 77.21481371789855075, 14.25334919248795096 ) ) ;
#17542=CARTESIAN_POINT ( 'NONE',  ( -12.53471296425194836, 104.4226862821014379, 2.311890736173176641 ) ) ;
#17543=CARTESIAN_POINT ( 'NONE',  ( -15.50000000000000533, 40.31018628210145494, -0.1745138560725808530 ) ) ;
#17546=CARTESIAN_POINT ( 'NONE',  ( 13.23911966647218996, 71.64768628210146062, -8.632099005475504683 ) ) ;
#17553=CARTESIAN_POINT ( 'NONE',  ( 10.69584247140445221, 44.04768628210144499, -6.932735513423970097 ) ) ;
#17556=CARTESIAN_POINT ( 'NONE',  ( 8.152565276336714462, 16.44768628210144001, -5.233372021372432847 ) ) ;
#17567=CARTESIAN_POINT ( 'NONE',  ( 6.932735513423970097, 73.94768628210145778, 10.69584247140445044 ) ) ;
#17576=CARTESIAN_POINT ( 'NONE',  ( 3.257655550456945548, 31.50231371789854862, 15.46528703574811736 ) ) ;
#17582=CARTESIAN_POINT ( 'NONE',  ( 9.465287035748106703, 29.20231371789855501, -2.064181346179063237 ) ) ;
#17589=CARTESIAN_POINT ( 'NONE',  ( -14.38691631536193860, 135.8648137178985849, -5.770363421894132649 ) ) ;
#17593=CARTESIAN_POINT ( 'NONE',  ( 7.228626920339068285, 52.67268628210144499, -10.49813415415989581 ) ) ;
#17600=CARTESIAN_POINT ( 'NONE',  ( -5.233372021372430183, 60.14768628210144641, -8.152565276336710909 ) ) ;
#17605=CARTESIAN_POINT ( 'NONE',  ( 11.61527771782819940, 99.53518628210144925, -4.622313124798573369 ) ) ;
#17617=CARTESIAN_POINT ( 'NONE',  ( -8.962234695871565293, 118.0398137178985678, -8.715434833792128799 ) ) ;
#17618=CARTESIAN_POINT ( 'NONE',  ( 7.228626920339069173, 117.0726862821014578, -10.49813415415989404 ) ) ;
#17624=CARTESIAN_POINT ( 'NONE',  ( -5.770363421894122880, 87.56481371789857349, 14.38691631536194393 ) ) ;
#17628=CARTESIAN_POINT ( 'NONE',  ( -6.840914352311947333, 81.23981371789855643, -6.594114490232462877 ) ) ;
#17631=CARTESIAN_POINT ( 'NONE',  ( -12.53471296425189152, 43.57731371789855501, -2.311890736173453753 ) ) ;
#17633=CARTESIAN_POINT ( 'NONE',  ( 2.311890736173175753, 92.92268628210145209, 12.53471296425194836 ) ) ;
#17639=CARTESIAN_POINT ( 'NONE',  ( 2.908627838312118019, 92.92268628210145209, 15.53471296425195369 ) ) ;
#17640=CARTESIAN_POINT ( 'NONE',  ( -4.622313124798576922, 14.43518628210144250, -11.61527771782819762 ) ) ;
#17643=CARTESIAN_POINT ( 'NONE',  ( 5.529263428287477744, 117.0726862821014294, -7.954856959092191815 ) ) ;
#17649=CARTESIAN_POINT ( 'NONE',  ( 9.534712964251941258, 53.82268628210144357, -1.715153634034235708 ) ) ;
#17655=CARTESIAN_POINT ( 'NONE',  ( 3.474262827703532341, 36.96481371789853654, -8.843639120294245259 ) ) ;
#17660=CARTESIAN_POINT ( 'NONE',  ( -7.228626920338836470, 35.52731371789855075, -10.49813415416005213 ) ) ;
#17663=CARTESIAN_POINT ( 'NONE',  ( -12.46528703574811558, 15.40231371789854542, 2.660918448318003726 ) ) ;
#17678=CARTESIAN_POINT ( 'NONE',  ( 13.04141134922778988, 28.62731371789854506, -8.927990412390371944 ) ) ;
#17681=CARTESIAN_POINT ( 'NONE',  ( 9.465287035748067623, 137.1976862821014436, 2.064181346179272847 ) ) ;
#17682=CARTESIAN_POINT ( 'NONE',  ( -10.49813415415989581, 41.17268628210144499, -7.228626920339068285 ) ) ;
#17687=CARTESIAN_POINT ( 'NONE',  ( 6.840914352312096547, 16.16018628210144570, -6.594114490232313663 ) ) ;
#17694=CARTESIAN_POINT ( 'NONE',  ( -9.500000000000005329, 98.48981371789855643, 0.1745138560723101806 ) ) ;
#17698=CARTESIAN_POINT ( 'NONE',  ( 12.50000000000000355, 93.88981371789856212, -0.1745138560722771515 ) ) ;
#17702=CARTESIAN_POINT ( 'NONE',  ( 12.46528703574811558, 75.20231371789856212, -2.660918448318005503 ) ) ;
#17709=CARTESIAN_POINT ( 'NONE',  ( -12.50000000000000355, 31.11018628210143788, -0.1745138560725492671 ) ) ;
#17716=CARTESIAN_POINT ( 'NONE',  ( -6.932735513424201912, 106.2523137178985735, 10.69584247140429412 ) ) ;
#17721=CARTESIAN_POINT ( 'NONE',  ( -3.257655550456946880, 72.90231371789855075, -15.46528703574811736 ) ) ;
#17725=CARTESIAN_POINT ( 'NONE',  ( 11.61527771782819940, 108.7351862821014663, -4.622313124798573369 ) ) ;
#17726=CARTESIAN_POINT ( 'NONE',  ( 15.46528703574804986, 54.39768628210144641, 3.257655550457285720 ) ) ;
#17727=PLANE ( 'NONE',  #2306 ) ;
#17729=CARTESIAN_POINT ( 'NONE',  ( -10.83675517735155047, 69.06018628210144072, -11.08355503943142750 ) ) ;
#17737=CARTESIAN_POINT ( 'NONE',  ( 12.46528703574805874, 35.99768628210144072, 2.660918448318279950 ) ) ;
#17740=CARTESIAN_POINT ( 'NONE',  ( 8.843639120294328748, 7.535186282101451916, -3.474262827703334722 ) ) ;
#17750=CARTESIAN_POINT ( 'NONE',  ( 4.622313124798573369, 74.23518628210145209, 11.61527771782819940 ) ) ;
#17758=CARTESIAN_POINT ( 'NONE',  ( 10.69584247140445221, 90.04768628210145209, -6.932735513423970097 ) ) ;
#17759=CARTESIAN_POINT ( 'NONE',  ( 8.632099005475788900, 28.05231371789855643, -13.23911966647199812 ) ) ;
#17765=CARTESIAN_POINT ( 'NONE',  ( -0.1745138560723084320, 17.98981371789853867, -9.500000000000005329 ) ) ;
#17771=CARTESIAN_POINT ( 'NONE',  ( -8.927990412390371944, 136.7273137178985110, -13.04141134922778988 ) ) ;
#17774=CARTESIAN_POINT ( 'NONE',  ( -4.944772684328673229, 47.78518628210144925, 11.48171059495397728 ) ) ;
#17782=CARTESIAN_POINT ( 'NONE',  ( 6.594114490232313663, 55.26018628210144357, 6.840914352312096547 ) ) ;
#17786=CARTESIAN_POINT ( 'NONE',  ( 8.962234695871762469, 98.96018628210146062, -8.715434833791931624 ) ) ;
#17798=CARTESIAN_POINT ( 'NONE',  ( 12.46528703574811558, 112.0023137178985735, -2.660918448318005503 ) ) ;
#17800=CARTESIAN_POINT ( 'NONE',  ( 12.46528703574805874, 118.7976862821014663, 2.660918448318279950 ) ) ;
#17805=CARTESIAN_POINT ( 'NONE',  ( 14.38691631536194393, 94.46481371789855075, 5.770363421894124656 ) ) ;
#17809=CARTESIAN_POINT ( 'NONE',  ( -8.710071997420127943, 105.2851862821014777, -3.796722387233380402 ) ) ;
#17814=CARTESIAN_POINT ( 'NONE',  ( 1.715153634034445762, 73.47731371789855359, -9.534712964251895073 ) ) ;
#17820=CARTESIAN_POINT ( 'NONE',  ( -12.50000000000000355, 43.28981371789855359, 0.1745138560722786503 ) ) ;
#17822=CARTESIAN_POINT ( 'NONE',  ( 12.53471296425194836, 109.0226862821014606, -2.311890736173178418 ) ) ;
#17827=CARTESIAN_POINT ( 'NONE',  ( 10.69584247140445221, 136.0476862821014379, -6.932735513423970097 ) ) ;
#17829=CARTESIAN_POINT ( 'NONE',  ( 13.23911966647218996, 80.84768628210143504, -8.632099005475504683 ) ) ;
#17833=CARTESIAN_POINT ( 'NONE',  ( 3.796722387233379514, 107.5851862821014748, -8.710071997420127943 ) ) ;
#17835=CARTESIAN_POINT ( 'NONE',  ( 15.53471296425195369, 17.02268628210144996, -2.908627838312120684 ) ) ;
#17846=CARTESIAN_POINT ( 'NONE',  ( 8.843639120294245259, 11.66481371789854293, 3.474262827703527901 ) ) ;
#17850=CARTESIAN_POINT ( 'NONE',  ( -6.932735513424201912, 51.05231371789854933, 10.69584247140429412 ) ) ;
#17852=CARTESIAN_POINT ( 'NONE',  ( 12.46528703574811558, 20.00231371789855217, -2.660918448318005503 ) ) ;
#17867=CARTESIAN_POINT ( 'NONE',  ( 10.83675517735179206, 9.939813717898537959, -11.08355503943118769 ) ) ;
#17869=CARTESIAN_POINT ( 'NONE',  ( -9.500000000000005329, 132.3101862821014549, -0.1745138560725176813 ) ) ;
#17870=CARTESIAN_POINT ( 'NONE',  ( -0.1745138560725500443, 28.81018628210144072, 12.50000000000000355 ) ) ;
#17874=CARTESIAN_POINT ( 'NONE',  ( 0.1745138560725837118, 125.4101862821014635, -15.50000000000000533 ) ) ;
#17876=CARTESIAN_POINT ( 'NONE',  ( 7.954856959092191815, 8.972686282101431487, 5.529263428287477744 ) ) ;
#17883=CARTESIAN_POINT ( 'NONE',  ( 9.534712964251900402, 84.97731371789856780, 1.715153634034445540 ) ) ;
#17888=CARTESIAN_POINT ( 'NONE',  ( -12.50000000000000355, 107.6898137178985735, 0.1745138560722786503 ) ) ;
#17892=CARTESIAN_POINT ( 'NONE',  ( -10.49813415416004858, 60.82731371789855501, 7.228626920338839135 ) ) ;
#17900=CARTESIAN_POINT ( 'NONE',  ( 10.49813415415989581, 36.57268628210145067, 7.228626920339068285 ) ) ;
#17906=CARTESIAN_POINT ( 'NONE',  ( 8.962234695871567070, 85.83981371789856496, 8.715434833792127023 ) ) ;
#17910=CARTESIAN_POINT ( 'NONE',  ( -8.632099005475794229, 69.45231371789853370, 13.23911966647199812 ) ) ;
#17915=CARTESIAN_POINT ( 'NONE',  ( 10.69584247140445221, 90.04768628210145209, -6.932735513423970097 ) ) ;
#17916=CARTESIAN_POINT ( 'NONE',  ( 5.770363421893814682, 46.63518628210144357, 14.38691631536207183 ) ) ;
#17919=CARTESIAN_POINT ( 'NONE',  ( 13.04141134922759804, 54.97268628210144215, 8.927990412390657937 ) ) ;
#17926=CARTESIAN_POINT ( 'NONE',  ( -6.932735513423968321, 32.54768628210144499, -10.69584247140445221 ) ) ;
#17928=CARTESIAN_POINT ( 'NONE',  ( -7.954856959092309943, 143.6273137178985451, 5.529263428287300108 ) ) ;
#17938=CARTESIAN_POINT ( 'NONE',  ( 7.228626920339069173, 43.47268628210144925, -10.49813415415989404 ) ) ;
#17946=CARTESIAN_POINT ( 'NONE',  ( -8.962234695871760692, 103.5601862821014549, 8.715434833791933400 ) ) ;
#17947=CARTESIAN_POINT ( 'NONE',  ( -13.23911966647199812, 25.75231371789854506, -8.632099005475788900 ) ) ;
#17955=CARTESIAN_POINT ( 'NONE',  ( 6.594114490232462877, 19.13981371789855146, -6.840914352311949109 ) ) ;
#17962=CARTESIAN_POINT ( 'NONE',  ( -8.632099005475794229, 133.8523137178985394, 13.23911966647199812 ) ) ;
#17965=CARTESIAN_POINT ( 'NONE',  ( -10.49813415415989581, 41.17268628210144499, -7.228626920339068285 ) ) ;
#17972=CARTESIAN_POINT ( 'NONE',  ( 0.1745138560725194299, 51.81018628210144783, -9.500000000000005329 ) ) ;
#17975=CARTESIAN_POINT ( 'NONE',  ( -4.622313124798576922, 88.03518628210144925, -11.61527771782819762 ) ) ;
#17989=CARTESIAN_POINT ( 'NONE',  ( -11.48171059495408208, 107.1148137178985564, 4.944772684328421875 ) ) ;
#17990=CARTESIAN_POINT ( 'NONE',  ( -10.49813415415989404, 96.37268628210145494, -7.228626920339069173 ) ) ;
#17996=CARTESIAN_POINT ( 'NONE',  ( -15.50000000000000533, 70.88981371789854791, 0.1745138560722471477 ) ) ;
#17999=CARTESIAN_POINT ( 'NONE',  ( -3.796722387233375073, 102.9851862821014805, 8.710071997420127943 ) ) ;
#18002=CARTESIAN_POINT ( 'NONE',  ( 5.233372021372610483, 74.05231371789854222, -8.152565276336593669 ) ) ;
#18005=CARTESIAN_POINT ( 'NONE',  ( -12.50000000000000355, 52.48981371789855643, 0.1745138560722786503 ) ) ;
#18007=CARTESIAN_POINT ( 'NONE',  ( -4.622313124798576922, 106.4351862821014549, -11.61527771782819762 ) ) ;
#18010=CARTESIAN_POINT ( 'NONE',  ( 11.48171059495397728, 137.4851862821014663, 4.944772684328674117 ) ) ;
#18012=CARTESIAN_POINT ( 'NONE',  ( 5.770363421893814682, 74.23518628210142367, 14.38691631536207183 ) ) ;
#18017=CARTESIAN_POINT ( 'NONE',  ( -8.152565276336710909, 113.0476862821014663, 5.233372021372435512 ) ) ;
#18019=CARTESIAN_POINT ( 'NONE',  ( 10.83675517735155225, 18.46018628210144286, 11.08355503943142573 ) ) ;
#18032=CARTESIAN_POINT ( 'NONE',  ( 8.710071997420211432, 28.91481371789854649, -3.796722387233181895 ) ) ;
#18036=CARTESIAN_POINT ( 'NONE',  ( 2.660918448318003282, 40.70231371789854791, 12.46528703574811558 ) ) ;
#18038=CARTESIAN_POINT ( 'NONE',  ( -15.53471296425188442, 135.5773137178985905, -2.908627838312459080 ) ) ;
#18056=CARTESIAN_POINT ( 'NONE',  ( -13.23911966647199812, 7.352313717898546486, -8.632099005475788900 ) ) ;
#18058=CARTESIAN_POINT ( 'NONE',  ( 7.954856959092191815, 128.5726862821014436, 5.529263428287477744 ) ) ;
#18061=CARTESIAN_POINT ( 'NONE',  ( -8.715434833791929847, 23.06018628210145138, -8.962234695871762469 ) ) ;
#18067=CARTESIAN_POINT ( 'NONE',  ( 14.38691631536207538, 127.1351862821014720, -5.770363421893813793 ) ) ;
#18069=CARTESIAN_POINT ( 'NONE',  ( -9.500000000000005329, 144.4898137178985280, 0.1745138560723101806 ) ) ;
#18075=CARTESIAN_POINT ( 'NONE',  ( -8.710071997420207879, 79.51481371789856212, 3.796722387233182339 ) ) ;
#18080=CARTESIAN_POINT ( 'NONE',  ( -4.622313124798826500, 105.9648137178985650, 11.61527771782809637 ) ) ;
#18084=CARTESIAN_POINT ( 'NONE',  ( -2.311890736173448424, 68.87731371789855928, 12.53471296425189330 ) ) ;
#18092=CARTESIAN_POINT ( 'NONE',  ( 2.311890736173175753, 37.72268628210144215, 12.53471296425194836 ) ) ;
#18098=CARTESIAN_POINT ( 'NONE',  ( -2.660918448318004614, 82.10231371789855359, -12.46528703574811558 ) ) ;
#18103=CARTESIAN_POINT ( 'NONE',  ( 13.23911966647199812, 57.95231371789854791, 8.632099005475788900 ) ) ;
#18106=CARTESIAN_POINT ( 'NONE',  ( -10.49813415415989581, 77.97268628210144925, -7.228626920339068285 ) ) ;
#18107=CARTESIAN_POINT ( 'NONE',  ( -11.08355503943142573, 29.96018628210143575, 10.83675517735155402 ) ) ;
#18110=CARTESIAN_POINT ( 'NONE',  ( 14.25334919248782661, 45.48518628210144499, 6.092822981423971385 ) ) ;
#18116=CARTESIAN_POINT ( 'NONE',  ( 2.660918448318279950, 15.29768628210143078, -12.46528703574805697 ) ) ;
#18118=CARTESIAN_POINT ( 'NONE',  ( 9.500000000000005329, 130.6898137178985451, -0.1745138560723090149 ) ) ;
#18129=CARTESIAN_POINT ( 'NONE',  ( -12.46528703574805874, 49.79768628210144499, -2.660918448318280838 ) ) ;
#18137=CARTESIAN_POINT ( 'NONE',  ( -10.69584247140444866, 103.8476862821014493, 6.932735513423972762 ) ) ;
#18138=CARTESIAN_POINT ( 'NONE',  ( -2.908627838312453306, 13.67731371789853867, 15.53471296425188797 ) ) ;
#18144=CARTESIAN_POINT ( 'NONE',  ( 2.660918448318002838, 132.7023137178985621, 12.46528703574811558 ) ) ;
#18151=CARTESIAN_POINT ( 'NONE',  ( -15.50000000000000533, 116.8898137178985621, 0.1745138560722471477 ) ) ;
#18154=CARTESIAN_POINT ( 'NONE',  ( 4.622313124798573369, 19.03518628210144925, 11.61527771782819940 ) ) ;
#18158=CARTESIAN_POINT ( 'NONE',  ( -14.25334919248782306, 105.2851862821014777, -6.092822981423979378 ) ) ;
#18161=CARTESIAN_POINT ( 'NONE',  ( 8.843639120294328748, 53.53518628210145636, -3.474262827703334722 ) ) ;
#18164=CARTESIAN_POINT ( 'NONE',  ( 12.50000000000000355, 81.71018628210144641, 0.1745138560725507937 ) ) ;
#18178=CARTESIAN_POINT ( 'NONE',  ( 12.50000000000000355, 103.0898137178985650, -0.1745138560722771515 ) ) ;
#18179=CARTESIAN_POINT ( 'NONE',  ( 2.660918448318279950, 98.09768628210146346, -12.46528703574805874 ) ) ;
#18183=CARTESIAN_POINT ( 'NONE',  ( -8.632099005475794229, 78.65231371789856496, 13.23911966647199812 ) ) ;
#18187=CARTESIAN_POINT ( 'NONE',  ( 9.465287035748067623, 91.19768628210145778, 2.064181346179272847 ) ) ;
#18189=CARTESIAN_POINT ( 'NONE',  ( -6.840914352311947333, 62.83981371789855785, -6.594114490232462877 ) ) ;
#18192=CARTESIAN_POINT ( 'NONE',  ( 6.840914352311949109, 104.2398137178985706, 6.594114490232462877 ) ) ;
#18194=CARTESIAN_POINT ( 'NONE',  ( -7.228626920338836470, 44.72731371789855359, -10.49813415416005213 ) ) ;
#18197=CARTESIAN_POINT ( 'NONE',  ( -4.622313124798576922, 97.23518628210145209, -11.61527771782819762 ) ) ;
#18200=CARTESIAN_POINT ( 'NONE',  ( -11.48171059495397373, 132.8851862821014720, -4.944772684328680334 ) ) ;
#18202=CARTESIAN_POINT ( 'NONE',  ( -15.46528703574804986, 86.59768628210143504, -3.257655550457287497 ) ) ;
#18206=CARTESIAN_POINT ( 'NONE',  ( -3.796722387233375073, 112.1851862821014691, 8.710071997420127943 ) ) ;
#18208=CARTESIAN_POINT ( 'NONE',  ( -14.25334919248782306, 4.085186282101443744, -6.092822981423979378 ) ) ;
#18221=CARTESIAN_POINT ( 'NONE',  ( -5.529263428287297444, 26.32731371789854791, -7.954856959092311719 ) ) ;
#18226=CARTESIAN_POINT ( 'NONE',  ( 4.622313124798831829, 27.76481371789854435, -11.61527771782809282 ) ) ;
#18228=CARTESIAN_POINT ( 'NONE',  ( -15.53471296425188442, 126.3773137178985309, -2.908627838312459080 ) ) ;
#18244=CARTESIAN_POINT ( 'NONE',  ( 14.25334919248795451, 10.51481371789855679, -6.092822981423661410 ) ) ;
#18246=CARTESIAN_POINT ( 'NONE',  ( 6.840914352312096547, 135.7601862821014720, -6.594114490232313663 ) ) ;
#18249=CARTESIAN_POINT ( 'NONE',  ( -11.48171059495397373, 22.48518628210144499, -4.944772684328680334 ) ) ;
#18253=CARTESIAN_POINT ( 'NONE',  ( -15.46528703574804986, 123.3976862821014606, -3.257655550457287497 ) ) ;
#18255=CARTESIAN_POINT ( 'NONE',  ( -5.233372021372430183, 4.947686282101431132, -8.152565276336710909 ) ) ;
#18261=CARTESIAN_POINT ( 'NONE',  ( 9.500000000000005329, 66.28981371789855359, -0.1745138560723090149 ) ) ;
#18265=CARTESIAN_POINT ( 'NONE',  ( 7.228626920338837358, 76.92731371789857064, 10.49813415416005036 ) ) ;
#18269=CARTESIAN_POINT ( 'NONE',  ( 2.660918448318002838, 40.70231371789854791, 12.46528703574811558 ) ) ;
#18276=CARTESIAN_POINT ( 'NONE',  ( -12.50000000000000355, 21.91018628210143859, -0.1745138560725492671 ) ) ;
#18281=CARTESIAN_POINT ( 'NONE',  ( 7.228626920338837358, 86.12731371789855928, 10.49813415416005036 ) ) ;
#18288=CARTESIAN_POINT ( 'NONE',  ( 13.04141134922778988, 65.42731371789857064, -8.927990412390371944 ) ) ;
#18292=CARTESIAN_POINT ( 'NONE',  ( 12.53471296425194836, 90.62268628210146915, -2.311890736173178418 ) ) ;
#18293=CARTESIAN_POINT ( 'NONE',  ( 3.257655550457285720, 24.49768628210144072, -15.46528703574804986 ) ) ;
#18298=CARTESIAN_POINT ( 'NONE',  ( -10.83675517735155047, 50.66018628210144925, -11.08355503943142750 ) ) ;
#18304=CARTESIAN_POINT ( 'NONE',  ( -12.53471296425194836, 12.42268628210144321, 2.311890736173176641 ) ) ;
#18306=CARTESIAN_POINT ( 'NONE',  ( -3.474262827703527901, 124.3648137178985849, 8.843639120294245259 ) ) ;
#18312=CARTESIAN_POINT ( 'NONE',  ( -8.715434833792127023, 134.1398137178985621, 8.962234695871568846 ) ) ;
#18317=CARTESIAN_POINT ( 'NONE',  ( 4.944772684328679446, 43.18518628210144072, -11.48171059495397373 ) ) ;
#18324=CARTESIAN_POINT ( 'NONE',  ( -10.49813415415989581, 87.17268628210143788, -7.228626920339068285 ) ) ;
#18325=CARTESIAN_POINT ( 'NONE',  ( -10.83675517735179028, 23.73981371789854222, 11.08355503943118947 ) ) ;
#18331=CARTESIAN_POINT ( 'NONE',  ( -2.064181346179062349, 8.502313717898553946, -9.465287035748106703 ) ) ;
#18336=CARTESIAN_POINT ( 'NONE',  ( 14.38691631536194393, 112.8648137178985564, 5.770363421894124656 ) ) ;
#18339=CARTESIAN_POINT ( 'NONE',  ( -10.49813415415989581, 31.97268628210143859, -7.228626920339068285 ) ) ;
#18344=CARTESIAN_POINT ( 'NONE',  ( 3.257655550457285720, 98.09768628210146346, -15.46528703574804986 ) ) ;
#18345=( NAMED_UNIT ( * ) PLANE_ANGLE_UNIT ( ) SI_UNIT ( $, .RADIAN. ) );
#18347=CARTESIAN_POINT ( 'NONE',  ( -5.233372021372430183, 50.94768628210145067, -8.152565276336710909 ) ) ;
#18351=CARTESIAN_POINT ( 'NONE',  ( -12.53471296425194836, 76.82268628210145778, 2.311890736173176641 ) ) ;
#18354=CARTESIAN_POINT ( 'NONE',  ( -9.500000000000005329, 49.51018628210145067, -0.1745138560725176813 ) ) ;
#18364=CARTESIAN_POINT ( 'NONE',  ( 4.622313124798831829, 110.5648137178985593, -11.61527771782809282 ) ) ;
#18365=CARTESIAN_POINT ( 'NONE',  ( -8.962234695871760692, 112.7601862821014720, 8.715434833791933400 ) ) ;
#18370=CARTESIAN_POINT ( 'NONE',  ( 8.632099005475788900, 74.05231371789854222, -13.23911966647199812 ) ) ;
#18373=CARTESIAN_POINT ( 'NONE',  ( 7.954856959092191815, 100.9726862821014635, 5.529263428287477744 ) ) ;
#18376=CARTESIAN_POINT ( 'NONE',  ( -8.843639120294245259, 53.06481371789855928, -3.474262827703533230 ) ) ;
#18378=CARTESIAN_POINT ( 'NONE',  ( 3.796722387233182339, 114.0148137178985763, 8.710071997420207879 ) ) ;
#18380=CARTESIAN_POINT ( 'NONE',  ( 11.61527771782809637, 30.06481371789855572, 4.622313124798827388 ) ) ;
#18383=CARTESIAN_POINT ( 'NONE',  ( 4.944772684328679446, 79.98518628210145209, -11.48171059495397373 ) ) ;
#18387=CARTESIAN_POINT ( 'NONE',  ( 6.092822981423978490, 79.98518628210145209, -14.25334919248782306 ) ) ;
#18392=CARTESIAN_POINT ( 'NONE',  ( -9.534712964251941258, 113.6226862821014549, 1.715153634034234154 ) ) ;
#18394=CARTESIAN_POINT ( 'NONE',  ( 8.962234695871762469, 135.7601862821014720, -8.715434833791931624 ) ) ;
#18407=CARTESIAN_POINT ( 'NONE',  ( 2.064181346179061460, 22.30231371789854933, 9.465287035748106703 ) ) ;
#18414=CARTESIAN_POINT ( 'NONE',  ( -4.944772684328424539, 17.41481371789854649, -11.48171059495408031 ) ) ;
#18416=CARTESIAN_POINT ( 'NONE',  ( 0.1745138560722461762, 123.7898137178985678, 15.50000000000000533 ) ) ;
#18424=CARTESIAN_POINT ( 'NONE',  ( 7.228626920339068285, 126.2726862821014606, -10.49813415415989581 ) ) ;
#18433=CARTESIAN_POINT ( 'NONE',  ( 8.715434833791931624, 138.0601862821014549, 8.962234695871760692 ) ) ;
#18437=CARTESIAN_POINT ( 'NONE',  ( -6.092822981423970496, 139.7851862821014493, 14.25334919248782661 ) ) ;
#18440=CARTESIAN_POINT ( 'NONE',  ( 3.474262827703335166, 120.2351862821014521, 8.843639120294326972 ) ) ;
#18442=CARTESIAN_POINT ( 'NONE',  ( 8.715434833791931624, 36.86018628210144499, 8.962234695871760692 ) ) ;
#18447=CARTESIAN_POINT ( 'NONE',  ( 3.257655550457285720, 116.4976862821014549, -15.46528703574804986 ) ) ;
#18449=CARTESIAN_POINT ( 'NONE',  ( 6.594114490232462877, 138.7398137178985564, -6.840914352311949109 ) ) ;
#18456=CARTESIAN_POINT ( 'NONE',  ( -7.954856959092309943, 79.22731371789853938, 5.529263428287300108 ) ) ;
#18460=CARTESIAN_POINT ( 'NONE',  ( 11.61527771782809637, 85.26481371789856212, 4.622313124798827388 ) ) ;
#18465=CARTESIAN_POINT ( 'NONE',  ( 6.932735513424201024, 55.65231371789855785, -10.69584247140429412 ) ) ;
#18470=CARTESIAN_POINT ( 'NONE',  ( 10.69584247140445221, 16.44768628210144001, -6.932735513423970097 ) ) ;
#18476=CARTESIAN_POINT ( 'NONE',  ( -0.1745138560722763466, 82.38981371789854791, -12.50000000000000355 ) ) ;
#18482=CARTESIAN_POINT ( 'NONE',  ( 13.23911966647199812, 67.15231371789852233, 8.632099005475788900 ) ) ;
#18485=CARTESIAN_POINT ( 'NONE',  ( -4.944772684328673229, 93.78518628210144925, 11.48171059495397728 ) ) ;
#18486=CARTESIAN_POINT ( 'NONE',  ( -6.092822981423970496, 29.38518628210144712, 14.25334919248782661 ) ) ;
#18490=CARTESIAN_POINT ( 'NONE',  ( 5.770363421893814682, 55.83518628210145351, 14.38691631536207183 ) ) ;
#18496=CARTESIAN_POINT ( 'NONE',  ( -11.61527771782819940, 21.33518628210144641, 4.622313124798574258 ) ) ;
#18499=CARTESIAN_POINT ( 'NONE',  ( -6.594114490232462877, 134.1398137178985621, 6.840914352311949109 ) ) ;
#18511=CARTESIAN_POINT ( 'NONE',  ( 0.1745138560725515708, 51.81018628210144783, -12.50000000000000355 ) ) ;
#18519=CARTESIAN_POINT ( 'NONE',  ( 2.311890736173175753, 74.52268628210146062, 12.53471296425194836 ) ) ;
#18520=CARTESIAN_POINT ( 'NONE',  ( 6.092822981423662299, 22.01481371789855501, 14.25334919248795096 ) ) ;
#18527=CARTESIAN_POINT ( 'NONE',  ( 12.50000000000000355, 139.8898137178985621, -0.1745138560722771515 ) ) ;
#18533=CARTESIAN_POINT ( 'NONE',  ( 10.83675517735179206, 111.1398137178985621, -11.08355503943118769 ) ) ;
#18536=CARTESIAN_POINT ( 'NONE',  ( -4.622313124798576922, 32.83518628210143930, -11.61527771782819762 ) ) ;
#18540=CARTESIAN_POINT ( 'NONE',  ( -8.927990412390661490, 112.4726862821014635, 13.04141134922759804 ) ) ;
#18544=CARTESIAN_POINT ( 'NONE',  ( 5.233372021372432847, 46.34768628210144925, 8.152565276336710909 ) ) ;
#18549=CARTESIAN_POINT ( 'NONE',  ( -4.944772684328673229, 75.38518628210144357, 11.48171059495397728 ) ) ;
#18552=CARTESIAN_POINT ( 'NONE',  ( -0.1745138560725182642, 38.01018628210144357, 9.500000000000005329 ) ) ;
#18563=CARTESIAN_POINT ( 'NONE',  ( 11.61527771782809637, 94.46481371789855075, 4.622313124798827388 ) ) ;
#18564=CARTESIAN_POINT ( 'NONE',  ( -10.69584247140444866, 113.0476862821014663, 6.932735513423972762 ) ) ;
#18569=CARTESIAN_POINT ( 'NONE',  ( 11.08355503943118769, 76.63981371789854791, 10.83675517735179028 ) ) ;
#18572=CARTESIAN_POINT ( 'NONE',  ( 8.152565276336714462, 99.24768628210145494, -5.233372021372432847 ) ) ;
#18575=CARTESIAN_POINT ( 'NONE',  ( -5.529263428287297444, 53.92731371789854222, -7.954856959092311719 ) ) ;
#18577=CARTESIAN_POINT ( 'NONE',  ( 9.465287035748106703, 112.0023137178985451, -2.064181346179063237 ) ) ;
#18579=CARTESIAN_POINT ( 'NONE',  ( -10.69584247140429412, 34.95231371789854791, -6.932735513424201024 ) ) ;
#18580=CARTESIAN_POINT ( 'NONE',  ( -11.61527771782819940, 85.73518628210143788, 4.622313124798574258 ) ) ;
#18588=CARTESIAN_POINT ( 'NONE',  ( -8.710071997420127943, 96.08518628210146062, -3.796722387233380402 ) ) ;
#18590=CARTESIAN_POINT ( 'NONE',  ( -12.50000000000000355, 123.1101862821014663, -0.1745138560725492671 ) ) ;
#18603=CARTESIAN_POINT ( 'NONE',  ( -5.529263428287297444, 17.12731371789855217, -7.954856959092311719 ) ) ;
#18608=CARTESIAN_POINT ( 'NONE',  ( -4.622313124798826500, 32.36481371789854933, 11.61527771782809637 ) ) ;
#18610=CARTESIAN_POINT ( 'NONE',  ( -0.1745138560722442889, 128.3898137178985621, -15.50000000000000533 ) ) ;
#18618=CARTESIAN_POINT ( 'NONE',  ( -2.660918448318275509, 139.4976862821014549, 12.46528703574805874 ) ) ;
#18626=CARTESIAN_POINT ( 'NONE',  ( 10.49813415415989581, 137.7726862821014606, 7.228626920339068285 ) ) ;
#18631=CARTESIAN_POINT ( 'NONE',  ( -6.092822981423970496, 130.5851862821014606, 14.25334919248782661 ) ) ;
#18633=CARTESIAN_POINT ( 'NONE',  ( 8.152565276336714462, 117.6476862821014322, -5.233372021372432847 ) ) ;
#18635=CARTESIAN_POINT ( 'NONE',  ( -8.715434833791929847, 32.26018628210145067, -8.962234695871762469 ) ) ;
#18639=CARTESIAN_POINT ( 'NONE',  ( -14.25334919248782306, 114.4851862821014663, -6.092822981423979378 ) ) ;
#18641=CARTESIAN_POINT ( 'NONE',  ( 5.529263428287477744, 6.672686282101436106, -7.954856959092191815 ) ) ;
#18648=CARTESIAN_POINT ( 'NONE',  ( -8.710071997420207879, 70.31481371789853085, 3.796722387233182339 ) ) ;
#18651=CARTESIAN_POINT ( 'NONE',  ( 2.311890736173452421, 82.67731371789854222, -12.53471296425189152 ) ) ;
#18655=CARTESIAN_POINT ( 'NONE',  ( -8.715434833792127023, 51.33981371789855785, 8.962234695871568846 ) ) ;
#18661=CARTESIAN_POINT ( 'NONE',  ( 6.932735513423970097, 18.74768628210143717, 10.69584247140445044 ) ) ;
#18665=CARTESIAN_POINT ( 'NONE',  ( -6.932735513424201912, 78.65231371789855075, 10.69584247140429412 ) ) ;
#18671=CARTESIAN_POINT ( 'NONE',  ( 11.08355503943118769, 49.03981371789855359, 10.83675517735179028 ) ) ;
#18674=CARTESIAN_POINT ( 'NONE',  ( 0.1745138560725515708, 79.41018628210144925, -12.50000000000000355 ) ) ;
#18675=CARTESIAN_POINT ( 'NONE',  ( -15.53471296425195369, 21.62268628210143717, 2.908627838312118019 ) ) ;
#18680=CARTESIAN_POINT ( 'NONE',  ( -15.50000000000000533, 40.31018628210145494, -0.1745138560725808530 ) ) ;
#18687=CARTESIAN_POINT ( 'NONE',  ( -12.46528703574805697, 22.19768628210145067, -2.660918448318280838 ) ) ;
#18689=CARTESIAN_POINT ( 'NONE',  ( 5.233372021372610483, 138.4523137178985621, -8.152565276336593669 ) ) ;
#18694=CARTESIAN_POINT ( 'NONE',  ( -0.1745138560722763466, 128.3898137178985621, -12.50000000000000355 ) ) ;
#18700=CARTESIAN_POINT ( 'NONE',  ( -12.50000000000000355, 49.51018628210145067, -0.1745138560725492671 ) ) ;
#18709=CARTESIAN_POINT ( 'NONE',  ( -10.69584247140444866, 85.44768628210144357, 6.932735513423972762 ) ) ;
#18710=CARTESIAN_POINT ( 'NONE',  ( 14.38691631536207538, 136.3351862821014606, -5.770363421893813793 ) ) ;
#18717=CARTESIAN_POINT ( 'NONE',  ( -4.622313124798826500, 133.5648137178985735, 11.61527771782809637 ) ) ;
#18723=CARTESIAN_POINT ( 'NONE',  ( -13.04141134922778456, 116.0273137178985792, 8.927990412390377273 ) ) ;
#18730=CARTESIAN_POINT ( 'NONE',  ( -11.08355503943142573, 112.7601862821014720, 10.83675517735155402 ) ) ;
#18733=CARTESIAN_POINT ( 'NONE',  ( 8.843639120294328748, 35.13518628210143646, -3.474262827703334722 ) ) ;
#18737=CARTESIAN_POINT ( 'NONE',  ( 4.944772684328679446, 70.78518628210144925, -11.48171059495397373 ) ) ;
#18740=CARTESIAN_POINT ( 'NONE',  ( 2.064181346179272847, 42.89768628210143220, -9.465287035748065847 ) ) ;
#18750=CARTESIAN_POINT ( 'NONE',  ( 11.48171059495408208, 93.31481371789855928, -4.944772684328420986 ) ) ;
#18751=CARTESIAN_POINT ( 'NONE',  ( 4.944772684328679446, 98.38518628210145778, -11.48171059495397373 ) ) ;
#18756=CARTESIAN_POINT ( 'NONE',  ( 2.908627838312458636, 82.67731371789852801, -15.53471296425188442 ) ) ;
#18760=ADVANCED_BREP_SHAPE_REPRESENTATION ( '', ( #21172, #17215 ), #1426 ) ;
#18762=CARTESIAN_POINT ( 'NONE',  ( 9.465287035748106703, 66.00231371789855928, -2.064181346179063237 ) ) ;
#18765=CARTESIAN_POINT ( 'NONE',  ( 6.594114490232462877, 120.3398137178985507, -6.840914352311949109 ) ) ;
#18767=CARTESIAN_POINT ( 'NONE',  ( 4.944772684328420986, 31.21481371789855430, 11.48171059495408208 ) ) ;
#18770=CARTESIAN_POINT ( 'NONE',  ( -12.53471296425194836, 86.02268628210146062, 2.311890736173176641 ) ) ;
#18775=PRODUCT_DEFINITION ( 'UNKNOWN', '', #4487, #32371 ) ;
#18779=CARTESIAN_POINT ( 'NONE',  ( -9.534712964251941258, 95.22268628210143504, 1.715153634034234154 ) ) ;
#18781=CARTESIAN_POINT ( 'NONE',  ( -4.944772684328673229, 130.5851862821014606, 11.48171059495397728 ) ) ;
#18792=CARTESIAN_POINT ( 'NONE',  ( -8.152565276336593669, 7.352313717898546486, -5.233372021372610483 ) ) ;
#18798=CARTESIAN_POINT ( 'NONE',  ( -8.715434833792127023, 32.93981371789854506, 8.962234695871568846 ) ) ;
#18800=CARTESIAN_POINT ( 'NONE',  ( -3.257655550456946880, 128.1023137178985678, -15.46528703574811736 ) ) ;
#18807=CARTESIAN_POINT ( 'NONE',  ( 12.50000000000000355, 127.7101862821014606, 0.1745138560725507937 ) ) ;
#18814=CARTESIAN_POINT ( 'NONE',  ( -12.50000000000000355, 141.5101862821014720, -0.1745138560725492671 ) ) ;
#18817=CARTESIAN_POINT ( 'NONE',  ( -14.25334919248782306, 114.4851862821014663, -6.092822981423979378 ) ) ;
#18819=CARTESIAN_POINT ( 'NONE',  ( -5.233372021372430183, 115.3476862821014493, -8.152565276336710909 ) ) ;
#18821=CARTESIAN_POINT ( 'NONE',  ( 11.61527771782819940, 7.535186282101452804, -4.622313124798573369 ) ) ;
#18825=CARTESIAN_POINT ( 'NONE',  ( -6.594114490232312775, 87.46018628210146062, -6.840914352312096547 ) ) ;
#18827=CARTESIAN_POINT ( 'NONE',  ( -9.500000000000005329, 126.0898137178985650, 0.1745138560723101806 ) ) ;
#18834=CARTESIAN_POINT ( 'NONE',  ( -5.529263428287297444, 72.32731371789854791, -7.954856959092311719 ) ) ;
#18837=CARTESIAN_POINT ( 'NONE',  ( -10.49813415416004858, 79.22731371789855359, 7.228626920338840023 ) ) ;
#18839=CARTESIAN_POINT ( 'NONE',  ( -9.862825201705371470, 142.9999999999999716, 9.257821876896041857 ) ) ;
#18841=CARTESIAN_POINT ( 'NONE',  ( -8.962234695871565293, 44.43981371789855217, -8.715434833792128799 ) ) ;
#18846=CARTESIAN_POINT ( 'NONE',  ( 2.660918448318279950, 15.29768628210143078, -12.46528703574805697 ) ) ;
#18850=CARTESIAN_POINT ( 'NONE',  ( -11.48171059495408208, 70.31481371789854506, 4.944772684328421875 ) ) ;
#18855=CARTESIAN_POINT ( 'NONE',  ( 15.46528703574811736, 66.00231371789855928, -3.257655550456947768 ) ) ;
#18858=CARTESIAN_POINT ( 'NONE',  ( -2.660918448318275509, 65.89768628210146062, 12.46528703574805874 ) ) ;
#18859=CARTESIAN_POINT ( 'NONE',  ( 2.908627838312118019, 28.52268628210144286, 15.53471296425195369 ) ) ;
#18864=CARTESIAN_POINT ( 'NONE',  ( -3.257655550457281723, 38.29768628210144499, 15.46528703574804986 ) ) ;
#18870=CARTESIAN_POINT ( 'NONE',  ( -4.622313124798576922, 23.63518628210144357, -11.61527771782819762 ) ) ;
#18872=CARTESIAN_POINT ( 'NONE',  ( -8.710071997420207879, 134.7148137178985507, 3.796722387233182339 ) ) ;
#18876=CARTESIAN_POINT ( 'NONE',  ( 11.48171059495408208, 139.3148137178985451, -4.944772684328420986 ) ) ;
#18883=CARTESIAN_POINT ( 'NONE',  ( 4.944772684328679446, 33.98518628210143788, -11.48171059495397373 ) ) ;
#18892=CARTESIAN_POINT ( 'NONE',  ( 8.715434833791931624, 82.86018628210145209, 8.962234695871760692 ) ) ;
#18893=CARTESIAN_POINT ( 'NONE',  ( -14.38691631536207183, 131.7351862821014663, 5.770363421893814682 ) ) ;
#18900=CARTESIAN_POINT ( 'NONE',  ( 2.311890736173452865, 137.8773137178986019, -12.53471296425189152 ) ) ;
#18906=CARTESIAN_POINT ( 'NONE',  ( 5.770363421894130873, 110.5648137178985593, -14.38691631536193860 ) ) ;
#18911=CARTESIAN_POINT ( 'NONE',  ( -11.61527771782819940, 131.7351862821014663, 4.622313124798574258 ) ) ;
#18914=CARTESIAN_POINT ( 'NONE',  ( 13.04141134922759804, 100.9726862821014635, 8.927990412390657937 ) ) ;
#18918=CARTESIAN_POINT ( 'NONE',  ( -1.715153634034234598, 33.12268628210143362, -9.534712964251941258 ) ) ;
#18922=CARTESIAN_POINT ( 'NONE',  ( -11.48171059495397373, 68.48518628210145209, -4.944772684328680334 ) ) ;
#18925=CARTESIAN_POINT ( 'NONE',  ( 1.715153634034233487, 46.92268628210143788, 9.534712964251941258 ) ) ;
#18933=CARTESIAN_POINT ( 'NONE',  ( 10.69584247140429589, 76.35231371789855359, 6.932735513424201024 ) ) ;
#18934=CARTESIAN_POINT ( 'NONE',  ( 11.48171059495397728, 91.48518628210145209, 4.944772684328674117 ) ) ;
#18940=CARTESIAN_POINT ( 'NONE',  ( 5.770363421894130873, 55.36481371789856354, -14.38691631536193860 ) ) ;
#18945=CARTESIAN_POINT ( 'NONE',  ( -8.710071997420207879, 61.11481371789854933, 3.796722387233182339 ) ) ;
#18948=CARTESIAN_POINT ( 'NONE',  ( -8.843639120294245259, 117.4648137178985650, -3.474262827703533230 ) ) ;
#18950=CARTESIAN_POINT ( 'NONE',  ( 2.660918448318002838, 31.50231371789854862, 12.46528703574811558 ) ) ;
#18951=CARTESIAN_POINT ( 'NONE',  ( -10.49813415415989581, 77.97268628210144925, -7.228626920339068285 ) ) ;
#18958=CARTESIAN_POINT ( 'NONE',  ( -1.715153634034234598, 97.52268628210144641, -9.534712964251941258 ) ) ;
#18961=CARTESIAN_POINT ( 'NONE',  ( 12.46528703574805874, 137.1976862821014720, 2.660918448318279950 ) ) ;
#18962=CARTESIAN_POINT ( 'NONE',  ( -6.520765304352172720, 143.0000000000000284, 10.25440256910218828 ) ) ;
#18971=CARTESIAN_POINT ( 'NONE',  ( -11.48171059495408208, 134.7148137178985507, 4.944772684328421875 ) ) ;
#18972=CARTESIAN_POINT ( 'NONE',  ( -0.1745138560725500443, 139.2101862821014606, 12.50000000000000355 ) ) ;
#18979=CARTESIAN_POINT ( 'NONE',  ( 8.632099005475788900, 110.8523137178985252, -13.23911966647199812 ) ) ;
#18987=CARTESIAN_POINT ( 'NONE',  ( 8.715434833791931624, 138.0601862821014549, 8.962234695871760692 ) ) ;
#18995=CARTESIAN_POINT ( 'NONE',  ( -4.622313124798576922, 134.0351862821014493, -11.61527771782819762 ) ) ;
#19000=CARTESIAN_POINT ( 'NONE',  ( -13.23911966647218463, 122.2476862821014691, 8.632099005475506459 ) ) ;
#19001=CARTESIAN_POINT ( 'NONE',  ( 7.954856959092191815, 110.1726862821014663, 5.529263428287477744 ) ) ;
#19003=CARTESIAN_POINT ( 'NONE',  ( 8.962234695871762469, 16.16018628210144570, -8.715434833791931624 ) ) ;
#19007=CARTESIAN_POINT ( 'NONE',  ( 2.064181346179272847, 79.69768628210141515, -9.465287035748065847 ) ) ;
#19010=CARTESIAN_POINT ( 'NONE',  ( -1.715153634034442431, 124.0773137178985621, 9.534712964251900402 ) ) ;
#19018=CARTESIAN_POINT ( 'NONE',  ( -7.954856959092309943, 60.82731371789854080, 5.529263428287300108 ) ) ;
#19021=CARTESIAN_POINT ( 'NONE',  ( 10.49813415416005213, 83.82731371789856212, -7.228626920338837358 ) ) ;
#19025=CARTESIAN_POINT ( 'NONE',  ( 0.1745138560722779009, 22.58981371789854720, 12.50000000000000355 ) ) ;
#19030=CARTESIAN_POINT ( 'NONE',  ( 0.1745138560725515708, 24.21018628210144641, -12.50000000000000355 ) ) ;
#19038=CARTESIAN_POINT ( 'NONE',  ( -12.53471296425189152, 61.97731371789854649, -2.311890736173453753 ) ) ;
#19044=CARTESIAN_POINT ( 'NONE',  ( -15.46528703574811736, 43.00231371789853796, 3.257655550456946436 ) ) ;
#19047=CARTESIAN_POINT ( 'NONE',  ( 12.46528703574805874, 72.79768628210146630, 2.660918448318279950 ) ) ;
#19048=CARTESIAN_POINT ( 'NONE',  ( -13.23911966647218463, 11.84768628210144747, 8.632099005475506459 ) ) ;
#19053=CARTESIAN_POINT ( 'NONE',  ( -5.770363421893818234, 32.83518628210143930, -14.38691631536207005 ) ) ;
#19058=CARTESIAN_POINT ( 'NONE',  ( -4.944772684328673229, 10.98518628210143433, 11.48171059495397728 ) ) ;
#19060=CARTESIAN_POINT ( 'NONE',  ( -9.500000000000005329, 107.6898137178985735, 0.1745138560723101806 ) ) ;
#19070=CARTESIAN_POINT ( 'NONE',  ( 10.49813415415989581, 36.57268628210144357, 7.228626920339069173 ) ) ;
#19078=CARTESIAN_POINT ( 'NONE',  ( 2.660918448318279950, 70.49768628210145494, -12.46528703574805697 ) ) ;
#19079=CARTESIAN_POINT ( 'NONE',  ( 8.632099005475788900, 9.652313717898541867, -13.23911966647199812 ) ) ;
#19085=CARTESIAN_POINT ( 'NONE',  ( -11.61527771782809282, 117.4648137178985650, -4.622313124798832717 ) ) ;
#19090=CARTESIAN_POINT ( 'NONE',  ( -15.46528703574811736, 89.00231371789853085, 3.257655550456946436 ) ) ;
#19095=CARTESIAN_POINT ( 'NONE',  ( 2.311890736173175753, 120.5226862821014606, 12.53471296425194836 ) ) ;
#19097=CARTESIAN_POINT ( 'NONE',  ( -8.927990412390661490, 84.87268628210145494, 13.04141134922759804 ) ) ;
#19101=CARTESIAN_POINT ( 'NONE',  ( -5.770363421893818234, 78.83518628210146062, -14.38691631536207005 ) ) ;
#19104=CARTESIAN_POINT ( 'NONE',  ( -3.474262827703337830, 32.83518628210143930, -8.843639120294326972 ) ) ;
#19108=CARTESIAN_POINT ( 'NONE',  ( -0.1745138560725500443, 65.61018628210145209, 12.50000000000000355 ) ) ;
#19111=CARTESIAN_POINT ( 'NONE',  ( -0.1745138560725182642, 47.21018628210144641, 9.500000000000005329 ) ) ;
#19121=CARTESIAN_POINT ( 'NONE',  ( 10.49813415416005213, 93.02731371789856496, -7.228626920338837358 ) ) ;
#19122=CARTESIAN_POINT ( 'NONE',  ( -6.932735513423968321, 87.74768628210144072, -10.69584247140445221 ) ) ;
#19128=CARTESIAN_POINT ( 'NONE',  ( 15.50000000000000533, 66.28981371789855359, -0.1745138560722452326 ) ) ;
#19135=CARTESIAN_POINT ( 'NONE',  ( 8.843639120294245259, 39.26481371789855501, 3.474262827703527901 ) ) ;
#19137=CARTESIAN_POINT ( 'NONE',  ( 5.233372021372610483, 92.45231371789854791, -8.152565276336593669 ) ) ;
#19139=CARTESIAN_POINT ( 'NONE',  ( -4.622313124798826500, 23.16481371789855359, 11.61527771782809637 ) ) ;
#19140=CARTESIAN_POINT ( 'NONE',  ( -2.660918448318275509, 75.09768628210143504, 12.46528703574805874 ) ) ;
#19148=CARTESIAN_POINT ( 'NONE',  ( 3.796722387233379514, 98.38518628210145778, -8.710071997420127943 ) ) ;
#19151=CARTESIAN_POINT ( 'NONE',  ( -11.61527771782819940, 122.5351862821014635, 4.622313124798574258 ) ) ;
#19163=CARTESIAN_POINT ( 'NONE',  ( 1.715153634034445762, 9.077313717898549683, -9.534712964251895073 ) ) ;
#19170=CARTESIAN_POINT ( 'NONE',  ( -0.1745138560722763466, 8.789813717898553591, -12.50000000000000355 ) ) ;
#19172=CARTESIAN_POINT ( 'NONE',  ( 11.08355503943118769, 104.2398137178985706, 10.83675517735179028 ) ) ;
#19177=CARTESIAN_POINT ( 'NONE',  ( -10.69584247140444866, 122.2476862821014549, 6.932735513423972762 ) ) ;
#19190=CARTESIAN_POINT ( 'NONE',  ( 5.770363421893814682, 120.2351862821014521, 14.38691631536207183 ) ) ;
#19194=CARTESIAN_POINT ( 'NONE',  ( 4.622313124798573369, 9.835186282101449962, 11.61527771782819940 ) ) ;
#19198=CARTESIAN_POINT ( 'NONE',  ( 5.233372021372432847, 83.14768628210143220, 8.152565276336710909 ) ) ;
#19200=CARTESIAN_POINT ( 'NONE',  ( -3.474262827703527901, 124.3648137178985849, 8.843639120294245259 ) ) ;
#19206=CARTESIAN_POINT ( 'NONE',  ( -9.465287035748106703, 52.20231371789854080, 2.064181346179061460 ) ) ;
#19212=CARTESIAN_POINT ( 'NONE',  ( 4.944772684328420986, 58.81481371789855217, 11.48171059495408208 ) ) ;
#19216=CARTESIAN_POINT ( 'NONE',  ( -11.48171059495408208, 33.51481371789854791, 4.944772684328421875 ) ) ;
#19226=CARTESIAN_POINT ( 'NONE',  ( -2.311890736173448424, 68.87731371789855928, 12.53471296425189330 ) ) ;
#19231=CARTESIAN_POINT ( 'NONE',  ( 15.50000000000000533, 47.88981371789855501, -0.1745138560722452326 ) ) ;
#19233=CARTESIAN_POINT ( 'NONE',  ( 11.61527771782819940, 25.93518628210143717, -4.622313124798573369 ) ) ;
#19235=CARTESIAN_POINT ( 'NONE',  ( -12.53471296425194836, 67.62268628210145494, 2.311890736173176641 ) ) ;
#19237=CARTESIAN_POINT ( 'NONE',  ( 13.04141134922759804, 8.972686282101431487, 8.927990412390657937 ) ) ;
#19241=CARTESIAN_POINT ( 'NONE',  ( 13.23911966647218996, 25.64768628210144286, -8.632099005475504683 ) ) ;
#19248=CARTESIAN_POINT ( 'NONE',  ( -12.50000000000000355, 3.510186282101451560, -0.1745138560725492671 ) ) ;
#19251=CARTESIAN_POINT ( 'NONE',  ( 7.954856959092311719, 120.6273137178985451, -5.529263428287300108 ) ) ;
#19256=CARTESIAN_POINT ( 'NONE',  ( -8.962234695871565293, 108.8398137178985507, -8.715434833792128799 ) ) ;
#19262=CARTESIAN_POINT ( 'NONE',  ( 11.61527771782819940, 35.13518628210143646, -4.622313124798573369 ) ) ;
#19270=CARTESIAN_POINT ( 'NONE',  ( -12.46528703574805697, 68.19768628210144357, -2.660918448318280838 ) ) ;
#19271=CARTESIAN_POINT ( 'NONE',  ( 8.632099005475504683, 138.3476862821014208, 13.23911966647218996 ) ) ;
#19277=CARTESIAN_POINT ( 'NONE',  ( 11.61527771782809637, 131.2648137178985621, 4.622313124798827388 ) ) ;
#19285=CARTESIAN_POINT ( 'NONE',  ( 5.770363421894130873, 101.3648137178985706, -14.38691631536193860 ) ) ;
#19289=CARTESIAN_POINT ( 'NONE',  ( -12.53471296425194836, 122.8226862821014720, 2.311890736173176641 ) ) ;
#19290=CARTESIAN_POINT ( 'NONE',  ( -13.04141134922759804, 59.57268628210145067, -8.927990412390657937 ) ) ;
#19293=CARTESIAN_POINT ( 'NONE',  ( -8.632099005475501130, 87.74768628210144072, -13.23911966647218996 ) ) ;
#19296=CARTESIAN_POINT ( 'NONE',  ( 8.152565276336714462, 34.84768628210143504, -5.233372021372432847 ) ) ;
#19301=CARTESIAN_POINT ( 'NONE',  ( 12.46528703574805874, 63.59768628210145636, 2.660918448318279950 ) ) ;
#19304=CARTESIAN_POINT ( 'NONE',  ( 9.500000000000005329, 26.51018628210144001, 0.1745138560725188748 ) ) ;
#19314=CARTESIAN_POINT ( 'NONE',  ( -0.1745138560722763466, 91.58981371789856496, -12.50000000000000355 ) ) ;
#19315=CARTESIAN_POINT ( 'NONE',  ( 4.944772684328679446, 89.18518628210145494, -11.48171059495397373 ) ) ;
#19320=CARTESIAN_POINT ( 'NONE',  ( 8.632099005475788900, 64.85231371789855359, -13.23911966647199812 ) ) ;
#19326=CARTESIAN_POINT ( 'NONE',  ( 3.796722387233182339, 40.41481371789855359, 8.710071997420207879 ) ) ;
#19328=CARTESIAN_POINT ( 'NONE',  ( -5.529263428287297444, 99.92731371789854222, -7.954856959092311719 ) ) ;
#19330=CARTESIAN_POINT ( 'NONE',  ( 10.49813415416005213, 19.42731371789854933, -7.228626920338837358 ) ) ;
#19331=CARTESIAN_POINT ( 'NONE',  ( 2.311890736173175753, 56.12268628210144072, 12.53471296425194836 ) ) ;
#19339=CARTESIAN_POINT ( 'NONE',  ( 6.840914352312096547, 89.76018628210145778, -6.594114490232313663 ) ) ;
#19341=CARTESIAN_POINT ( 'NONE',  ( 6.932735513423970097, 110.7476862821014549, 10.69584247140445044 ) ) ;
#19342=CARTESIAN_POINT ( 'NONE',  ( -6.397436014819822603, 142.9999999999999432, 10.66666770903068162 ) ) ;
#19353=CARTESIAN_POINT ( 'NONE',  ( 11.61527771782809637, 140.4648137178985792, 4.622313124798827388 ) ) ;
#19358=CARTESIAN_POINT ( 'NONE',  ( 12.53471296425189330, 11.37731371789854684, 2.311890736173451533 ) ) ;
#19360=CARTESIAN_POINT ( 'NONE',  ( -13.23911966647199812, 117.7523137178985735, -8.632099005475788900 ) ) ;
#19367=CARTESIAN_POINT ( 'NONE',  ( 6.932735513423970097, 110.7476862821014549, 10.69584247140445044 ) ) ;
#19373=CARTESIAN_POINT ( 'NONE',  ( -10.49813415415989581, 114.7726862821014606, -7.228626920339068285 ) ) ;
#19379=CARTESIAN_POINT ( 'NONE',  ( 13.23911966647218996, 117.6476862821014322, -8.632099005475504683 ) ) ;
#19382=CARTESIAN_POINT ( 'NONE',  ( -9.534712964251941258, 141.2226862821014493, 1.715153634034234154 ) ) ;
#19387=CARTESIAN_POINT ( 'NONE',  ( 7.954856959092191815, 82.57268628210144357, 5.529263428287477744 ) ) ;
#19388=CARTESIAN_POINT ( 'NONE',  ( 5.233372021372610483, 129.2523137178985451, -8.152565276336593669 ) ) ;
#19394=CARTESIAN_POINT ( 'NONE',  ( -9.500000000000005329, 52.48981371789855643, 0.1745138560723101806 ) ) ;
#19398=CARTESIAN_POINT ( 'NONE',  ( 10.69584247140429589, 57.95231371789854791, 6.932735513424201024 ) ) ;
#19402=CARTESIAN_POINT ( 'NONE',  ( 6.932735513424201024, 37.25231371789855217, -10.69584247140429412 ) ) ;
#19405=CARTESIAN_POINT ( 'NONE',  ( -0.1745138560725500443, 10.41018628210144215, 12.50000000000000355 ) ) ;
#19407=CARTESIAN_POINT ( 'NONE',  ( -0.1745138560722763466, 63.98981371789854933, -12.50000000000000355 ) ) ;
#19412=CARTESIAN_POINT ( 'NONE',  ( -8.632099005475794229, 41.85231371789854649, 13.23911966647199812 ) ) ;
#19415=CARTESIAN_POINT ( 'NONE',  ( 12.50000000000000355, 26.51018628210144357, 0.1745138560725507937 ) ) ;
#19417=CARTESIAN_POINT ( 'NONE',  ( -8.962234695871760692, 75.96018628210144641, 8.715434833791933400 ) ) ;
#19418=CARTESIAN_POINT ( 'NONE',  ( 8.927990412390657937, 6.672686282101436106, -13.04141134922759804 ) ) ;
#19422=CARTESIAN_POINT ( 'NONE',  ( 15.46528703574804986, 35.99768628210143362, 3.257655550457285720 ) ) ;
#19428=CARTESIAN_POINT ( 'NONE',  ( 12.46528703574805874, 8.397686282101442856, 2.660918448318279950 ) ) ;
#19430=CARTESIAN_POINT ( 'NONE',  ( 3.474262827703532341, 110.5648137178985593, -8.843639120294245259 ) ) ;
#19437=CARTESIAN_POINT ( 'NONE',  ( -12.50000000000000355, 116.8898137178985621, 0.1745138560722786503 ) ) ;
#19443=CARTESIAN_POINT ( 'NONE',  ( 6.932735513423970097, 37.14768628210143930, 10.69584247140445044 ) ) ;
#19451=CARTESIAN_POINT ( 'NONE',  ( 4.944772684328679446, 52.38518628210145067, -11.48171059495397373 ) ) ;
#19458=CARTESIAN_POINT ( 'NONE',  ( 0.1745138560722779009, 114.5898137178985650, 12.50000000000000355 ) ) ;
#19465=CARTESIAN_POINT ( 'NONE',  ( 8.927990412390371944, 95.32731371789854791, 13.04141134922778811 ) ) ;
#19469=CARTESIAN_POINT ( 'NONE',  ( 10.69584247140445221, 126.8476862821014635, -6.932735513423970097 ) ) ;
#19470=CARTESIAN_POINT ( 'NONE',  ( 0.1745138560725837118, 70.21018628210144641, -15.50000000000000533 ) ) ;
#19473=CARTESIAN_POINT ( 'NONE',  ( 14.25334919248782661, 91.48518628210145209, 6.092822981423971385 ) ) ;
#19477=CARTESIAN_POINT ( 'NONE',  ( -8.710071997420127943, 13.28518628210143149, -3.796722387233380402 ) ) ;
#19480=CARTESIAN_POINT ( 'NONE',  ( -7.228626920339069173, 57.27268628210144641, 10.49813415415989581 ) ) ;
#19483=CARTESIAN_POINT ( 'NONE',  ( -5.233372021372430183, 23.34768628210144570, -8.152565276336710909 ) ) ;
#19495=CARTESIAN_POINT ( 'NONE',  ( -10.69584247140429412, 80.95231371789856212, -6.932735513424201024 ) ) ;
#19496=CARTESIAN_POINT ( 'NONE',  ( -11.61527771782819940, 94.93518628210145494, 4.622313124798574258 ) ) ;
#19501=CARTESIAN_POINT ( 'NONE',  ( -15.53471296425188442, 52.77731371789855785, -2.908627838312459080 ) ) ;
#19507=CARTESIAN_POINT ( 'NONE',  ( -5.529263428287297444, 44.72731371789853938, -7.954856959092311719 ) ) ;
#19509=CARTESIAN_POINT ( 'NONE',  ( -9.465287035748106703, 89.00231371789853085, 2.064181346179061460 ) ) ;
#19511=CARTESIAN_POINT ( 'NONE',  ( -12.50000000000000355, 15.68981371789854329, 0.1745138560722786503 ) ) ;
#19513=CARTESIAN_POINT ( 'NONE',  ( 6.932735513423970097, 55.54768628210144499, 10.69584247140445044 ) ) ;
#19521=CARTESIAN_POINT ( 'NONE',  ( 9.500000000000005329, 72.51018628210145778, 0.1745138560725188748 ) ) ;
#19523=CARTESIAN_POINT ( 'NONE',  ( -4.622313124798576922, 115.6351862821014578, -11.61527771782819762 ) ) ;
#19534=CARTESIAN_POINT ( 'NONE',  ( -12.53471296425189152, 135.5773137178985621, -2.311890736173453753 ) ) ;
#19535=CARTESIAN_POINT ( 'NONE',  ( 4.622313124798573369, 138.6351862821014720, 11.61527771782819940 ) ) ;
#19540=CARTESIAN_POINT ( 'NONE',  ( 8.962234695871567070, 12.23981371789853512, 8.715434833792127023 ) ) ;
#19542=CARTESIAN_POINT ( 'NONE',  ( 13.23911966647199812, 113.1523137178985650, 8.632099005475788900 ) ) ;
#19548=CARTESIAN_POINT ( 'NONE',  ( -4.622313124798576922, 115.6351862821014578, -11.61527771782819762 ) ) ;
#19554=CARTESIAN_POINT ( 'NONE',  ( -4.622313124798576922, 124.8351862821014748, -11.61527771782819762 ) ) ;
#19558=CARTESIAN_POINT ( 'NONE',  ( -15.50000000000000533, 113.9101862821014493, -0.1745138560725808530 ) ) ;
#19560=CARTESIAN_POINT ( 'NONE',  ( -8.962234695871760692, 11.56018628210145316, 8.715434833791933400 ) ) ;
#19567=CARTESIAN_POINT ( 'NONE',  ( 5.233372021372432847, 73.94768628210142936, 8.152565276336710909 ) ) ;
#19574=CARTESIAN_POINT ( 'NONE',  ( -3.796722387233185003, 54.21481371789855785, -8.710071997420207879 ) ) ;
#19578=CARTESIAN_POINT ( 'NONE',  ( -0.1745138560722763466, 54.78981371789855359, -12.50000000000000355 ) ) ;
#19581=CARTESIAN_POINT ( 'NONE',  ( -10.49813415416004858, 33.22731371789855359, 7.228626920338839135 ) ) ;
#19593=CARTESIAN_POINT ( 'NONE',  ( 12.50000000000000355, 66.28981371789855359, -0.1745138560722771515 ) ) ;
#19598=CARTESIAN_POINT ( 'NONE',  ( -11.08355503943118592, 44.43981371789855928, -10.83675517735179383 ) ) ;
#19601=CARTESIAN_POINT ( 'NONE',  ( 10.49813415415989581, 18.17268628210144854, 7.228626920339068285 ) ) ;
#19602=CARTESIAN_POINT ( 'NONE',  ( 12.50000000000000355, 63.31018628210144072, 0.1745138560725507937 ) ) ;
#19604=CARTESIAN_POINT ( 'NONE',  ( -12.50000000000000355, 141.5101862821014720, -0.1745138560725492671 ) ) ;
#19608=CARTESIAN_POINT ( 'NONE',  ( 15.53471296425195369, 35.42268628210144499, -2.908627838312120684 ) ) ;
#19618=CARTESIAN_POINT ( 'NONE',  ( 6.594114490232462877, 120.3398137178985507, -6.840914352311949109 ) ) ;
#19624=CARTESIAN_POINT ( 'NONE',  ( 12.50000000000000355, 112.2898137178985678, -0.1745138560722771515 ) ) ;
#19628=DIRECTION ( 'NONE',  ( 0.000000000000000000, -0.9932091452657081376, -0.1163425707149433747 ) ) ;
#19640=CARTESIAN_POINT ( 'NONE',  ( 11.48171059495397728, 54.68518628210144783, 4.944772684328674117 ) ) ;
#19645=DIRECTION ( 'NONE',  ( 1.000000000000000000, 0.000000000000000000, 0.000000000000000000 ) ) ;
#19647=CARTESIAN_POINT ( 'NONE',  ( 12.46528703574811558, 130.4023137178985792, -2.660918448318005503 ) ) ;
#19652=CARTESIAN_POINT ( 'NONE',  ( 8.632099005475788900, 92.45231371789854791, -13.23911966647199812 ) ) ;
#19656=CARTESIAN_POINT ( 'NONE',  ( 8.962234695871762469, 117.3601862821014521, -8.715434833791931624 ) ) ;
#19657=CARTESIAN_POINT ( 'NONE',  ( -2.908627838312119351, 69.92268628210143788, -15.53471296425195369 ) ) ;
#19660=CARTESIAN_POINT ( 'NONE',  ( 15.53471296425195369, 81.42268628210145209, -2.908627838312120684 ) ) ;
#19664=CARTESIAN_POINT ( 'NONE',  ( -3.796722387233375073, 20.18518628210144783, 8.710071997420127943 ) ) ;
#19668=CARTESIAN_POINT ( 'NONE',  ( 12.50000000000000355, 63.31018628210144072, 0.1745138560725507937 ) ) ;
#19671=CARTESIAN_POINT ( 'NONE',  ( -9.500000000000005329, 21.91018628210143859, -0.1745138560725176813 ) ) ;
#19682=CARTESIAN_POINT ( 'NONE',  ( -12.53471296425194659, 95.22268628210144925, 2.311890736173176641 ) ) ;
#19688=CARTESIAN_POINT ( 'NONE',  ( 6.092822981423662299, 40.41481371789855359, 14.25334919248795096 ) ) ;
#19694=CARTESIAN_POINT ( 'NONE',  ( -6.594114490232462877, 42.13981371789854791, 6.840914352311949109 ) ) ;
#19696=CARTESIAN_POINT ( 'NONE',  ( -9.500000000000005329, 98.48981371789855643, 0.1745138560723101806 ) ) ;
#19698=CARTESIAN_POINT ( 'NONE',  ( -10.83675517735179028, 143.3398137178985507, 11.08355503943118947 ) ) ;
#19701=CARTESIAN_POINT ( 'NONE',  ( 4.622313124798573369, 65.03518628210144925, 11.61527771782819940 ) ) ;
#19709=CARTESIAN_POINT ( 'NONE',  ( -2.064181346179269738, 84.29768628210146630, 9.465287035748067623 ) ) ;
#19712=CARTESIAN_POINT ( 'NONE',  ( 10.69584247140445221, 108.4476862821014578, -6.932735513423970097 ) ) ;
#19726=CARTESIAN_POINT ( 'NONE',  ( -2.660918448318004614, 118.9023137178985507, -12.46528703574811558 ) ) ;
#19727=CARTESIAN_POINT ( 'NONE',  ( -11.61527771782819940, 140.9351862821014834, 4.622313124798574258 ) ) ;
#19732=CARTESIAN_POINT ( 'NONE',  ( -12.53471296425189152, 6.777313717898553413, -2.311890736173453309 ) ) ;
#19734=CARTESIAN_POINT ( 'NONE',  ( -8.927990412390371944, 109.1273137178985451, -13.04141134922778988 ) ) ;
#19739=CARTESIAN_POINT ( 'NONE',  ( 2.660918448318279950, 116.4976862821014549, -12.46528703574805697 ) ) ;
#19746=CARTESIAN_POINT ( 'NONE',  ( 11.48171059495397728, 119.0851862821014606, 4.944772684328674117 ) ) ;
#19751=CARTESIAN_POINT ( 'NONE',  ( -10.83675517735155047, 96.66018628210144925, -11.08355503943142750 ) ) ;
#19752=CARTESIAN_POINT ( 'NONE',  ( -12.46528703574805874, 22.19768628210144712, -2.660918448318280838 ) ) ;
#19753=CARTESIAN_POINT ( 'NONE',  ( 2.064181346179272847, 134.8976862821014606, -9.465287035748065847 ) ) ;
#19756=ORIENTED_EDGE ( 'NONE', *, *, #32646, .T. ) ;
#19758=CARTESIAN_POINT ( 'NONE',  ( -8.843639120294326972, 58.13518628210145067, 3.474262827703335166 ) ) ;
#19766=CARTESIAN_POINT ( 'NONE',  ( 8.152565276336593669, 48.75231371789854506, 5.233372021372610483 ) ) ;
#19771=CARTESIAN_POINT ( 'NONE',  ( -0.1745138560722763466, 63.98981371789854933, -12.50000000000000355 ) ) ;
#19774=CARTESIAN_POINT ( 'NONE',  ( 6.932735513424201024, 28.05231371789855643, -10.69584247140429412 ) ) ;
#19789=CARTESIAN_POINT ( 'NONE',  ( -13.04141134922778456, 33.22731371789855359, 8.927990412390377273 ) ) ;
#19791=CARTESIAN_POINT ( 'NONE',  ( -6.840914352312096547, 140.3601862821014663, 6.594114490232313663 ) ) ;
#19792=CARTESIAN_POINT ( 'NONE',  ( -4.944772684328673229, 47.78518628210144925, 11.48171059495397728 ) ) ;
#19797=CARTESIAN_POINT ( 'NONE',  ( -8.632099005475501130, 14.14768628210144286, -13.23911966647218996 ) ) ;
#19806=CARTESIAN_POINT ( 'NONE',  ( 6.840914352311949109, 104.2398137178985706, 6.594114490232462877 ) ) ;
#19813=CARTESIAN_POINT ( 'NONE',  ( 7.228626920338837358, 122.9273137178985564, 10.49813415416005036 ) ) ;
#19825=CARTESIAN_POINT ( 'NONE',  ( 12.46528703574805874, 54.39768628210146062, 2.660918448318279950 ) ) ;
#19830=CARTESIAN_POINT ( 'NONE',  ( 11.48171059495408208, 102.5148137178985621, -4.944772684328420986 ) ) ;
#19836=CARTESIAN_POINT ( 'NONE',  ( 15.50000000000000533, 103.0898137178985792, -0.1745138560722452326 ) ) ;
#19839=CARTESIAN_POINT ( 'NONE',  ( -11.61527771782819940, 113.3351862821014606, 4.622313124798574258 ) ) ;
#19840=CARTESIAN_POINT ( 'NONE',  ( 8.632099005475504683, 55.54768628210144499, 13.23911966647218996 ) ) ;
#19843=CARTESIAN_POINT ( 'NONE',  ( 8.927990412390657937, 61.87268628210144783, -13.04141134922759804 ) ) ;
#19846=CARTESIAN_POINT ( 'NONE',  ( -7.954856959092191815, 22.77268628210143220, -5.529263428287477744 ) ) ;
#19850=CARTESIAN_POINT ( 'NONE',  ( 8.715434833791931624, 55.26018628210144357, 8.962234695871760692 ) ) ;
#19853=CARTESIAN_POINT ( 'NONE',  ( -3.796722387233375073, 20.18518628210144783, 8.710071997420127943 ) ) ;
#19864=CARTESIAN_POINT ( 'NONE',  ( -12.46528703574805874, 68.19768628210144357, -2.660918448318280838 ) ) ;
#19869=CARTESIAN_POINT ( 'NONE',  ( 13.23911966647199812, 39.55231371789854933, 8.632099005475788900 ) ) ;
#19877=CARTESIAN_POINT ( 'NONE',  ( 5.529263428287300108, 30.92731371789853867, 7.954856959092309943 ) ) ;
#19882=CARTESIAN_POINT ( 'NONE',  ( -7.228626920338836470, 17.12731371789854862, -10.49813415416005213 ) ) ;
#19883=CARTESIAN_POINT ( 'NONE',  ( 6.932735513423970097, 64.74768628210145494, 10.69584247140445044 ) ) ;
#19885=DIRECTION ( 'NONE',  ( 0.000000000000000000, 1.000000000000000000, 0.000000000000000000 ) ) ;
#19891=CARTESIAN_POINT ( 'NONE',  ( -5.233372021372430183, 78.54768628210145209, -8.152565276336710909 ) ) ;
#19893=CARTESIAN_POINT ( 'NONE',  ( -10.49813415415989581, 114.7726862821014606, -7.228626920339068285 ) ) ;
#19906=CARTESIAN_POINT ( 'NONE',  ( 11.48171059495408208, 120.9148137178985536, -4.944772684328420986 ) ) ;
#19907=CARTESIAN_POINT ( 'NONE',  ( -7.228626920339070061, 130.8726862821014834, 10.49813415415989404 ) ) ;
#19912=CARTESIAN_POINT ( 'NONE',  ( -3.257655550456946880, 100.5023137178985451, -15.46528703574811736 ) ) ;
#19914=CARTESIAN_POINT ( 'NONE',  ( -12.46528703574805697, 95.79768628210143788, -2.660918448318280838 ) ) ;
#19919=CARTESIAN_POINT ( 'NONE',  ( -8.962234695871760692, 121.9601862821014464, 8.715434833791933400 ) ) ;
#19926=CARTESIAN_POINT ( 'NONE',  ( 7.228626920339068285, 117.0726862821014720, -10.49813415415989581 ) ) ;
#19931=CARTESIAN_POINT ( 'NONE',  ( 0.1745138560725837118, 107.0101862821014578, -15.50000000000000533 ) ) ;
#19932=CARTESIAN_POINT ( 'NONE',  ( 8.715434833791931624, 9.260186282101429356, 8.962234695871760692 ) ) ;
#19933=CARTESIAN_POINT ( 'NONE',  ( -3.796722387233375073, 139.7851862821014493, 8.710071997420127943 ) ) ;
#19939=CARTESIAN_POINT ( 'NONE',  ( -8.152565276336710909, 57.84768628210144925, 5.233372021372435512 ) ) ;
#19946=CARTESIAN_POINT ( 'NONE',  ( 2.064181346179061460, 31.50231371789854862, 9.465287035748106703 ) ) ;
#19950=CARTESIAN_POINT ( 'NONE',  ( 4.622313124798831829, 55.36481371789855643, -11.61527771782809282 ) ) ;
#19953=CARTESIAN_POINT ( 'NONE',  ( -15.46528703574811736, 144.2023137178985905, 3.257655550456946436 ) ) ;
#19956=CARTESIAN_POINT ( 'NONE',  ( 0.1745138560725515708, 5.810186282101447830, -12.50000000000000355 ) ) ;
#19967=CARTESIAN_POINT ( 'NONE',  ( -5.770363421894122880, 13.96481371789853831, 14.38691631536194393 ) ) ;
#19969=CARTESIAN_POINT ( 'NONE',  ( -12.50000000000000355, 3.510186282101451560, -0.1745138560725492671 ) ) ;
#19970=CARTESIAN_POINT ( 'NONE',  ( 8.962234695871762469, 52.96018628210144641, -8.715434833791931624 ) ) ;
#19973=CARTESIAN_POINT ( 'NONE',  ( 5.770363421893814682, 19.03518628210144570, 14.38691631536207183 ) ) ;
#19982=CARTESIAN_POINT ( 'NONE',  ( -5.233372021372612259, 97.05231371789855643, 8.152565276336593669 ) ) ;
#19988=CARTESIAN_POINT ( 'NONE',  ( 12.46528703574811558, 112.0023137178985593, -2.660918448318005947 ) ) ;
#20001=CARTESIAN_POINT ( 'NONE',  ( -4.622313124798576922, 60.43518628210145494, -11.61527771782819762 ) ) ;
#20006=CARTESIAN_POINT ( 'NONE',  ( 4.944772684328420986, 104.8148137178985593, 11.48171059495408208 ) ) ;
#20011=CARTESIAN_POINT ( 'NONE',  ( 6.092822981423662299, 68.01481371789854791, 14.25334919248795096 ) ) ;
#20016=CARTESIAN_POINT ( 'NONE',  ( -11.48171059495397373, 96.08518628210146062, -4.944772684328680334 ) ) ;
#20017=CARTESIAN_POINT ( 'NONE',  ( -13.04141134922759804, 68.77268628210143220, -8.927990412390657937 ) ) ;
#20021=CARTESIAN_POINT ( 'NONE',  ( -10.83675517735155047, 59.86018628210145209, -11.08355503943142750 ) ) ;
#20027=CARTESIAN_POINT ( 'NONE',  ( -2.311890736173176641, 42.32268628210145067, -12.53471296425194836 ) ) ;
#20030=CARTESIAN_POINT ( 'NONE',  ( -6.840914352312096547, 29.96018628210143575, 6.594114490232313663 ) ) ;
#20042=CARTESIAN_POINT ( 'NONE',  ( 0.1745138560725515708, 61.01018628210145067, -12.50000000000000355 ) ) ;
#20047=CARTESIAN_POINT ( 'NONE',  ( -2.908627838312453306, 41.27731371789855075, 15.53471296425188797 ) ) ;
#20055=CARTESIAN_POINT ( 'NONE',  ( 7.954856959092311719, 28.62731371789854506, -5.529263428287300108 ) ) ;
#20060=CARTESIAN_POINT ( 'NONE',  ( 11.61527771782809637, 11.66481371789854293, 4.622313124798827388 ) ) ;
#20062=CARTESIAN_POINT ( 'NONE',  ( -4.622313124798576922, 60.43518628210145494, -11.61527771782819762 ) ) ;
#20069=CARTESIAN_POINT ( 'NONE',  ( -6.840914352312096547, 75.96018628210144641, 6.594114490232313663 ) ) ;
#20071=CARTESIAN_POINT ( 'NONE',  ( 12.53471296425194836, 109.0226862821014606, -2.311890736173178418 ) ) ;
#20084=CARTESIAN_POINT ( 'NONE',  ( -10.49813415416004858, 125.2273137178985820, 7.228626920338839135 ) ) ;
#20085=CARTESIAN_POINT ( 'NONE',  ( -10.69584247140444866, 122.2476862821014549, 6.932735513423972762 ) ) ;
#20091=CARTESIAN_POINT ( 'NONE',  ( -3.257655550456946880, 91.30231371789854222, -15.46528703574811736 ) ) ;
#20092=CARTESIAN_POINT ( 'NONE',  ( 0.1745138560725515708, 88.61018628210146630, -12.50000000000000355 ) ) ;
#20095=CARTESIAN_POINT ( 'NONE',  ( -9.465287035748106703, 70.60231371789853938, 2.064181346179061460 ) ) ;
#20099=CARTESIAN_POINT ( 'NONE',  ( 12.53471296425194836, 127.4226862821014663, -2.311890736173178418 ) ) ;
#20105=CARTESIAN_POINT ( 'NONE',  ( 13.04141134922759804, 100.9726862821014635, 8.927990412390657937 ) ) ;
#20106=CARTESIAN_POINT ( 'NONE',  ( 8.962234695871762469, 16.16018628210144570, -8.715434833791931624 ) ) ;
#20109=CARTESIAN_POINT ( 'NONE',  ( -5.233372021372430183, 133.7476862821013981, -8.152565276336710909 ) ) ;
#20113=CARTESIAN_POINT ( 'NONE',  ( -0.1745138560725182642, 56.41018628210145636, 9.500000000000005329 ) ) ;
#20121=CARTESIAN_POINT ( 'NONE',  ( 9.534712964251900402, 29.77731371789854364, 1.715153634034445540 ) ) ;
#20127=CARTESIAN_POINT ( 'NONE',  ( 11.48171059495408208, 47.31481371789855928, -4.944772684328420986 ) ) ;
#20130=CARTESIAN_POINT ( 'NONE',  ( 3.257655550456945548, 141.9023137178985507, 15.46528703574811736 ) ) ;
#20147=CARTESIAN_POINT ( 'NONE',  ( -14.38691631536193860, 25.46481371789855075, -5.770363421894132649 ) ) ;
#20149=CARTESIAN_POINT ( 'NONE',  ( 2.660918448318279950, 15.29768628210143078, -12.46528703574805697 ) ) ;
#20151=CARTESIAN_POINT ( 'NONE',  ( 4.622313124798573369, 55.83518628210144641, 11.61527771782819940 ) ) ;
#20163=CARTESIAN_POINT ( 'NONE',  ( 3.474262827703532341, 92.16481371789855359, -8.843639120294245259 ) ) ;
#20170=CARTESIAN_POINT ( 'NONE',  ( -11.48171059495408208, 97.91481371789856780, 4.944772684328421875 ) ) ;
#20174=CARTESIAN_POINT ( 'NONE',  ( 2.311890736173452865, 73.47731371789856780, -12.53471296425189152 ) ) ;
#20183=CARTESIAN_POINT ( 'NONE',  ( 4.622313124798573369, 55.83518628210144641, 11.61527771782819940 ) ) ;
#20189=CARTESIAN_POINT ( 'NONE',  ( -2.660918448318004614, 109.7023137178985621, -12.46528703574811558 ) ) ;
#20194=CARTESIAN_POINT ( 'NONE',  ( -10.83675517735179028, 78.93981371789855928, 11.08355503943118947 ) ) ;
#20198=CARTESIAN_POINT ( 'NONE',  ( -10.49813415415989581, 105.5726862821014578, -7.228626920339068285 ) ) ;
#20199=CARTESIAN_POINT ( 'NONE',  ( -14.38691631536207183, 48.93518628210144072, 5.770363421893814682 ) ) ;
#20203=CARTESIAN_POINT ( 'NONE',  ( 14.25334919248782661, 73.08518628210143220, 6.092822981423971385 ) ) ;
#20208=CARTESIAN_POINT ( 'NONE',  ( -4.944772684328673229, 38.58518628210144641, 11.48171059495397728 ) ) ;
#20211=CARTESIAN_POINT ( 'NONE',  ( -7.954856959092191815, 4.372686282101438948, -5.529263428287477744 ) ) ;
#20224=CARTESIAN_POINT ( 'NONE',  ( 6.932735513423970097, 64.74768628210145494, 10.69584247140445044 ) ) ;
#20230=CARTESIAN_POINT ( 'NONE',  ( 2.908627838312458636, 45.87731371789854506, -15.53471296425188442 ) ) ;
#20237=CARTESIAN_POINT ( 'NONE',  ( 5.233372021372610483, 28.05231371789855643, -8.152565276336593669 ) ) ;
#20244=CARTESIAN_POINT ( 'NONE',  ( -11.08355503943118592, 136.4398137178985735, -10.83675517735179383 ) ) ;
#20248=CARTESIAN_POINT ( 'NONE',  ( -2.311890736173176641, 51.52268628210145351, -12.53471296425194836 ) ) ;
#20255=CARTESIAN_POINT ( 'NONE',  ( 8.152565276336714462, 71.64768628210146062, -5.233372021372432847 ) ) ;
#20260=CARTESIAN_POINT ( 'NONE',  ( 0.1745138560725515708, 97.81018628210144072, -12.50000000000000355 ) ) ;
#20273=CARTESIAN_POINT ( 'NONE',  ( -6.932735513424201912, 124.6523137178985650, 10.69584247140429412 ) ) ;
#20274=CARTESIAN_POINT ( 'NONE',  ( -12.46528703574805874, 123.3976862821014606, -2.660918448318280838 ) ) ;
#20280=CARTESIAN_POINT ( 'NONE',  ( -0.1745138560722442889, 91.58981371789856496, -15.50000000000000533 ) ) ;
#20284=CARTESIAN_POINT ( 'NONE',  ( -6.594114490232462877, 69.73981371789855643, 6.840914352311949109 ) ) ;
#20287=CARTESIAN_POINT ( 'NONE',  ( -4.944772684328424539, 54.21481371789854364, -11.48171059495408031 ) ) ;
#20290=CARTESIAN_POINT ( 'NONE',  ( -12.53471296425194836, 95.22268628210146346, 2.311890736173176641 ) ) ;
#20295=CARTESIAN_POINT ( 'NONE',  ( -8.927990412390661490, 94.07268628210144357, 13.04141134922759804 ) ) ;
#20296=CARTESIAN_POINT ( 'NONE',  ( 12.46528703574805874, 8.397686282101441080, 2.660918448318279950 ) ) ;
#20300=CARTESIAN_POINT ( 'NONE',  ( 8.843639120294328748, 136.3351862821014606, -3.474262827703334722 ) ) ;
#20301=CARTESIAN_POINT ( 'NONE',  ( 8.843639120294245259, 85.26481371789857633, 3.474262827703527901 ) ) ;
#20305=CARTESIAN_POINT ( 'NONE',  ( 3.796722387233379514, 61.58518628210146062, -8.710071997420127943 ) ) ;
#20313=CARTESIAN_POINT ( 'NONE',  ( -3.796722387233185003, 45.01481371789854791, -8.710071997420207879 ) ) ;
#20318=CARTESIAN_POINT ( 'NONE',  ( 2.311890736173452421, 36.67731371789854933, -12.53471296425189152 ) ) ;
#20321=CARTESIAN_POINT ( 'NONE',  ( 10.49813415416005213, 10.22731371789853227, -7.228626920338837358 ) ) ;
#20339=CARTESIAN_POINT ( 'NONE',  ( -14.25334919248795096, 24.31481371789855217, 6.092822981423662299 ) ) ;
#20341=CARTESIAN_POINT ( 'NONE',  ( -8.152565276336710909, 140.6476862821014322, 5.233372021372435512 ) ) ;
#20342=CARTESIAN_POINT ( 'NONE',  ( -2.311890736173176641, 51.52268628210145351, -12.53471296425194836 ) ) ;
#20354=CARTESIAN_POINT ( 'NONE',  ( -3.796722387233185003, 100.2148137178985650, -8.710071997420207879 ) ) ;
#20361=CARTESIAN_POINT ( 'NONE',  ( 8.715434833792128799, 101.9398137178985593, -8.962234695871567070 ) ) ;
#20365=CARTESIAN_POINT ( 'NONE',  ( 10.49813415416005213, 65.42731371789855643, -7.228626920338837358 ) ) ;
#20373=CARTESIAN_POINT ( 'NONE',  ( -8.715434833791929847, 41.46018628210144641, -8.962234695871762469 ) ) ;
#20380=CARTESIAN_POINT ( 'NONE',  ( 4.622313124798831829, 110.5648137178985593, -11.61527771782809282 ) ) ;
#20386=CARTESIAN_POINT ( 'NONE',  ( -0.1745138560722442889, 82.38981371789856212, -15.50000000000000533 ) ) ;
#20390=CARTESIAN_POINT ( 'NONE',  ( -4.944772684328673229, 112.1851862821014549, 11.48171059495397728 ) ) ;
#20391=CARTESIAN_POINT ( 'NONE',  ( 15.53471296425195369, 53.82268628210144357, -2.908627838312120684 ) ) ;
#20394=CARTESIAN_POINT ( 'NONE',  ( -15.50000000000000533, 67.91018628210144925, -0.1745138560725808530 ) ) ;
#20400=CARTESIAN_POINT ( 'NONE',  ( -2.311890736173176641, 33.12268628210144072, -12.53471296425194836 ) ) ;
#20403=CARTESIAN_POINT ( 'NONE',  ( 6.594114490232313663, 9.260186282101427580, 6.840914352312096547 ) ) ;
#20413=CARTESIAN_POINT ( 'NONE',  ( -10.69584247140444866, 67.04768628210145209, 6.932735513423972762 ) ) ;
#20421=CARTESIAN_POINT ( 'NONE',  ( -5.770363421894122880, 32.36481371789854933, 14.38691631536194393 ) ) ;
#20428=CARTESIAN_POINT ( 'NONE',  ( -8.152565276336593669, 25.75231371789854506, -5.233372021372610483 ) ) ;
#20435=CARTESIAN_POINT ( 'NONE',  ( -15.53471296425188442, 135.5773137178985905, -2.908627838312459080 ) ) ;
#20437=CARTESIAN_POINT ( 'NONE',  ( -4.944772684328673229, 38.58518628210144641, 11.48171059495397728 ) ) ;
#20445=CARTESIAN_POINT ( 'NONE',  ( 6.840914352312096547, 52.96018628210144641, -6.594114490232313663 ) ) ;
#20448=CARTESIAN_POINT ( 'NONE',  ( 7.228626920339068285, 98.67268628210145209, -10.49813415415989581 ) ) ;
#20460=CARTESIAN_POINT ( 'NONE',  ( 11.61527771782809637, 112.8648137178985564, 4.622313124798827388 ) ) ;
#20461=CARTESIAN_POINT ( 'NONE',  ( 10.69584247140445221, 117.6476862821014606, -6.932735513423970097 ) ) ;
#20467=CARTESIAN_POINT ( 'NONE',  ( -14.25334919248795096, 88.71481371789855075, 6.092822981423662299 ) ) ;
#20472=CARTESIAN_POINT ( 'NONE',  ( 8.152565276336593669, 67.15231371789852233, 5.233372021372610483 ) ) ;
#20475=CARTESIAN_POINT ( 'NONE',  ( -2.660918448318004614, 54.50231371789855217, -12.46528703574811558 ) ) ;
#20477=CARTESIAN_POINT ( 'NONE',  ( -11.61527771782819940, 104.1351862821014578, 4.622313124798574258 ) ) ;
#20483=CARTESIAN_POINT ( 'NONE',  ( 14.38691631536207538, 108.7351862821014663, -5.770363421893813793 ) ) ;
#20484=CARTESIAN_POINT ( 'NONE',  ( -7.228626920339070061, 11.27268628210142865, 10.49813415415989404 ) ) ;
#20487=CARTESIAN_POINT ( 'NONE',  ( 0.1745138560725194299, 125.4101862821014635, -9.500000000000005329 ) ) ;
#20493=CARTESIAN_POINT ( 'NONE',  ( -3.796722387233375073, 66.18518628210145494, 8.710071997420127943 ) ) ;
#20501=CARTESIAN_POINT ( 'NONE',  ( 8.843639120294245259, 39.26481371789855501, 3.474262827703527901 ) ) ;
#20507=CARTESIAN_POINT ( 'NONE',  ( 10.69584247140429589, 39.55231371789854933, 6.932735513424201024 ) ) ;
#20510=CARTESIAN_POINT ( 'NONE',  ( -10.49813415416004858, 14.82731371789855501, 7.228626920338839135 ) ) ;
#20525=CARTESIAN_POINT ( 'NONE',  ( -8.927990412390371944, 17.12731371789855217, -13.04141134922778988 ) ) ;
#20527=CARTESIAN_POINT ( 'NONE',  ( -7.954856959092191815, 133.1726862821014663, -5.529263428287477744 ) ) ;
#20528=CARTESIAN_POINT ( 'NONE',  ( 2.660918448318279950, 42.89768628210143930, -12.46528703574805697 ) ) ;
#20533=CARTESIAN_POINT ( 'NONE',  ( 8.710071997420127943, 17.88518628210143646, 3.796722387233375073 ) ) ;
#20540=CARTESIAN_POINT ( 'NONE',  ( -5.233372021372612259, 87.85231371789855359, 8.152565276336593669 ) ) ;
#20545=CARTESIAN_POINT ( 'NONE',  ( -8.962234695871565293, 99.63981371789856212, -8.715434833792128799 ) ) ;
#20549=CARTESIAN_POINT ( 'NONE',  ( -2.660918448318004614, 72.90231371789855075, -12.46528703574811558 ) ) ;
#20557=CARTESIAN_POINT ( 'NONE',  ( 11.61527771782819940, 35.13518628210143646, -4.622313124798573369 ) ) ;
#20563=CARTESIAN_POINT ( 'NONE',  ( -8.962234695871565293, 108.8398137178985507, -8.715434833792128799 ) ) ;
#20568=CARTESIAN_POINT ( 'NONE',  ( 14.25334919248795451, 74.91481371789855359, -6.092822981423661410 ) ) ;
#20572=CARTESIAN_POINT ( 'NONE',  ( 4.944772684328679446, 98.38518628210145778, -11.48171059495397373 ) ) ;
#20573=CARTESIAN_POINT ( 'NONE',  ( -11.08355503943142573, 48.36018628210145209, 10.83675517735155402 ) ) ;
#20576=CARTESIAN_POINT ( 'NONE',  ( 5.770363421893814682, 74.23518628210142367, 14.38691631536207183 ) ) ;
#20582=CARTESIAN_POINT ( 'NONE',  ( -0.1745138560725500443, 47.21018628210143930, 12.50000000000000355 ) ) ;
#20585=CARTESIAN_POINT ( 'NONE',  ( -5.233372021372430183, 4.947686282101431132, -8.152565276336710909 ) ) ;
#20597=EDGE_CURVE ( 'NONE', #15372, #21580, #7395, .T. ) ;
#20598=CARTESIAN_POINT ( 'NONE',  ( 7.228626920339069173, 61.87268628210144783, -10.49813415415989404 ) ) ;
#20606=CARTESIAN_POINT ( 'NONE',  ( 11.08355503943118769, 12.23981371789853512, 10.83675517735179028 ) ) ;
#20613=CARTESIAN_POINT ( 'NONE',  ( 3.474262827703532341, 18.56481371789855928, -8.843639120294245259 ) ) ;
#20619=CARTESIAN_POINT ( 'NONE',  ( 2.908627838312458636, 137.8773137178985735, -15.53471296425188442 ) ) ;
#20622=CARTESIAN_POINT ( 'NONE',  ( -11.61527771782819940, 48.93518628210144783, 4.622313124798574258 ) ) ;
#20630=CARTESIAN_POINT ( 'NONE',  ( 1.715153634034233487, 65.32268628210144357, 9.534712964251941258 ) ) ;
#20633=CARTESIAN_POINT ( 'NONE',  ( -7.228626920339069173, 103.2726862821014606, 10.49813415415989581 ) ) ;
#20644=CARTESIAN_POINT ( 'NONE',  ( -6.932735513424201912, 106.2523137178985735, 10.69584247140429412 ) ) ;
#20645=CARTESIAN_POINT ( 'NONE',  ( -2.311890736173176641, 115.9226862821014521, -12.53471296425194659 ) ) ;
#20651=CARTESIAN_POINT ( 'NONE',  ( 15.46528703574811736, 93.60231371789855359, -3.257655550456947768 ) ) ;
#20654=CARTESIAN_POINT ( 'NONE',  ( 3.474262827703335166, 92.63518628210147199, 8.843639120294326972 ) ) ;
#20656=CARTESIAN_POINT ( 'NONE',  ( -7.954856959092309943, 70.02731371789855075, 5.529263428287300108 ) ) ;
#20659=CARTESIAN_POINT ( 'NONE',  ( 12.46528703574811558, 56.80231371789856354, -2.660918448318005503 ) ) ;
#20662=CARTESIAN_POINT ( 'NONE',  ( 8.715434833791931624, 101.2601862821014578, 8.962234695871760692 ) ) ;
#20665=CARTESIAN_POINT ( 'NONE',  ( 4.622313124798573369, 138.6351862821014720, 11.61527771782819940 ) ) ;
#20667=CARTESIAN_POINT ( 'NONE',  ( -3.257655550457281723, 84.29768628210146630, 15.46528703574804986 ) ) ;
#20670=CARTESIAN_POINT ( 'NONE',  ( -9.500000000000005329, 113.9101862821014493, -0.1745138560725176813 ) ) ;
#20671=CARTESIAN_POINT ( 'NONE',  ( 14.25334919248782661, 8.685186282101437172, 6.092822981423971385 ) ) ;
#20676=CARTESIAN_POINT ( 'NONE',  ( 3.796722387233379514, 52.38518628210145778, -8.710071997420127943 ) ) ;
#20684=CARTESIAN_POINT ( 'NONE',  ( -9.534712964251895073, 34.37731371789854506, -1.715153634034446428 ) ) ;
#20688=CARTESIAN_POINT ( 'NONE',  ( -2.660918448318005058, 45.30231371789855643, -12.46528703574811558 ) ) ;
#20691=CARTESIAN_POINT ( 'NONE',  ( 12.53471296425189330, 11.37731371789854506, 2.311890736173451977 ) ) ;
#20708=CARTESIAN_POINT ( 'NONE',  ( 14.38691631536194393, 30.06481371789855572, 5.770363421894124656 ) ) ;
#20711=CARTESIAN_POINT ( 'NONE',  ( -9.500000000000005329, 123.1101862821014663, -0.1745138560725176813 ) ) ;
#20712=CARTESIAN_POINT ( 'NONE',  ( 12.53471296425194836, 35.42268628210144499, -2.311890736173178418 ) ) ;
#20717=CARTESIAN_POINT ( 'NONE',  ( -3.474262827703337830, 14.43518628210144072, -8.843639120294326972 ) ) ;
#20724=CARTESIAN_POINT ( 'NONE',  ( 8.152565276336593669, 85.55231371789855643, 5.233372021372610483 ) ) ;
#20730=CARTESIAN_POINT ( 'NONE',  ( 8.715434833792128799, 92.73981371789855643, -8.962234695871567070 ) ) ;
#20734=CARTESIAN_POINT ( 'NONE',  ( -12.46528703574811558, 61.40231371789855785, 2.660918448318003726 ) ) ;
#20743=CARTESIAN_POINT ( 'NONE',  ( -8.962234695871760692, 39.16018628210144215, 8.715434833791933400 ) ) ;
#20749=CARTESIAN_POINT ( 'NONE',  ( -10.49813415416004858, 88.42731371789858485, 7.228626920338839135 ) ) ;
#20754=CARTESIAN_POINT ( 'NONE',  ( -13.04141134922778456, 70.02731371789855075, 8.927990412390377273 ) ) ;
#20759=CARTESIAN_POINT ( 'NONE',  ( 10.49813415415989581, 110.1726862821014521, 7.228626920339068285 ) ) ;
#20760=CARTESIAN_POINT ( 'NONE',  ( -13.04141134922759804, 50.37268628210144783, -8.927990412390657937 ) ) ;
#20763=CARTESIAN_POINT ( 'NONE',  ( 2.908627838312118019, 56.12268628210142651, 15.53471296425195369 ) ) ;
#20770=CARTESIAN_POINT ( 'NONE',  ( 10.69584247140445221, 34.84768628210143504, -6.932735513423970097 ) ) ;
#20772=CARTESIAN_POINT ( 'NONE',  ( 2.064181346179272847, 6.097686282101443922, -9.465287035748065847 ) ) ;
#20784=CARTESIAN_POINT ( 'NONE',  ( 12.46528703574805874, 54.39768628210145351, 2.660918448318279950 ) ) ;
#20791=CARTESIAN_POINT ( 'NONE',  ( -12.53471296425194836, 104.4226862821014379, 2.311890736173176641 ) ) ;
#20792=CARTESIAN_POINT ( 'NONE',  ( 10.83675517735179206, 28.33981371789855430, -11.08355503943118769 ) ) ;
#20800=CARTESIAN_POINT ( 'NONE',  ( 3.796722387233182339, 12.81481371789855217, 8.710071997420207879 ) ) ;
#20807=CARTESIAN_POINT ( 'NONE',  ( -5.770363421894122880, 124.3648137178985849, 14.38691631536194393 ) ) ;
#20811=CARTESIAN_POINT ( 'NONE',  ( 2.660918448318279950, 42.89768628210143930, -12.46528703574805697 ) ) ;
#20818=CARTESIAN_POINT ( 'NONE',  ( -8.710071997420127943, 59.28518628210144925, -3.796722387233380402 ) ) ;
#20822=CARTESIAN_POINT ( 'NONE',  ( -0.1745138560725500443, 102.4101862821014493, 12.50000000000000355 ) ) ;
#20834=CARTESIAN_POINT ( 'NONE',  ( -8.715434833792127023, 97.33981371789855075, 8.962234695871568846 ) ) ;
#20835=CARTESIAN_POINT ( 'NONE',  ( 0.1745138560725515708, 97.81018628210144072, -12.50000000000000355 ) ) ;
#20840=CARTESIAN_POINT ( 'NONE',  ( -13.23911966647199812, 71.75231371789854506, -8.632099005475788900 ) ) ;
#20843=CARTESIAN_POINT ( 'NONE',  ( -7.954856959092191815, 105.5726862821014294, -5.529263428287477744 ) ) ;
#20847=CARTESIAN_POINT ( 'NONE',  ( 7.954856959092311719, 74.62731371789853085, -5.529263428287300108 ) ) ;
#20851=CARTESIAN_POINT ( 'NONE',  ( 10.69584247140429589, 48.75231371789854506, 6.932735513424201024 ) ) ;
#20854=CARTESIAN_POINT ( 'NONE',  ( 2.660918448318279950, 107.2976862821014521, -12.46528703574805697 ) ) ;
#20858=CARTESIAN_POINT ( 'NONE',  ( 2.311890736173175753, 138.9226862821014663, 12.53471296425194836 ) ) ;
#20860=CARTESIAN_POINT ( 'NONE',  ( 0.1745138560725837118, 88.61018628210146630, -15.50000000000000533 ) ) ;
#20865=CARTESIAN_POINT ( 'NONE',  ( 3.796722387233379514, 116.7851862821014635, -8.710071997420127943 ) ) ;
#20867=CARTESIAN_POINT ( 'NONE',  ( 15.53471296425195369, 7.822686282101448896, -2.908627838312120684 ) ) ;
#20870=ORIENTED_EDGE ( 'NONE', *, *, #25320, .F. ) ;
#20878=CARTESIAN_POINT ( 'NONE',  ( 1.715153634034445762, 27.47731371789854649, -9.534712964251895073 ) ) ;
#20882=CARTESIAN_POINT ( 'NONE',  ( -11.48171059495408208, 42.71481371789855075, 4.944772684328421875 ) ) ;
#20884=CARTESIAN_POINT ( 'NONE',  ( -5.770363421894122880, 133.5648137178985735, 14.38691631536194393 ) ) ;
#20900=CARTESIAN_POINT ( 'NONE',  ( -3.257655550457281723, 139.4976862821014549, 15.46528703574804986 ) ) ;
#20902=CARTESIAN_POINT ( 'NONE',  ( 8.710071997420127943, 137.4851862821014379, 3.796722387233375073 ) ) ;
#20905=CARTESIAN_POINT ( 'NONE',  ( 6.932735513423970097, 27.94768628210143646, 10.69584247140445044 ) ) ;
#20910=CARTESIAN_POINT ( 'NONE',  ( -0.1745138560725817967, 120.8101862821014691, 15.50000000000000533 ) ) ;
#20912=CARTESIAN_POINT ( 'NONE',  ( -5.529263428287477744, 11.27268628210142865, 7.954856959092191815 ) ) ;
#20919=CARTESIAN_POINT ( 'NONE',  ( -2.064181346179062349, 82.10231371789853938, -9.465287035748106703 ) ) ;
#20923=CARTESIAN_POINT ( 'NONE',  ( -8.962234695871565293, 90.43981371789855928, -8.715434833792128799 ) ) ;
#20927=CARTESIAN_POINT ( 'NONE',  ( -6.932735513424201912, 60.25231371789855217, 10.69584247140429412 ) ) ;
#20938=CARTESIAN_POINT ( 'NONE',  ( -11.61527771782819940, 48.93518628210144783, 4.622313124798574258 ) ) ;
#20944=CARTESIAN_POINT ( 'NONE',  ( -7.228626920338836470, 81.52731371789855075, -10.49813415416005213 ) ) ;
#20949=CARTESIAN_POINT ( 'NONE',  ( 6.092822981423662299, 58.81481371789855217, 14.25334919248795096 ) ) ;
#20952=CARTESIAN_POINT ( 'NONE',  ( -12.50000000000000355, 77.11018628210145209, -0.1745138560725492671 ) ) ;
#20953=CARTESIAN_POINT ( 'NONE',  ( -14.38691631536207183, 39.73518628210145209, 5.770363421893814682 ) ) ;
#20958=CARTESIAN_POINT ( 'NONE',  ( 8.632099005475504683, 55.54768628210144499, 13.23911966647218996 ) ) ;
#20964=CARTESIAN_POINT ( 'NONE',  ( -8.962234695871760692, 29.96018628210143930, 8.715434833791933400 ) ) ;
#20966=CARTESIAN_POINT ( 'NONE',  ( 8.152565276336593669, 140.7523137178985166, 5.233372021372610483 ) ) ;
#20977=CARTESIAN_POINT ( 'NONE',  ( -12.46528703574805874, 40.59768628210144925, -2.660918448318280838 ) ) ;
#20985=CARTESIAN_POINT ( 'NONE',  ( 11.48171059495397728, 100.6851862821014691, 4.944772684328674117 ) ) ;
#20986=CARTESIAN_POINT ( 'NONE',  ( 15.46528703574811736, 29.20231371789855501, -3.257655550456947768 ) ) ;
#20992=CARTESIAN_POINT ( 'NONE',  ( 12.53471296425189330, 140.1773137178985849, 2.311890736173451977 ) ) ;
#20998=CARTESIAN_POINT ( 'NONE',  ( -0.1745138560722442889, 119.1898137178985593, -15.50000000000000533 ) ) ;
#21003=CARTESIAN_POINT ( 'NONE',  ( -7.228626920339069173, 38.87268628210144072, 10.49813415415989581 ) ) ;
#21007=CARTESIAN_POINT ( 'NONE',  ( 15.46528703574804986, 109.5976862821014493, 3.257655550457285720 ) ) ;
#21010=CARTESIAN_POINT ( 'NONE',  ( -0.1745138560725182642, 56.41018628210145636, 9.500000000000005329 ) ) ;
#21013=CARTESIAN_POINT ( 'NONE',  ( 8.715434833791931624, 82.86018628210145209, 8.962234695871760692 ) ) ;
#21026=CARTESIAN_POINT ( 'NONE',  ( 12.50000000000000355, 112.2898137178985678, -0.1745138560722771515 ) ) ;
#21027=CARTESIAN_POINT ( 'NONE',  ( -11.61527771782819940, 104.1351862821014578, 4.622313124798574258 ) ) ;
#21031=CARTESIAN_POINT ( 'NONE',  ( 8.927990412390371944, 67.72731371789853938, 13.04141134922778811 ) ) ;
#21034=CARTESIAN_POINT ( 'NONE',  ( -3.474262827703337830, 106.4351862821014691, -8.843639120294326972 ) ) ;
#21037=CARTESIAN_POINT ( 'NONE',  ( 5.529263428287300108, 58.52731371789855785, 7.954856959092309943 ) ) ;
#21039=CARTESIAN_POINT ( 'NONE',  ( -3.796722387233185003, 109.4148137178985536, -8.710071997420207879 ) ) ;
#21041=CARTESIAN_POINT ( 'NONE',  ( -4.622313124798826500, 50.76481371789855501, 11.61527771782809637 ) ) ;
#21043=CARTESIAN_POINT ( 'NONE',  ( 12.50000000000000355, 109.3101862821014549, 0.1745138560725507937 ) ) ;
#21046=CARTESIAN_POINT ( 'NONE',  ( -8.715434833791929847, 133.4601862821014606, -8.962234695871762469 ) ) ;
#21048=CARTESIAN_POINT ( 'NONE',  ( -15.53471296425195369, 86.02268628210144641, 2.908627838312118019 ) ) ;
#21054=CARTESIAN_POINT ( 'NONE',  ( -2.064181346179269738, 121.0976862821014635, 9.465287035748067623 ) ) ;
#21056=CARTESIAN_POINT ( 'NONE',  ( -8.632099005475501130, 4.947686282101431132, -13.23911966647218996 ) ) ;
#21068=CARTESIAN_POINT ( 'NONE',  ( 9.465287035748106703, 20.00231371789855217, -2.064181346179063237 ) ) ;
#21073=CARTESIAN_POINT ( 'NONE',  ( 8.715434833792128799, 19.13981371789855146, -8.962234695871567070 ) ) ;
#21076=CARTESIAN_POINT ( 'NONE',  ( 5.770363421894130873, 138.1648137178985678, -14.38691631536193860 ) ) ;
#21092=CARTESIAN_POINT ( 'NONE',  ( -15.53471296425195369, 141.2226862821014493, 2.908627838312118019 ) ) ;
#21094=CARTESIAN_POINT ( 'NONE',  ( -3.474262827703337830, 124.8351862821014748, -8.843639120294326972 ) ) ;
#21096=CARTESIAN_POINT ( 'NONE',  ( 4.944772684328679446, 24.78518628210143859, -11.48171059495397373 ) ) ;
#21098=CLOSED_SHELL ( 'NONE', ( #14013, #12372, #28018, #2231, #11259 ) ) ;
#21102=CARTESIAN_POINT ( 'NONE',  ( -6.092822981423970496, 121.3851862821014578, 14.25334919248782661 ) ) ;
#21104=CARTESIAN_POINT ( 'NONE',  ( 8.152565276336714462, 7.247686282101430066, -5.233372021372432847 ) ) ;
#21110=CARTESIAN_POINT ( 'NONE',  ( 3.796722387233182339, 68.01481371789854791, 8.710071997420207879 ) ) ;
#21114=CARTESIAN_POINT ( 'NONE',  ( 10.69584247140429589, 85.55231371789857064, 6.932735513424201024 ) ) ;
#21118=CARTESIAN_POINT ( 'NONE',  ( -12.50000000000000355, 43.28981371789855359, 0.1745138560722786503 ) ) ;
#21124=CARTESIAN_POINT ( 'NONE',  ( 11.61527771782819940, 44.33518628210145351, -4.622313124798573369 ) ) ;
#21130=CARTESIAN_POINT ( 'NONE',  ( -8.962234695871565293, 90.43981371789855928, -8.715434833792128799 ) ) ;
#21136=CARTESIAN_POINT ( 'NONE',  ( -13.23911966647199812, 53.35231371789856780, -8.632099005475788900 ) ) ;
#21139=CARTESIAN_POINT ( 'NONE',  ( 4.622313124798573369, 92.63518628210145778, 11.61527771782819940 ) ) ;
#21140=CARTESIAN_POINT ( 'NONE',  ( -0.1745138560725817967, 28.81018628210143717, 15.50000000000000533 ) ) ;
#21143=CARTESIAN_POINT ( 'NONE',  ( 14.38691631536207538, 53.53518628210145636, -5.770363421893813793 ) ) ;
#21149=CARTESIAN_POINT ( 'NONE',  ( -11.48171059495397373, 13.28518628210142971, -4.944772684328680334 ) ) ;
#21152=CARTESIAN_POINT ( 'NONE',  ( 8.843639120294245259, 131.2648137178985621, 3.474262827703527901 ) ) ;
#21162=CARTESIAN_POINT ( 'NONE',  ( 12.50000000000000355, 44.91018628210144215, 0.1745138560725507937 ) ) ;
#21170=CARTESIAN_POINT ( 'NONE',  ( 4.622313124798573369, 92.63518628210145778, 11.61527771782819940 ) ) ;
#21171=CARTESIAN_POINT ( 'NONE',  ( 2.908627838312458636, 18.27731371789853299, -15.53471296425188442 ) ) ;
#21172=MANIFOLD_SOLID_BREP ( 'Cavity1', #21098 ) ;
#21178=CARTESIAN_POINT ( 'NONE',  ( -12.50000000000000355, 135.2898137178985678, 0.1745138560722786503 ) ) ;
#21185=CARTESIAN_POINT ( 'NONE',  ( 2.908627838312458636, 110.2773137178985650, -15.53471296425188442 ) ) ;
#21188=CARTESIAN_POINT ( 'NONE',  ( -12.53471296425194836, 21.62268628210144072, 2.311890736173176641 ) ) ;
#21193=CARTESIAN_POINT ( 'NONE',  ( 15.46528703574804986, 100.3976862821014606, 3.257655550457285720 ) ) ;
#21197=CARTESIAN_POINT ( 'NONE',  ( -8.152565276336710909, 67.04768628210143788, 5.233372021372435512 ) ) ;
#21201=CARTESIAN_POINT ( 'NONE',  ( 10.69584247140445221, 80.84768628210144925, -6.932735513423970097 ) ) ;
#21213=CARTESIAN_POINT ( 'NONE',  ( -11.61527771782809282, 99.06481371789855928, -4.622313124798832717 ) ) ;
#21214=CARTESIAN_POINT ( 'NONE',  ( 0.1745138560725515708, 107.0101862821014578, -12.50000000000000355 ) ) ;
#21220=CARTESIAN_POINT ( 'NONE',  ( 14.25334919248795451, 74.91481371789855359, -6.092822981423661410 ) ) ;
#21223=CARTESIAN_POINT ( 'NONE',  ( 8.843639120294328748, 99.53518628210146346, -3.474262827703334722 ) ) ;
#21225=CARTESIAN_POINT ( 'NONE',  ( 5.233372021372610483, 55.65231371789855785, -8.152565276336593669 ) ) ;
#21227=CARTESIAN_POINT ( 'NONE',  ( 0.1745138560723095977, 114.5898137178985650, 9.500000000000005329 ) ) ;
#21229=CARTESIAN_POINT ( 'NONE',  ( 12.46528703574811558, 29.20231371789855501, -2.660918448318005503 ) ) ;
#21233=CARTESIAN_POINT ( 'NONE',  ( -2.660918448318275509, 84.29768628210145209, 12.46528703574805874 ) ) ;
#21237=CARTESIAN_POINT ( 'NONE',  ( 15.53471296425195369, 90.62268628210145494, -2.908627838312120684 ) ) ;
#21242=CARTESIAN_POINT ( 'NONE',  ( -6.594114490232312775, 115.0601862821014691, -6.840914352312096547 ) ) ;
#21244=CARTESIAN_POINT ( 'NONE',  ( 12.50000000000000355, 127.7101862821014606, 0.1745138560725507937 ) ) ;
#21253=CARTESIAN_POINT ( 'NONE',  ( -12.50000000000000355, 5.000000000000004441, -1.353084311261909534E-13 ) ) ;
#21256=CARTESIAN_POINT ( 'NONE',  ( -9.500000000000005329, 24.88981371789854080, 0.1745138560723101806 ) ) ;
#21258=EDGE_LOOP ( 'NONE', ( #8182, #20870, #23067 ) ) ;
#21261=CARTESIAN_POINT ( 'NONE',  ( 2.311890736173452421, 18.27731371789853654, -12.53471296425189152 ) ) ;
#21263=CARTESIAN_POINT ( 'NONE',  ( 15.46528703574811736, 130.4023137178985792, -3.257655550456947768 ) ) ;
#21270=CARTESIAN_POINT ( 'NONE',  ( 12.53471296425194836, 136.6226862821014834, -2.311890736173178418 ) ) ;
#21275=( NAMED_UNIT ( * ) PLANE_ANGLE_UNIT ( ) SI_UNIT ( $, .RADIAN. ) );
#21282=CARTESIAN_POINT ( 'NONE',  ( -14.38691631536207183, 140.9351862821014549, 5.770363421893814682 ) ) ;
#21284=CARTESIAN_POINT ( 'NONE',  ( -8.152565276336710909, 122.2476862821014691, 5.233372021372435512 ) ) ;
#21287=CARTESIAN_POINT ( 'NONE',  ( 4.944772684328679446, 33.98518628210143788, -11.48171059495397373 ) ) ;
#21291=CARTESIAN_POINT ( 'NONE',  ( -8.927990412390661490, 130.8726862821014834, 13.04141134922759804 ) ) ;
#21293=CARTESIAN_POINT ( 'NONE',  ( 1.715153634034445762, 137.8773137178985735, -9.534712964251895073 ) ) ;
#21300=CARTESIAN_POINT ( 'NONE',  ( 1.715153634034445762, 82.67731371789852801, -9.534712964251895073 ) ) ;
#21304=CARTESIAN_POINT ( 'NONE',  ( 8.715434833792128799, 83.53981371789856780, -8.962234695871567070 ) ) ;
#21306=CARTESIAN_POINT ( 'NONE',  ( -6.996070402016868250, 143.0000000000000000, 10.82654737139870882 ) ) ;
#21308=CARTESIAN_POINT ( 'NONE',  ( 11.61527771782809637, 39.26481371789855501, 4.622313124798827388 ) ) ;
#21312=CARTESIAN_POINT ( 'NONE',  ( -10.69584247140444866, 21.04768628210144854, 6.932735513423972762 ) ) ;
#21317=CARTESIAN_POINT ( 'NONE',  ( 12.46528703574811558, 84.40231371789853654, -2.660918448318005503 ) ) ;
#21323=CARTESIAN_POINT ( 'NONE',  ( -3.257655550456946880, 54.50231371789855928, -15.46528703574811736 ) ) ;
#21327=CARTESIAN_POINT ( 'NONE',  ( -2.660918448318275509, 84.29768628210145209, 12.46528703574805874 ) ) ;
#21329=CARTESIAN_POINT ( 'NONE',  ( 11.08355503943142750, 34.56018628210144783, -10.83675517735155225 ) ) ;
#21333=CARTESIAN_POINT ( 'NONE',  ( 6.092822981423978490, 43.18518628210144072, -14.25334919248782306 ) ) ;
#21339=CARTESIAN_POINT ( 'NONE',  ( -0.1745138560725500443, 19.61018628210144144, 12.50000000000000355 ) ) ;
#21341=CARTESIAN_POINT ( 'NONE',  ( -5.529263428287297444, 136.7273137178985110, -7.954856959092311719 ) ) ;
#21346=CARTESIAN_POINT ( 'NONE',  ( -2.660918448318005058, 137.3023137178985564, -12.46528703574811558 ) ) ;
#21350=CARTESIAN_POINT ( 'NONE',  ( 12.50000000000000355, 54.11018628210144499, 0.1745138560725507937 ) ) ;
#21358=CARTESIAN_POINT ( 'NONE',  ( -7.228626920339069173, 75.67268628210146630, 10.49813415415989581 ) ) ;
#21359=CARTESIAN_POINT ( 'NONE',  ( -15.53471296425188442, 15.97731371789853405, -2.908627838312459080 ) ) ;
#21366=CARTESIAN_POINT ( 'NONE',  ( -2.660918448318004614, 137.3023137178985564, -12.46528703574811558 ) ) ;
#21372=CARTESIAN_POINT ( 'NONE',  ( 15.46528703574811736, 112.0023137178985451, -3.257655550456947768 ) ) ;
#21375=CARTESIAN_POINT ( 'NONE',  ( 12.46528703574805874, 35.99768628210144072, 2.660918448318279950 ) ) ;
#21380=CARTESIAN_POINT ( 'NONE',  ( -15.46528703574804986, 104.9976862821014549, -3.257655550457287497 ) ) ;
#21383=CARTESIAN_POINT ( 'NONE',  ( -1.715153634034234598, 42.32268628210145067, -9.534712964251941258 ) ) ;
#21387=CARTESIAN_POINT ( 'NONE',  ( 4.622313124798573369, 74.23518628210145209, 11.61527771782819940 ) ) ;
#21390=CARTESIAN_POINT ( 'NONE',  ( -6.840914352312096547, 39.16018628210144215, 6.594114490232313663 ) ) ;
#21399=CARTESIAN_POINT ( 'NONE',  ( 7.228626920338837358, 95.32731371789856212, 10.49813415416005036 ) ) ;
#21400=CARTESIAN_POINT ( 'NONE',  ( -0.1745138560725500443, 111.6101862821014521, 12.50000000000000355 ) ) ;
#21405=CARTESIAN_POINT ( 'NONE',  ( -15.50000000000000533, 80.08981371789856496, 0.1745138560722471477 ) ) ;
#21409=CARTESIAN_POINT ( 'NONE',  ( 9.500000000000005329, 100.1101862821014521, 0.1745138560725188748 ) ) ;
#21411=CARTESIAN_POINT ( 'NONE',  ( -3.796722387233185003, 54.21481371789855785, -8.710071997420207879 ) ) ;
#21413=CARTESIAN_POINT ( 'NONE',  ( 8.843639120294245259, 112.8648137178985564, 3.474262827703527901 ) ) ;
#21415=CARTESIAN_POINT ( 'NONE',  ( 4.944772684328420986, 22.01481371789855501, 11.48171059495408208 ) ) ;
#21417=CARTESIAN_POINT ( 'NONE',  ( 11.48171059495397728, 91.48518628210145209, 4.944772684328674117 ) ) ;
#21426=CARTESIAN_POINT ( 'NONE',  ( 8.152565276336714462, 117.6476862821014322, -5.233372021372432847 ) ) ;
#21429=CARTESIAN_POINT ( 'NONE',  ( -10.49813415415989581, 123.9726862821014493, -7.228626920339068285 ) ) ;
#21441=CARTESIAN_POINT ( 'NONE',  ( -7.954856959092309943, 14.82731371789855324, 5.529263428287300108 ) ) ;
#21448=CARTESIAN_POINT ( 'NONE',  ( -2.311890736173447980, 22.87731371789854151, 12.53471296425189330 ) ) ;
#21450=CARTESIAN_POINT ( 'NONE',  ( 3.257655550456945548, 132.7023137178985337, 15.46528703574811736 ) ) ;
#21458=CARTESIAN_POINT ( 'NONE',  ( -4.622313124798576922, 124.8351862821014748, -11.61527771782819762 ) ) ;
#21466=CARTESIAN_POINT ( 'NONE',  ( 4.622313124798573369, 138.6351862821014720, 11.61527771782819940 ) ) ;
#21470=CARTESIAN_POINT ( 'NONE',  ( 15.50000000000000533, 11.08981371789854897, -0.1745138560722452326 ) ) ;
#21474=CARTESIAN_POINT ( 'NONE',  ( 9.500000000000005329, 109.3101862821014549, 0.1745138560725188748 ) ) ;
#21476=CARTESIAN_POINT ( 'NONE',  ( 12.46528703574805874, 26.79768628210144144, 2.660918448318279950 ) ) ;
#21480=CARTESIAN_POINT ( 'NONE',  ( -10.83675517735155047, 115.0601862821014691, -11.08355503943142750 ) ) ;
#21482=CARTESIAN_POINT ( 'NONE',  ( 9.534712964251941258, 7.822686282101448896, -1.715153634034235708 ) ) ;
#21490=CARTESIAN_POINT ( 'NONE',  ( -2.064181346179062349, 72.90231371789855075, -9.465287035748106703 ) ) ;
#21493=CARTESIAN_POINT ( 'NONE',  ( 2.660918448318003282, 77.50231371789855928, 12.46528703574811558 ) ) ;
#21497=CARTESIAN_POINT ( 'NONE',  ( -11.48171059495408208, 51.91481371789855359, 4.944772684328421875 ) ) ;
#21501=CARTESIAN_POINT ( 'NONE',  ( -12.53471296425194836, 21.62268628210144072, 2.311890736173176641 ) ) ;
#21506=CARTESIAN_POINT ( 'NONE',  ( -11.48171059495408208, 88.71481371789855075, 4.944772684328421875 ) ) ;
#21511=CARTESIAN_POINT ( 'NONE',  ( 14.25334919248795451, 65.71481371789855075, -6.092822981423661410 ) ) ;
#21514=CARTESIAN_POINT ( 'NONE',  ( 12.46528703574805874, 91.19768628210145778, 2.660918448318279950 ) ) ;
#21515=CARTESIAN_POINT ( 'NONE',  ( -8.632099005475501130, 23.34768628210144570, -13.23911966647218996 ) ) ;
#21519=CARTESIAN_POINT ( 'NONE',  ( -13.04141134922759804, 41.17268628210143078, -8.927990412390657937 ) ) ;
#21525=CARTESIAN_POINT ( 'NONE',  ( -10.49813415415989581, 22.77268628210143575, -7.228626920339068285 ) ) ;
#21528=CARTESIAN_POINT ( 'NONE',  ( -9.465287035748106703, 135.0023137178985166, 2.064181346179061460 ) ) ;
#21532=CARTESIAN_POINT ( 'NONE',  ( 10.49813415416005213, 139.0273137178985507, -7.228626920338837358 ) ) ;
#21539=CARTESIAN_POINT ( 'NONE',  ( 8.962234695871762469, 43.76018628210144357, -8.715434833791931624 ) ) ;
#21546=CARTESIAN_POINT ( 'NONE',  ( -11.61527771782819940, 85.73518628210143788, 4.622313124798574258 ) ) ;
#21547=CARTESIAN_POINT ( 'NONE',  ( 2.908627838312118019, 138.9226862821014663, 15.53471296425195369 ) ) ;
#21553=CARTESIAN_POINT ( 'NONE',  ( -10.49813415416004858, 134.4273137178985849, 7.228626920338839135 ) ) ;
#21560=CARTESIAN_POINT ( 'NONE',  ( 6.092822981423662299, 114.0148137178985763, 14.25334919248795096 ) ) ;
#21563=CARTESIAN_POINT ( 'NONE',  ( 7.228626920339068285, 34.27268628210144641, -10.49813415415989581 ) ) ;
#21567=CARTESIAN_POINT ( 'NONE',  ( -13.23911966647218463, 103.8476862821014493, 8.632099005475506459 ) ) ;
#21570=CARTESIAN_POINT ( 'NONE',  ( -6.840914352312096547, 39.16018628210144215, 6.594114490232313663 ) ) ;
#21574=CARTESIAN_POINT ( 'NONE',  ( 7.228626920339068285, 71.07268628210144357, -10.49813415415989581 ) ) ;
#21577=CARTESIAN_POINT ( 'NONE',  ( 8.843639120294328748, 44.33518628210144641, -3.474262827703334722 ) ) ;
#21580=VERTEX_POINT ( 'NONE', #33769 ) ;
#21588=CARTESIAN_POINT ( 'NONE',  ( -4.622313124798826500, 78.36481371789855643, 11.61527771782809637 ) ) ;
#21589=CARTESIAN_POINT ( 'NONE',  ( -7.228626920339070061, 103.2726862821014606, 10.49813415415989404 ) ) ;
#21593=CARTESIAN_POINT ( 'NONE',  ( -2.908627838312453306, 78.07731371789854791, 15.53471296425188797 ) ) ;
#21599=CARTESIAN_POINT ( 'NONE',  ( 3.796722387233182339, 49.61481371789856354, 8.710071997420207879 ) ) ;
#21601=CARTESIAN_POINT ( 'NONE',  ( 9.465287035748106703, 121.2023137178985479, -2.064181346179063237 ) ) ;
#21603=CARTESIAN_POINT ( 'NONE',  ( 11.61527771782809637, 39.26481371789855501, 4.622313124798827388 ) ) ;
#21604=CARTESIAN_POINT ( 'NONE',  ( 12.46528703574805874, 91.19768628210145778, 2.660918448318279950 ) ) ;
#21611=CARTESIAN_POINT ( 'NONE',  ( 2.064181346179272847, 98.09768628210146346, -9.465287035748065847 ) ) ;
#21613=CARTESIAN_POINT ( 'NONE',  ( -10.69584247140444866, 131.4476862821014436, 6.932735513423972762 ) ) ;
#21615=VERTEX_POINT ( 'NONE', #10639 ) ;
#21625=CARTESIAN_POINT ( 'NONE',  ( 9.534712964251900402, 11.37731371789854506, 1.715153634034445540 ) ) ;
#21630=CARTESIAN_POINT ( 'NONE',  ( 10.49813415416005213, 28.62731371789854862, -7.228626920338837358 ) ) ;
#21632=CARTESIAN_POINT ( 'NONE',  ( -10.83675517735179028, 124.9398137178985451, 11.08355503943118947 ) ) ;
#21638=CARTESIAN_POINT ( 'NONE',  ( 11.48171059495397728, 128.2851862821014493, 4.944772684328674117 ) ) ;
#21649=CARTESIAN_POINT ( 'NONE',  ( 10.83675517735155225, 128.8601862821014663, 11.08355503943142573 ) ) ;
#21651=CARTESIAN_POINT ( 'NONE',  ( 2.064181346179272847, 116.4976862821014549, -9.465287035748065847 ) ) ;
#21653=CARTESIAN_POINT ( 'NONE',  ( 0.1745138560725515708, 15.01018628210143468, -12.50000000000000355 ) ) ;
#21658=CARTESIAN_POINT ( 'NONE',  ( 0.1745138560725194299, 88.61018628210146630, -9.500000000000005329 ) ) ;
#21660=CARTESIAN_POINT ( 'NONE',  ( -9.534712964251895073, 135.5773137178985905, -1.715153634034446428 ) ) ;
#21666=CARTESIAN_POINT ( 'NONE',  ( -8.843639120294245259, 71.46481371789856496, -3.474262827703533230 ) ) ;
#21669=CARTESIAN_POINT ( 'NONE',  ( -10.69584247140429412, 80.95231371789856212, -6.932735513424201024 ) ) ;
#21671=CARTESIAN_POINT ( 'NONE',  ( -10.73304900139428675, 142.9999999999998010, 8.431259175847527487 ) ) ;
#21673=CARTESIAN_POINT ( 'NONE',  ( 4.622313124798831829, 46.16481371789854649, -11.61527771782809282 ) ) ;
#21679=CARTESIAN_POINT ( 'NONE',  ( 4.944772684328679446, 24.78518628210143859, -11.48171059495397373 ) ) ;
#21685=CARTESIAN_POINT ( 'NONE',  ( -12.53471296425189152, 71.17731371789855643, -2.311890736173453753 ) ) ;
#21691=CARTESIAN_POINT ( 'NONE',  ( 5.770363421894130873, 55.36481371789856354, -14.38691631536193860 ) ) ;
#21694=CARTESIAN_POINT ( 'NONE',  ( 12.53471296425194836, 63.02268628210145351, -2.311890736173178418 ) ) ;
#21695=CARTESIAN_POINT ( 'NONE',  ( 15.46528703574804986, 35.99768628210143362, 3.257655550457285720 ) ) ;
#21701=CARTESIAN_POINT ( 'NONE',  ( 3.257655550457285720, 24.49768628210144072, -15.46528703574804986 ) ) ;
#21707=CARTESIAN_POINT ( 'NONE',  ( 11.48171059495397728, 17.88518628210143646, 4.944772684328674117 ) ) ;
#21709=CARTESIAN_POINT ( 'NONE',  ( -3.796722387233185003, 127.8148137178985735, -8.710071997420207879 ) ) ;
#21714=CARTESIAN_POINT ( 'NONE',  ( 2.660918448318003282, 132.7023137178985621, 12.46528703574811558 ) ) ;
#21720=CARTESIAN_POINT ( 'NONE',  ( 8.962234695871762469, 25.36018628210144499, -8.715434833791931624 ) ) ;
#21729=CARTESIAN_POINT ( 'NONE',  ( -2.311890736173176641, 79.12268628210145494, -12.53471296425194836 ) ) ;
#21730=CARTESIAN_POINT ( 'NONE',  ( 3.257655550457285720, 134.8976862821014606, -15.46528703574804986 ) ) ;
#21736=CARTESIAN_POINT ( 'NONE',  ( -10.49813415416004858, 143.6273137178986019, 7.228626920338839135 ) ) ;
#21743=CARTESIAN_POINT ( 'NONE',  ( 2.908627838312458636, 119.4773137178985678, -15.53471296425188442 ) ) ;
#21750=CARTESIAN_POINT ( 'NONE',  ( -14.25334919248782306, 96.08518628210146062, -6.092822981423979378 ) ) ;
#21754=CARTESIAN_POINT ( 'NONE',  ( -3.796722387233375073, 38.58518628210143930, 8.710071997420127943 ) ) ;
#21759=CARTESIAN_POINT ( 'NONE',  ( -4.622313124798576922, 69.63518628210145778, -11.61527771782819762 ) ) ;
#21762=CARTESIAN_POINT ( 'NONE',  ( -5.529263428287477744, 38.87268628210144072, 7.954856959092191815 ) ) ;
#21772=CARTESIAN_POINT ( 'NONE',  ( 7.228626920338837358, 86.12731371789855928, 10.49813415416005036 ) ) ;
#21773=CARTESIAN_POINT ( 'NONE',  ( 4.944772684328679446, 79.98518628210145209, -11.48171059495397373 ) ) ;
#21778=CARTESIAN_POINT ( 'NONE',  ( 0.1745138560722461762, 59.38981371789856212, 15.50000000000000533 ) ) ;
#21783=CARTESIAN_POINT ( 'NONE',  ( -6.594114490232462877, 60.53981371789856070, 6.840914352311949109 ) ) ;
#21785=CARTESIAN_POINT ( 'NONE',  ( 8.843639120294245259, 122.0648137178985877, 3.474262827703527901 ) ) ;
#21787=CARTESIAN_POINT ( 'NONE',  ( -6.932735513424201912, 32.65231371789854364, 10.69584247140429412 ) ) ;
#21789=CARTESIAN_POINT ( 'NONE',  ( 4.944772684328679446, 89.18518628210145494, -11.48171059495397373 ) ) ;
#21797=CARTESIAN_POINT ( 'NONE',  ( -3.474262827703337830, 97.23518628210146630, -8.843639120294326972 ) ) ;
#21800=CARTESIAN_POINT ( 'NONE',  ( 4.944772684328679446, 135.1851862821014549, -11.48171059495397373 ) ) ;
#21801=CARTESIAN_POINT ( 'NONE',  ( -10.41470757995802643, 142.9999999999999716, 3.937110085335259413 ) ) ;
#21810=CARTESIAN_POINT ( 'NONE',  ( -8.962234695871565293, 136.4398137178985735, -8.715434833792128799 ) ) ;
#21816=CARTESIAN_POINT ( 'NONE',  ( -11.61527771782809282, 34.66481371789854649, -4.622313124798832717 ) ) ;
#21818=CARTESIAN_POINT ( 'NONE',  ( -14.25334919248795096, 107.1148137178985564, 6.092822981423662299 ) ) ;
#21825=CARTESIAN_POINT ( 'NONE',  ( 10.69584247140445221, 126.8476862821014635, -6.932735513423970097 ) ) ;
#21832=CARTESIAN_POINT ( 'NONE',  ( 12.50000000000000355, 136.9101862821014777, 0.1745138560725507937 ) ) ;
#21838=CARTESIAN_POINT ( 'NONE',  ( 8.632099005475504683, 110.7476862821014691, 13.23911966647218996 ) ) ;
#21839=CARTESIAN_POINT ( 'NONE',  ( -8.843639120294326972, 113.3351862821014606, 3.474262827703335166 ) ) ;
#21841=CARTESIAN_POINT ( 'NONE',  ( 4.944772684328679446, 6.385186282101440014, -11.48171059495397373 ) ) ;
#21845=CARTESIAN_POINT ( 'NONE',  ( -9.465287035748065847, 86.59768628210143504, -2.064181346179273735 ) ) ;
#21847=CARTESIAN_POINT ( 'NONE',  ( -8.710071997420207879, 125.5148137178985763, 3.796722387233182339 ) ) ;
#21853=CARTESIAN_POINT ( 'NONE',  ( 0.1745138560723095977, 59.38981371789856212, 9.500000000000005329 ) ) ;
#21856=CARTESIAN_POINT ( 'NONE',  ( -11.61527771782809282, 80.66481371789856780, -4.622313124798832717 ) ) ;
#21860=CARTESIAN_POINT ( 'NONE',  ( -2.311890736173448424, 41.27731371789855075, 12.53471296425189330 ) ) ;
#21863=CARTESIAN_POINT ( 'NONE',  ( 10.49813415415989581, 27.37268628210144783, 7.228626920339068285 ) ) ;
#21868=CARTESIAN_POINT ( 'NONE',  ( -12.46528703574811558, 70.60231371789856780, 2.660918448318003726 ) ) ;
#21873=CARTESIAN_POINT ( 'NONE',  ( 15.46528703574811736, 38.40231371789853654, -3.257655550456947768 ) ) ;
#21876=CARTESIAN_POINT ( 'NONE',  ( 0.1745138560725515708, 70.21018628210144641, -12.50000000000000355 ) ) ;
#21877=CARTESIAN_POINT ( 'NONE',  ( -14.38691631536207183, 30.53518628210144570, 5.770363421893814682 ) ) ;
#21883=CARTESIAN_POINT ( 'NONE',  ( 0.1745138560725837118, 24.21018628210144996, -15.50000000000000533 ) ) ;
#21890=CARTESIAN_POINT ( 'NONE',  ( 11.61527771782819940, 7.535186282101452804, -4.622313124798573369 ) ) ;
#21892=CARTESIAN_POINT ( 'NONE',  ( 1.715153634034445762, 128.6773137178985280, -9.534712964251895073 ) ) ;
#21897=CARTESIAN_POINT ( 'NONE',  ( -12.50000000000000355, 135.2898137178985678, 0.1745138560722786503 ) ) ;
#21904=CARTESIAN_POINT ( 'NONE',  ( -11.61527771782819940, 39.73518628210144499, 4.622313124798574258 ) ) ;
#21912=CARTESIAN_POINT ( 'NONE',  ( 11.61527771782819940, 71.93518628210145494, -4.622313124798573369 ) ) ;
#21913=CARTESIAN_POINT ( 'NONE',  ( 2.908627838312458636, 9.077313717898549683, -15.53471296425188442 ) ) ;
#21919=CARTESIAN_POINT ( 'NONE',  ( -6.932735513424201912, 124.6523137178985650, 10.69584247140429412 ) ) ;
#21927=CARTESIAN_POINT ( 'NONE',  ( 15.50000000000000533, 93.88981371789856212, -0.1745138560722452326 ) ) ;
#21932=CARTESIAN_POINT ( 'NONE',  ( 7.228626920339068285, 126.2726862821014606, -10.49813415415989581 ) ) ;
#21933=CARTESIAN_POINT ( 'NONE',  ( -14.38691631536207183, 76.53518628210146346, 5.770363421893814682 ) ) ;
#21936=CARTESIAN_POINT ( 'NONE',  ( -13.04141134922759804, 77.97268628210142083, -8.927990412390657937 ) ) ;
#21941=CARTESIAN_POINT ( 'NONE',  ( -5.233372021372430183, 41.74768628210143362, -8.152565276336710909 ) ) ;
#21945=CARTESIAN_POINT ( 'NONE',  ( 10.49813415415989581, 54.97268628210144925, 7.228626920339068285 ) ) ;
#21948=CARTESIAN_POINT ( 'NONE',  ( 7.954856959092191815, 36.57268628210144357, 5.529263428287477744 ) ) ;
#21958=CARTESIAN_POINT ( 'NONE',  ( 12.50000000000000355, 84.68981371789854506, -0.1745138560722771515 ) ) ;
#21959=CARTESIAN_POINT ( 'NONE',  ( -0.1745138560725500443, 93.21018628210146062, 12.50000000000000355 ) ) ;
#21964=CARTESIAN_POINT ( 'NONE',  ( 15.46528703574811736, 66.00231371789855928, -3.257655550456947768 ) ) ;
#21971=CARTESIAN_POINT ( 'NONE',  ( 9.465287035748106703, 47.60231371789853938, -2.064181346179063237 ) ) ;
#21974=CARTESIAN_POINT ( 'NONE',  ( -5.233372021372612259, 97.05231371789855643, 8.152565276336593669 ) ) ;
#21976=CARTESIAN_POINT ( 'NONE',  ( -8.715434833792127023, 23.73981371789854578, 8.962234695871568846 ) ) ;
#21977=CARTESIAN_POINT ( 'NONE',  ( -12.53471296425194836, 76.82268628210145778, 2.311890736173176641 ) ) ;
#21986=CARTESIAN_POINT ( 'NONE',  ( 8.843639120294328748, 99.53518628210146346, -3.474262827703334722 ) ) ;
#21988=CARTESIAN_POINT ( 'NONE',  ( -8.715434833791929847, 124.2601862821014578, -8.962234695871762469 ) ) ;
#21998=CARTESIAN_POINT ( 'NONE',  ( 0.1745138560722779009, 132.9898137178985564, 12.50000000000000355 ) ) ;
#22005=CARTESIAN_POINT ( 'NONE',  ( -2.908627838312453306, 105.6773137178985706, 15.53471296425188797 ) ) ;
#22011=CARTESIAN_POINT ( 'NONE',  ( -12.46528703574805697, 123.3976862821014606, -2.660918448318280838 ) ) ;
#22020=CARTESIAN_POINT ( 'NONE',  ( -7.228626920339069173, 130.8726862821014834, 10.49813415415989581 ) ) ;
#22025=CARTESIAN_POINT ( 'NONE',  ( -8.632099005475501130, 124.5476862821014663, -13.23911966647218996 ) ) ;
#22027=CARTESIAN_POINT ( 'NONE',  ( 10.49813415415989581, 18.17268628210144854, 7.228626920339068285 ) ) ;
#22031=CARTESIAN_POINT ( 'NONE',  ( -2.064181346179269738, 84.29768628210146630, 9.465287035748067623 ) ) ;
#22034=CARTESIAN_POINT ( 'NONE',  ( -9.534712964251895073, 126.3773137178985309, -1.715153634034446428 ) ) ;
#22041=CARTESIAN_POINT ( 'NONE',  ( -6.840914352311947333, 53.63981371789855501, -6.594114490232462877 ) ) ;
#22045=CARTESIAN_POINT ( 'NONE',  ( 0.1745138560722779009, 59.38981371789856212, 12.50000000000000355 ) ) ;
#22049=CARTESIAN_POINT ( 'NONE',  ( 12.46528703574811558, 38.40231371789855075, -2.660918448318005503 ) ) ;
#22051=CARTESIAN_POINT ( 'NONE',  ( -10.49813415415989581, 13.57268628210145600, -7.228626920339068285 ) ) ;
#22057=CARTESIAN_POINT ( 'NONE',  ( -4.622313124798826500, 69.16481371789855359, 11.61527771782809637 ) ) ;
#22064=CARTESIAN_POINT ( 'NONE',  ( 0.1745138560722461762, 31.78981371789855004, 15.50000000000000533 ) ) ;
#22067=CARTESIAN_POINT ( 'NONE',  ( 7.228626920339068285, 71.07268628210144357, -10.49813415415989581 ) ) ;
#22068=CARTESIAN_POINT ( 'NONE',  ( -3.257655550457281723, 10.69768628210143646, 15.46528703574804986 ) ) ;
#22072=CARTESIAN_POINT ( 'NONE',  ( 15.53471296425195369, 26.22268628210144925, -2.908627838312120684 ) ) ;
#22079=CARTESIAN_POINT ( 'NONE',  ( 2.311890736173175753, 10.12268628210144428, 12.53471296425194836 ) ) ;
#22081=CARTESIAN_POINT ( 'NONE',  ( 3.796722387233182339, 114.0148137178985763, 8.710071997420207879 ) ) ;
#22087=CARTESIAN_POINT ( 'NONE',  ( -11.61527771782809282, 135.8648137178985849, -4.622313124798832717 ) ) ;
#22093=CARTESIAN_POINT ( 'NONE',  ( 4.622313124798573369, 28.23518628210144854, 11.61527771782819940 ) ) ;
#22101=CARTESIAN_POINT ( 'NONE',  ( 7.228626920339068285, 71.07268628210144357, -10.49813415415989581 ) ) ;
#22102=CARTESIAN_POINT ( 'NONE',  ( 15.53471296425195369, 136.6226862821014549, -2.908627838312120684 ) ) ;
#22108=CARTESIAN_POINT ( 'NONE',  ( -8.715434833792127023, 115.7398137178985706, 8.962234695871568846 ) ) ;
#22114=CARTESIAN_POINT ( 'NONE',  ( 15.46528703574811736, 93.60231371789855359, -3.257655550456947768 ) ) ;
#22118=CARTESIAN_POINT ( 'NONE',  ( 2.660918448318279950, 125.6976862821014578, -12.46528703574805697 ) ) ;
#22119=CARTESIAN_POINT ( 'NONE',  ( -10.83675517735155047, 59.86018628210145209, -11.08355503943142750 ) ) ;
#22123=CARTESIAN_POINT ( 'NONE',  ( -13.04141134922759804, 87.17268628210142367, -8.927990412390657937 ) ) ;
#22127=CARTESIAN_POINT ( 'NONE',  ( 3.796722387233379514, 43.18518628210144072, -8.710071997420127943 ) ) ;
#22132=CARTESIAN_POINT ( 'NONE',  ( 11.48171059495397728, 54.68518628210144783, 4.944772684328674117 ) ) ;
#22135=CARTESIAN_POINT ( 'NONE',  ( 8.152565276336714462, 34.84768628210143504, -5.233372021372432847 ) ) ;
#22144=CARTESIAN_POINT ( 'NONE',  ( -12.50000000000000355, 89.28981371789855359, 0.1745138560722786503 ) ) ;
#22145=CARTESIAN_POINT ( 'NONE',  ( -12.50000000000000355, 86.31018628210145494, -0.1745138560725492671 ) ) ;
#22151=CARTESIAN_POINT ( 'NONE',  ( -11.08355503943118592, 53.63981371789855501, -10.83675517735179383 ) ) ;
#22159=CARTESIAN_POINT ( 'NONE',  ( 3.474262827703532341, 46.16481371789854649, -8.843639120294245259 ) ) ;
#22161=CARTESIAN_POINT ( 'NONE',  ( -7.954856959092309943, 88.42731371789855643, 5.529263428287300108 ) ) ;
#22163=CARTESIAN_POINT ( 'NONE',  ( -2.660918448318004614, 8.502313717898557499, -12.46528703574811558 ) ) ;
#22164=CARTESIAN_POINT ( 'NONE',  ( 11.61527771782819940, 71.93518628210145494, -4.622313124798573369 ) ) ;
#22172=CARTESIAN_POINT ( 'NONE',  ( -8.710071997420127943, 86.88518628210145778, -3.796722387233380402 ) ) ;
#22175=CARTESIAN_POINT ( 'NONE',  ( 4.622313124798573369, 120.2351862821014663, 11.61527771782819940 ) ) ;
#22186=CARTESIAN_POINT ( 'NONE',  ( 12.53471296425189330, 140.1773137178985849, 2.311890736173451977 ) ) ;
#22195=CARTESIAN_POINT ( 'NONE',  ( -2.908627838312453306, 114.8773137178985735, 15.53471296425188797 ) ) ;
#22201=CARTESIAN_POINT ( 'NONE',  ( 8.962234695871762469, 108.1601862821014635, -8.715434833791931624 ) ) ;
#22207=CARTESIAN_POINT ( 'NONE',  ( -11.48171059495397373, 114.4851862821014521, -4.944772684328680334 ) ) ;
#22212=CARTESIAN_POINT ( 'NONE',  ( 15.46528703574804986, 118.7976862821014521, 3.257655550457285720 ) ) ;
#22215=CARTESIAN_POINT ( 'NONE',  ( 12.50000000000000355, 17.31018628210144428, 0.1745138560725507937 ) ) ;
#22218=CARTESIAN_POINT ( 'NONE',  ( 6.840914352312096547, 80.56018628210146915, -6.594114490232313663 ) ) ;
#22219=CARTESIAN_POINT ( 'NONE',  ( 7.954856959092311719, 129.8273137178985905, -5.529263428287300108 ) ) ;
#22227=CARTESIAN_POINT ( 'NONE',  ( 3.796722387233182339, 58.81481371789855217, 8.710071997420207879 ) ) ;
#22232=CARTESIAN_POINT ( 'NONE',  ( -7.228626920338836470, 63.12731371789855217, -10.49813415416005213 ) ) ;
#22236=CARTESIAN_POINT ( 'NONE',  ( 7.228626920338837358, 30.92731371789854222, 10.49813415416005036 ) ) ;
#22242=CARTESIAN_POINT ( 'NONE',  ( -10.69584247140444866, 11.84768628210144925, 6.932735513423972762 ) ) ;
#22246=CARTESIAN_POINT ( 'NONE',  ( -4.944772684328424539, 63.41481371789856070, -11.48171059495408031 ) ) ;
#22251=CARTESIAN_POINT ( 'NONE',  ( -14.38691631536193860, 43.86481371789854933, -5.770363421894132649 ) ) ;
#22253=CARTESIAN_POINT ( 'NONE',  ( -12.50000000000000355, 21.91018628210143859, -0.1745138560725492671 ) ) ;
#22255=CARTESIAN_POINT ( 'NONE',  ( 6.932735513423970097, 73.94768628210145778, 10.69584247140445044 ) ) ;
#22256=CARTESIAN_POINT ( 'NONE',  ( 15.53471296425195369, 7.822686282101448896, -2.908627838312120684 ) ) ;
#22260=CARTESIAN_POINT ( 'NONE',  ( 13.04141134922759804, 36.57268628210144357, 8.927990412390657937 ) ) ;
#22267=CARTESIAN_POINT ( 'NONE',  ( -1.715153634034442431, 114.8773137178985735, 9.534712964251900402 ) ) ;
#22273=CARTESIAN_POINT ( 'NONE',  ( -6.932735513424201912, 124.6523137178985650, 10.69584247140429412 ) ) ;
#22279=CARTESIAN_POINT ( 'NONE',  ( -2.660918448318275509, 38.29768628210145209, 12.46528703574805874 ) ) ;
#22286=CARTESIAN_POINT ( 'NONE',  ( 8.715434833791931624, 64.46018628210146062, 8.962234695871760692 ) ) ;
#22292=CARTESIAN_POINT ( 'NONE',  ( -10.49813415416004858, 116.0273137178985650, 7.228626920338839135 ) ) ;
#22298=CARTESIAN_POINT ( 'NONE',  ( 15.53471296425188797, 103.3773137178985451, 2.908627838312457747 ) ) ;
#22302=CARTESIAN_POINT ( 'NONE',  ( -6.932735513423968321, 115.3476862821014635, -10.69584247140445221 ) ) ;
#22303=CARTESIAN_POINT ( 'NONE',  ( 14.38691631536207538, 62.73518628210145920, -5.770363421893813793 ) ) ;
#22306=CARTESIAN_POINT ( 'NONE',  ( -0.1745138560725817967, 84.01018628210145778, 15.50000000000000533 ) ) ;
#22309=CARTESIAN_POINT ( 'NONE',  ( -7.954856959092191815, 13.57268628210145422, -5.529263428287477744 ) ) ;
#22313=CARTESIAN_POINT ( 'NONE',  ( -4.944772684328673229, 66.18518628210144072, 11.48171059495397728 ) ) ;
#22316=CARTESIAN_POINT ( 'NONE',  ( 3.474262827703335166, 19.03518628210144570, 8.843639120294326972 ) ) ;
#22327=CARTESIAN_POINT ( 'NONE',  ( -7.228626920338836470, 81.52731371789855075, -10.49813415416005213 ) ) ;
#22328=CARTESIAN_POINT ( 'NONE',  ( 11.48171059495397728, 82.28518628210146346, 4.944772684328674117 ) ) ;
#22333=CARTESIAN_POINT ( 'NONE',  ( -2.908627838312453306, 50.47731371789854649, 15.53471296425188797 ) ) ;
#22338=CARTESIAN_POINT ( 'NONE',  ( -0.1745138560723084320, 45.58981371789855785, -9.500000000000005329 ) ) ;
#22341=CARTESIAN_POINT ( 'NONE',  ( 2.064181346179061460, 86.70231371789851949, 9.465287035748106703 ) ) ;
#22343=CARTESIAN_POINT ( 'NONE',  ( -11.61527771782809282, 7.064813717898549505, -4.622313124798832717 ) ) ;
#22345=CARTESIAN_POINT ( 'NONE',  ( -10.49813415415989581, 59.57268628210145778, -7.228626920339068285 ) ) ;
#22354=CARTESIAN_POINT ( 'NONE',  ( -2.064181346179269738, 75.09768628210143504, 9.465287035748067623 ) ) ;
#22357=CARTESIAN_POINT ( 'NONE',  ( 0.1745138560725515708, 107.0101862821014578, -12.50000000000000355 ) ) ;
#22371=CARTESIAN_POINT ( 'NONE',  ( -7.228626920338836470, 136.7273137178985678, -10.49813415416005213 ) ) ;
#22376=CARTESIAN_POINT ( 'NONE',  ( 0.1745138560722779009, 13.38981371789854613, 12.50000000000000355 ) ) ;
#22378=CARTESIAN_POINT ( 'NONE',  ( -15.50000000000000533, 116.8898137178985621, 0.1745138560722471477 ) ) ;
#22383=CARTESIAN_POINT ( 'NONE',  ( 4.622313124798573369, 111.0351862821014635, 11.61527771782819940 ) ) ;
#22389=CARTESIAN_POINT ( 'NONE',  ( 0.1745138560725515708, 125.4101862821014635, -12.50000000000000355 ) ) ;
#22395=CARTESIAN_POINT ( 'NONE',  ( 13.04141134922759804, 128.5726862821014436, 8.927990412390657937 ) ) ;
#22398=CARTESIAN_POINT ( 'NONE',  ( 12.46528703574805874, 17.59768628210143859, 2.660918448318279950 ) ) ;
#22403=CARTESIAN_POINT ( 'NONE',  ( -8.843639120294326972, 76.53518628210146346, 3.474262827703335166 ) ) ;
#22411=CARTESIAN_POINT ( 'NONE',  ( -8.710071997420207879, 61.11481371789854933, 3.796722387233182339 ) ) ;
#22416=CARTESIAN_POINT ( 'NONE',  ( 2.660918448318003282, 68.30231371789855643, 12.46528703574811558 ) ) ;
#22419=CARTESIAN_POINT ( 'NONE',  ( -4.944772684328424539, 35.81481371789854506, -11.48171059495408031 ) ) ;
#22428=CARTESIAN_POINT ( 'NONE',  ( 12.50000000000000355, 75.48981371789855643, -0.1745138560722771515 ) ) ;
#22434=CARTESIAN_POINT ( 'NONE',  ( -0.1745138560722442889, 45.58981371789855785, -15.50000000000000533 ) ) ;
#22437=CARTESIAN_POINT ( 'NONE',  ( -4.622313124798576922, 23.63518628210144357, -11.61527771782819762 ) ) ;
#22438=CARTESIAN_POINT ( 'NONE',  ( -2.660918448318275509, 75.09768628210143504, 12.46528703574805874 ) ) ;
#22439=CARTESIAN_POINT ( 'NONE',  ( 14.38691631536207538, 16.73518628210143788, -5.770363421893813793 ) ) ;
#22443=CARTESIAN_POINT ( 'NONE',  ( -8.632099005475501130, 23.34768628210144570, -13.23911966647218996 ) ) ;
#22451=CARTESIAN_POINT ( 'NONE',  ( -3.474262827703527901, 115.1648137178985678, 8.843639120294245259 ) ) ;
#22457=CARTESIAN_POINT ( 'NONE',  ( -2.660918448318005058, 118.9023137178985507, -12.46528703574811558 ) ) ;
#22470=CARTESIAN_POINT ( 'NONE',  ( -4.944772684328673229, 56.98518628210144499, 11.48171059495397728 ) ) ;
#22479=CARTESIAN_POINT ( 'NONE',  ( 4.944772684328420986, 114.0148137178985621, 11.48171059495408208 ) ) ;
#22487=CARTESIAN_POINT ( 'NONE',  ( 14.25334919248795451, 102.5148137178985621, -6.092822981423661410 ) ) ;
#22490=CARTESIAN_POINT ( 'NONE',  ( 12.53471296425194836, 118.2226862821014635, -2.311890736173178418 ) ) ;
#22491=CARTESIAN_POINT ( 'NONE',  ( -14.38691631536207183, 58.13518628210145067, 5.770363421893814682 ) ) ;
#22494=CARTESIAN_POINT ( 'NONE',  ( 14.25334919248782661, 82.28518628210146346, 6.092822981423971385 ) ) ;
#22497=CARTESIAN_POINT ( 'NONE',  ( 8.843639120294328748, 16.73518628210143788, -3.474262827703334722 ) ) ;
#22501=CARTESIAN_POINT ( 'NONE',  ( -11.61527771782819940, 58.13518628210144357, 4.622313124798574258 ) ) ;
#22504=CARTESIAN_POINT ( 'NONE',  ( 1.715153634034233487, 28.52268628210144286, 9.534712964251941258 ) ) ;
#22515=CARTESIAN_POINT ( 'NONE',  ( -10.69584247140444866, 94.64768628210146062, 6.932735513423972762 ) ) ;
#22521=CARTESIAN_POINT ( 'NONE',  ( 14.38691631536194393, 48.46481371789856496, 5.770363421894124656 ) ) ;
#22526=CARTESIAN_POINT ( 'NONE',  ( -5.529263428287297444, 35.52731371789855075, -7.954856959092311719 ) ) ;
#22528=CARTESIAN_POINT ( 'NONE',  ( -9.534712964251895073, 89.57731371789856212, -1.715153634034446428 ) ) ;
#22530=CARTESIAN_POINT ( 'NONE',  ( -14.25334919248795096, 143.9148137178985678, 6.092822981423662299 ) ) ;
#22532=CARTESIAN_POINT ( 'NONE',  ( -7.228626920339069173, 66.47268628210144925, 10.49813415415989581 ) ) ;
#22540=CARTESIAN_POINT ( 'NONE',  ( -9.534712964251941258, 67.62268628210145494, 1.715153634034234154 ) ) ;
#22542=CARTESIAN_POINT ( 'NONE',  ( -11.61527771782819940, 113.3351862821014606, 4.622313124798574258 ) ) ;
#22554=CARTESIAN_POINT ( 'NONE',  ( -2.064181346179062349, 8.502313717898553946, -9.465287035748106703 ) ) ;
#22555=CARTESIAN_POINT ( 'NONE',  ( -2.660918448318275509, 139.4976862821014549, 12.46528703574805874 ) ) ;
#22559=CARTESIAN_POINT ( 'NONE',  ( -11.61527771782809282, 16.26481371789853370, -4.622313124798832717 ) ) ;
#22561=CARTESIAN_POINT ( 'NONE',  ( 3.257655550456945548, 114.3023137178985422, 15.46528703574811736 ) ) ;
#22567=CARTESIAN_POINT ( 'NONE',  ( 12.46528703574805874, 118.7976862821014663, 2.660918448318279950 ) ) ;
#22575=CARTESIAN_POINT ( 'NONE',  ( 10.49813415415989581, 128.5726862821014720, 7.228626920339068285 ) ) ;
#22581=CARTESIAN_POINT ( 'NONE',  ( 8.927990412390657937, 98.67268628210146630, -13.04141134922759804 ) ) ;
#22582=CARTESIAN_POINT ( 'NONE',  ( 4.622313124798573369, 19.03518628210144925, 11.61527771782819940 ) ) ;
#22584=CARTESIAN_POINT ( 'NONE',  ( -2.064181346179269738, 130.2976862821014379, 9.465287035748067623 ) ) ;
#22591=CARTESIAN_POINT ( 'NONE',  ( 3.796722387233379514, 70.78518628210143504, -8.710071997420127943 ) ) ;
#22598=CARTESIAN_POINT ( 'NONE',  ( -2.064181346179062349, 63.70231371789854791, -9.465287035748106703 ) ) ;
#22603=CARTESIAN_POINT ( 'NONE',  ( -11.61527771782809282, 62.26481371789854791, -4.622313124798832717 ) ) ;
#22606=CARTESIAN_POINT ( 'NONE',  ( -11.48171059495408208, 24.31481371789855217, 4.944772684328421875 ) ) ;
#22622=CARTESIAN_POINT ( 'NONE',  ( 2.908627838312458636, 36.67731371789854933, -15.53471296425188442 ) ) ;
#22624=CARTESIAN_POINT ( 'NONE',  ( 10.49813415415989581, 8.972686282101431487, 7.228626920339068285 ) ) ;
#22625=CARTESIAN_POINT ( 'NONE',  ( 12.53471296425194836, 53.82268628210144357, -2.311890736173178418 ) ) ;
#22627=CARTESIAN_POINT ( 'NONE',  ( 15.53471296425195369, 17.02268628210144996, -2.908627838312120684 ) ) ;
#22631=CARTESIAN_POINT ( 'NONE',  ( -12.53471296425194836, 141.2226862821014493, 2.311890736173176641 ) ) ;
#22637=CARTESIAN_POINT ( 'NONE',  ( 8.715434833791931624, 9.260186282101429356, 8.962234695871760692 ) ) ;
#22639=CARTESIAN_POINT ( 'NONE',  ( 5.233372021372610483, 120.0523137178985280, -8.152565276336593669 ) ) ;
#22646=CARTESIAN_POINT ( 'NONE',  ( 8.715434833792128799, 120.3398137178985650, -8.962234695871567070 ) ) ;
#22661=CARTESIAN_POINT ( 'NONE',  ( -12.50000000000000355, 58.71018628210145351, -0.1745138560725492671 ) ) ;
#22668=CARTESIAN_POINT ( 'NONE',  ( 10.69584247140429589, 113.1523137178985650, 6.932735513424201024 ) ) ;
#22673=CARTESIAN_POINT ( 'NONE',  ( 3.257655550456945548, 95.90231371789855075, 15.46528703574811736 ) ) ;
#22678=CARTESIAN_POINT ( 'NONE',  ( -2.311890736173176641, 115.9226862821014521, -12.53471296425194836 ) ) ;
#22679=CARTESIAN_POINT ( 'NONE',  ( -14.25334919248782306, 68.48518628210145209, -6.092822981423979378 ) ) ;
#22683=CARTESIAN_POINT ( 'NONE',  ( -10.83675517735155047, 78.26018628210144357, -11.08355503943142750 ) ) ;
#22686=CARTESIAN_POINT ( 'NONE',  ( -5.529263428287477744, 20.47268628210143859, 7.954856959092191815 ) ) ;
#22690=CARTESIAN_POINT ( 'NONE',  ( -12.46528703574805697, 58.99768628210144783, -2.660918448318280838 ) ) ;
#22693=CARTESIAN_POINT ( 'NONE',  ( 3.796722387233379514, 24.78518628210144215, -8.710071997420127943 ) ) ;
#22707=CARTESIAN_POINT ( 'NONE',  ( 4.622313124798573369, 65.03518628210144925, 11.61527771782819940 ) ) ;
#22712=CARTESIAN_POINT ( 'NONE',  ( 10.83675517735179206, 37.53981371789855359, -11.08355503943118769 ) ) ;
#22718=CARTESIAN_POINT ( 'NONE',  ( 3.474262827703532341, 36.96481371789853654, -8.843639120294245259 ) ) ;
#22720=CARTESIAN_POINT ( 'NONE',  ( 3.796722387233182339, 86.41481371789855359, 8.710071997420207879 ) ) ;
#22722=CARTESIAN_POINT ( 'NONE',  ( 8.927990412390371944, 141.3273137178985621, 13.04141134922778811 ) ) ;
#22723=CARTESIAN_POINT ( 'NONE',  ( -0.1745138560725500443, 65.61018628210145209, 12.50000000000000355 ) ) ;
#22729=CARTESIAN_POINT ( 'NONE',  ( 6.594114490232313663, 82.86018628210146630, 6.840914352312096547 ) ) ;
#22731=CARTESIAN_POINT ( 'NONE',  ( 8.715434833791931624, 119.6601862821014493, 8.962234695871760692 ) ) ;
#22744=CARTESIAN_POINT ( 'NONE',  ( 10.49813415416005213, 129.8273137178985905, -7.228626920338837358 ) ) ;
#22749=CARTESIAN_POINT ( 'NONE',  ( 2.660918448318003282, 13.10231371789855004, 12.46528703574811558 ) ) ;
#22750=CARTESIAN_POINT ( 'NONE',  ( 14.25334919248795451, 102.5148137178985621, -6.092822981423661410 ) ) ;
#22751=CARTESIAN_POINT ( 'NONE',  ( -11.61527771782819940, 104.1351862821014578, 4.622313124798574258 ) ) ;
#22754=CARTESIAN_POINT ( 'NONE',  ( 2.311890736173175753, 120.5226862821014606, 12.53471296425194836 ) ) ;
#22760=CARTESIAN_POINT ( 'NONE',  ( -2.311890736173176641, 125.1226862821014549, -12.53471296425194836 ) ) ;
#22766=CARTESIAN_POINT ( 'NONE',  ( -2.908627838312119351, 97.52268628210144641, -15.53471296425195369 ) ) ;
#22767=CARTESIAN_POINT ( 'NONE',  ( -2.660918448318275509, 10.69768628210143646, 12.46528703574805874 ) ) ;
#22769=CARTESIAN_POINT ( 'NONE',  ( -8.710071997420127943, 123.6851862821014549, -3.796722387233380402 ) ) ;
#22774=CARTESIAN_POINT ( 'NONE',  ( 5.529263428287477744, 61.87268628210144783, -7.954856959092191815 ) ) ;
#22781=CARTESIAN_POINT ( 'NONE',  ( 0.1745138560723095977, 40.98981371789854933, 9.500000000000005329 ) ) ;
#22785=CARTESIAN_POINT ( 'NONE',  ( -8.715434833792127023, 69.73981371789855643, 8.962234695871568846 ) ) ;
#22788=CARTESIAN_POINT ( 'NONE',  ( 11.61527771782809637, 20.86481371789854222, 4.622313124798827388 ) ) ;
#22792=CARTESIAN_POINT ( 'NONE',  ( 4.944772684328679446, 6.385186282101440014, -11.48171059495397373 ) ) ;
#22805=CARTESIAN_POINT ( 'NONE',  ( -15.53471296425188442, 15.97731371789853405, -2.908627838312459080 ) ) ;
#22807=CARTESIAN_POINT ( 'NONE',  ( 12.50000000000000355, 17.31018628210144428, 0.1745138560725507937 ) ) ;
#22808=CARTESIAN_POINT ( 'NONE',  ( -12.50000000000000355, 40.31018628210144783, -0.1745138560725492671 ) ) ;
#22813=CARTESIAN_POINT ( 'NONE',  ( -5.770363421893818234, 14.43518628210144072, -14.38691631536207005 ) ) ;
#22821=CARTESIAN_POINT ( 'NONE',  ( 3.474262827703532341, 101.3648137178985706, -8.843639120294245259 ) ) ;
#22830=CARTESIAN_POINT ( 'NONE',  ( -11.48171059495408208, 116.3148137178985593, 4.944772684328421875 ) ) ;
#22844=CARTESIAN_POINT ( 'NONE',  ( -10.49813415415989581, 59.57268628210145778, -7.228626920339068285 ) ) ;
#22850=CARTESIAN_POINT ( 'NONE',  ( -10.49813415416004858, 97.62731371789855928, 7.228626920338839135 ) ) ;
#22855=CARTESIAN_POINT ( 'NONE',  ( -11.08355503943118592, 72.03981371789855359, -10.83675517735179383 ) ) ;
#22860=CARTESIAN_POINT ( 'NONE',  ( 2.311890736173175753, 102.1226862821014691, 12.53471296425194836 ) ) ;
#22861=CARTESIAN_POINT ( 'NONE',  ( 2.908627838312118019, 65.32268628210144357, 15.53471296425195369 ) ) ;
#22864=CARTESIAN_POINT ( 'NONE',  ( 14.38691631536207538, 71.93518628210142651, -5.770363421893813793 ) ) ;
#22869=CARTESIAN_POINT ( 'NONE',  ( 2.311890736173175753, 37.72268628210144215, 12.53471296425194836 ) ) ;
#22872=CARTESIAN_POINT ( 'NONE',  ( 3.474262827703335166, 28.23518628210144854, 8.843639120294326972 ) ) ;
#22882=CARTESIAN_POINT ( 'NONE',  ( 8.962234695871762469, 71.36018628210145209, -8.715434833791931624 ) ) ;
#22889=CARTESIAN_POINT ( 'NONE',  ( 15.46528703574811736, 47.60231371789853938, -3.257655550456947768 ) ) ;
#22897=CARTESIAN_POINT ( 'NONE',  ( -9.534712964251895073, 15.97731371789853405, -1.715153634034446428 ) ) ;
#22902=CARTESIAN_POINT ( 'NONE',  ( 6.932735513424201024, 18.85231371789855714, -10.69584247140429412 ) ) ;
#22905=CARTESIAN_POINT ( 'NONE',  ( 2.660918448318279950, 61.29768628210143788, -12.46528703574805697 ) ) ;
#22914=CARTESIAN_POINT ( 'NONE',  ( -9.500000000000005329, 77.11018628210145209, -0.1745138560725176813 ) ) ;
#22917=CARTESIAN_POINT ( 'NONE',  ( -12.46528703574805697, 104.9976862821014691, -2.660918448318280838 ) ) ;
#22929=CARTESIAN_POINT ( 'NONE',  ( -12.53471296425189152, 126.3773137178985593, -2.311890736173453753 ) ) ;
#22930=CARTESIAN_POINT ( 'NONE',  ( 4.622313124798573369, 120.2351862821014663, 11.61527771782819940 ) ) ;
#22936=CARTESIAN_POINT ( 'NONE',  ( 5.770363421894130873, 92.16481371789855359, -14.38691631536193860 ) ) ;
#22937=CARTESIAN_POINT ( 'NONE',  ( -0.1745138560725500443, 102.4101862821014493, 12.50000000000000355 ) ) ;
#22941=CARTESIAN_POINT ( 'NONE',  ( 2.311890736173175753, 111.3226862821014720, 12.53471296425194836 ) ) ;
#22946=CARTESIAN_POINT ( 'NONE',  ( 6.932735513423970097, 119.9476862821014578, 10.69584247140445044 ) ) ;
#22952=CARTESIAN_POINT ( 'NONE',  ( 15.53471296425195369, 109.0226862821014606, -2.908627838312120684 ) ) ;
#22953=CARTESIAN_POINT ( 'NONE',  ( 12.46528703574805874, 17.59768628210144215, 2.660918448318279950 ) ) ;
#22956=CARTESIAN_POINT ( 'NONE',  ( 6.840914352312096547, 135.7601862821014720, -6.594114490232313663 ) ) ;
#22960=CARTESIAN_POINT ( 'NONE',  ( -2.064181346179269738, 56.69768628210144357, 9.465287035748067623 ) ) ;
#22967=CARTESIAN_POINT ( 'NONE',  ( 6.840914352311949109, 30.63981371789855146, 6.594114490232462877 ) ) ;
#22972=CARTESIAN_POINT ( 'NONE',  ( -12.53471296425189152, 52.77731371789855075, -2.311890736173453309 ) ) ;
#22975=CARTESIAN_POINT ( 'NONE',  ( -12.53471296425189152, 15.97731371789853760, -2.311890736173453753 ) ) ;
#22989=CARTESIAN_POINT ( 'NONE',  ( -0.1745138560722442889, 27.18981371789855572, -15.50000000000000533 ) ) ;
#22991=CARTESIAN_POINT ( 'NONE',  ( 2.311890736173175753, 10.12268628210144428, 12.53471296425194836 ) ) ;
#22992=CARTESIAN_POINT ( 'NONE',  ( -11.61527771782819940, 39.73518628210144499, 4.622313124798574258 ) ) ;
#23003=CARTESIAN_POINT ( 'NONE',  ( 3.796722387233182339, 95.61481371789857064, 8.710071997420207879 ) ) ;
#23010=CARTESIAN_POINT ( 'NONE',  ( -7.228626920338836470, 109.1273137178985593, -10.49813415416005213 ) ) ;
#23014=CARTESIAN_POINT ( 'NONE',  ( 8.962234695871567070, 58.23981371789854933, 8.715434833792127023 ) ) ;
#23025=CARTESIAN_POINT ( 'NONE',  ( -6.932735513423968321, 50.94768628210144357, -10.69584247140445221 ) ) ;
#23032=CARTESIAN_POINT ( 'NONE',  ( 2.660918448318002838, 105.1023137178985536, 12.46528703574811558 ) ) ;
#23038=CARTESIAN_POINT ( 'NONE',  ( -15.50000000000000533, 70.88981371789854791, 0.1745138560722471477 ) ) ;
#23042=CARTESIAN_POINT ( 'NONE',  ( 2.660918448318279950, 107.2976862821014521, -12.46528703574805697 ) ) ;
#23043=CARTESIAN_POINT ( 'NONE',  ( 14.38691631536207538, 44.33518628210144641, -5.770363421893813793 ) ) ;
#23048=CARTESIAN_POINT ( 'NONE',  ( 15.46528703574804986, 63.59768628210142793, 3.257655550457285720 ) ) ;
#23052=CARTESIAN_POINT ( 'NONE',  ( -4.944772684328673229, 47.78518628210144925, 11.48171059495397728 ) ) ;
#23055=CARTESIAN_POINT ( 'NONE',  ( -8.843639120294326972, 12.13518628210144712, 3.474262827703335166 ) ) ;
#23065=CARTESIAN_POINT ( 'NONE',  ( -6.932735513423968321, 60.14768628210144641, -10.69584247140445221 ) ) ;
#23067=ORIENTED_EDGE ( 'NONE', *, *, #24913, .F. ) ;
#23071=CARTESIAN_POINT ( 'NONE',  ( 5.770363421894130873, 46.16481371789854649, -14.38691631536193860 ) ) ;
#23078=CARTESIAN_POINT ( 'NONE',  ( -3.796722387233185003, 26.61481371789854933, -8.710071997420207879 ) ) ;
#23084=CARTESIAN_POINT ( 'NONE',  ( 6.092822981423662299, 123.2148137178985792, 14.25334919248795096 ) ) ;
#23087=CARTESIAN_POINT ( 'NONE',  ( 10.49813415415989581, 54.97268628210144925, 7.228626920339068285 ) ) ;
#23094=CARTESIAN_POINT ( 'NONE',  ( -0.1745138560725182642, 74.81018628210145494, 9.500000000000005329 ) ) ;
#23098=CARTESIAN_POINT ( 'NONE',  ( 10.69584247140445221, 99.24768628210146915, -6.932735513423970097 ) ) ;
#23110=CARTESIAN_POINT ( 'NONE',  ( 4.622313124798831829, 128.9648137178985507, -11.61527771782809282 ) ) ;
#23112=CARTESIAN_POINT ( 'NONE',  ( 12.50000000000000355, 127.7101862821014606, 0.1745138560725507937 ) ) ;
#23119=CARTESIAN_POINT ( 'NONE',  ( -15.46528703574811736, 98.20231371789854791, 3.257655550456946436 ) ) ;
#23123=CARTESIAN_POINT ( 'NONE',  ( -6.840914352311947333, 72.03981371789855359, -6.594114490232462877 ) ) ;
#23126=CARTESIAN_POINT ( 'NONE',  ( -8.715434833792127023, 51.33981371789855785, 8.962234695871568846 ) ) ;
#23130=CARTESIAN_POINT ( 'NONE',  ( -11.48171059495397373, 96.08518628210146062, -4.944772684328680334 ) ) ;
#23136=CARTESIAN_POINT ( 'NONE',  ( 11.08355503943142750, 108.1601862821014635, -10.83675517735155225 ) ) ;
#23137=CARTESIAN_POINT ( 'NONE',  ( -12.46528703574805874, 12.99768628210143362, -2.660918448318280838 ) ) ;
#23140=CARTESIAN_POINT ( 'NONE',  ( 8.710071997420127943, 137.4851862821014379, 3.796722387233375073 ) ) ;
#23145=CARTESIAN_POINT ( 'NONE',  ( 9.500000000000005329, 63.31018628210144783, 0.1745138560725188748 ) ) ;
#23153=CARTESIAN_POINT ( 'NONE',  ( -5.529263428287297444, 35.52731371789855075, -7.954856959092311719 ) ) ;
#23158=CARTESIAN_POINT ( 'NONE',  ( -12.46528703574811558, 52.20231371789854791, 2.660918448318004170 ) ) ;
#23161=CARTESIAN_POINT ( 'NONE',  ( 2.660918448318002838, 13.10231371789855004, 12.46528703574811558 ) ) ;
#23175=CARTESIAN_POINT ( 'NONE',  ( -15.53471296425188442, 25.17731371789854933, -2.908627838312459080 ) ) ;
#23178=CARTESIAN_POINT ( 'NONE',  ( 0.1745138560725515708, 15.01018628210143468, -12.50000000000000355 ) ) ;
#23179=CARTESIAN_POINT ( 'NONE',  ( 2.311890736173175753, 46.92268628210145209, 12.53471296425194836 ) ) ;
#23191=CARTESIAN_POINT ( 'NONE',  ( -8.843639120294245259, 99.06481371789857349, -3.474262827703533230 ) ) ;
#23198=CARTESIAN_POINT ( 'NONE',  ( -4.622313124798826500, 96.76481371789854791, 11.61527771782809637 ) ) ;
#23202=CARTESIAN_POINT ( 'NONE',  ( 10.69584247140429589, 67.15231371789855075, 6.932735513424201024 ) ) ;
#23210=CARTESIAN_POINT ( 'NONE',  ( -4.944772684328673229, 38.58518628210144641, 11.48171059495397728 ) ) ;
#23217=CARTESIAN_POINT ( 'NONE',  ( 11.61527771782809637, 112.8648137178985564, 4.622313124798827388 ) ) ;
#23222=CARTESIAN_POINT ( 'NONE',  ( -5.770363421894122880, 78.36481371789855643, 14.38691631536194393 ) ) ;
#23226=CARTESIAN_POINT ( 'NONE',  ( -11.48171059495397373, 105.2851862821014493, -4.944772684328680334 ) ) ;
#23227=CARTESIAN_POINT ( 'NONE',  ( -8.927990412390661490, 38.87268628210144072, 13.04141134922759804 ) ) ;
#23230=CARTESIAN_POINT ( 'NONE',  ( -8.632099005475501130, 69.34768628210143504, -13.23911966647218996 ) ) ;
#23236=CARTESIAN_POINT ( 'NONE',  ( 6.932735513423970097, 37.14768628210143930, 10.69584247140445044 ) ) ;
#23239=CARTESIAN_POINT ( 'NONE',  ( -5.529263428287477744, 11.27268628210142865, 7.954856959092191815 ) ) ;
#23252=CARTESIAN_POINT ( 'NONE',  ( -11.48171059495397373, 68.48518628210145209, -4.944772684328680334 ) ) ;
#23259=CARTESIAN_POINT ( 'NONE',  ( 3.257655550456945548, 40.70231371789854791, 15.46528703574811736 ) ) ;
#23265=CARTESIAN_POINT ( 'NONE',  ( 9.500000000000005329, 29.48981371789855288, -0.1745138560723090149 ) ) ;
#23271=CARTESIAN_POINT ( 'NONE',  ( -14.38691631536193860, 126.6648137178985820, -5.770363421894132649 ) ) ;
#23274=CARTESIAN_POINT ( 'NONE',  ( 12.46528703574805874, 45.19768628210143646, 2.660918448318279950 ) ) ;
#23282=CARTESIAN_POINT ( 'NONE',  ( -8.152565276336710909, 57.84768628210144925, 5.233372021372435512 ) ) ;
#23285=CARTESIAN_POINT ( 'NONE',  ( -11.61527771782819940, 85.73518628210143788, 4.622313124798574258 ) ) ;
#23297=CARTESIAN_POINT ( 'NONE',  ( -2.660918448318004614, 128.1023137178985678, -12.46528703574811558 ) ) ;
#23298=CARTESIAN_POINT ( 'NONE',  ( 6.932735513423970097, 119.9476862821014578, 10.69584247140445044 ) ) ;
#23304=CARTESIAN_POINT ( 'NONE',  ( 15.53471296425188797, 103.3773137178985451, 2.908627838312457747 ) ) ;
#23308=CARTESIAN_POINT ( 'NONE',  ( -0.1745138560723084320, 82.38981371789856212, -9.500000000000005329 ) ) ;
#23311=CARTESIAN_POINT ( 'NONE',  ( 2.311890736173452865, 45.87731371789854506, -12.53471296425189152 ) ) ;
#23313=CARTESIAN_POINT ( 'NONE',  ( -11.61527771782819940, 94.93518628210145494, 4.622313124798574258 ) ) ;
#23317=CARTESIAN_POINT ( 'NONE',  ( 8.632099005475504683, 101.5476862821014663, 13.23911966647218996 ) ) ;
#23318=CARTESIAN_POINT ( 'NONE',  ( -4.944772684328673229, 20.18518628210144783, 11.48171059495397728 ) ) ;
#23321=CARTESIAN_POINT ( 'NONE',  ( 7.954856959092191815, 128.5726862821014436, 5.529263428287477744 ) ) ;
#23326=CARTESIAN_POINT ( 'NONE',  ( 7.954856959092191815, 54.97268628210144215, 5.529263428287477744 ) ) ;
#23334=CARTESIAN_POINT ( 'NONE',  ( -0.1745138560723084320, 45.58981371789855785, -9.500000000000005329 ) ) ;
#23339=CARTESIAN_POINT ( 'NONE',  ( 0.1745138560722779009, 50.18981371789854506, 12.50000000000000355 ) ) ;
#23342=CARTESIAN_POINT ( 'NONE',  ( -2.311890736173448424, 13.67731371789854400, 12.53471296425189330 ) ) ;
#23357=CARTESIAN_POINT ( 'NONE',  ( -14.25334919248795096, 15.11481371789854933, 6.092822981423662299 ) ) ;
#23359=CARTESIAN_POINT ( 'NONE',  ( 3.796722387233379514, 135.1851862821014549, -8.710071997420127943 ) ) ;
#23361=CARTESIAN_POINT ( 'NONE',  ( -4.622313124798576922, 51.23518628210143788, -11.61527771782819762 ) ) ;
#23367=CARTESIAN_POINT ( 'NONE',  ( 5.529263428287477744, 25.07268628210145067, -7.954856959092191815 ) ) ;
#23375=CARTESIAN_POINT ( 'NONE',  ( -8.710071997420207879, 88.71481371789855075, 3.796722387233182339 ) ) ;
#23380=CARTESIAN_POINT ( 'NONE',  ( -8.715434833792127023, 97.33981371789855075, 8.962234695871568846 ) ) ;
#23384=CARTESIAN_POINT ( 'NONE',  ( -10.69584247140429412, 71.75231371789855928, -6.932735513424201024 ) ) ;
#23394=CARTESIAN_POINT ( 'NONE',  ( 10.49813415415989581, 45.77268628210144641, 7.228626920339068285 ) ) ;
#23399=CARTESIAN_POINT ( 'NONE',  ( 4.622313124798831829, 101.3648137178985564, -11.61527771782809282 ) ) ;
#23404=CARTESIAN_POINT ( 'NONE',  ( 15.53471296425188797, 75.77731371789855075, 2.908627838312457747 ) ) ;
#23408=CARTESIAN_POINT ( 'NONE',  ( 10.49813415415989581, 100.9726862821014635, 7.228626920339068285 ) ) ;
#23409=CARTESIAN_POINT ( 'NONE',  ( -14.25334919248782306, 50.08518628210143930, -6.092822981423979378 ) ) ;
#23412=CARTESIAN_POINT ( 'NONE',  ( 13.04141134922759804, 73.37268628210144072, 8.927990412390657937 ) ) ;
#23418=CARTESIAN_POINT ( 'NONE',  ( -11.48171059495397373, 40.88518628210144357, -4.944772684328680334 ) ) ;
#23421=CARTESIAN_POINT ( 'NONE',  ( 3.474262827703335166, 9.835186282101449962, 8.843639120294326972 ) ) ;
#23431=CARTESIAN_POINT ( 'NONE',  ( 2.660918448318279950, 70.49768628210145494, -12.46528703574805874 ) ) ;
#23438=CARTESIAN_POINT ( 'NONE',  ( -11.08355503943118592, 44.43981371789855928, -10.83675517735179383 ) ) ;
#23445=CARTESIAN_POINT ( 'NONE',  ( -9.534712964251895073, 25.17731371789854933, -1.715153634034446428 ) ) ;
#23451=CARTESIAN_POINT ( 'NONE',  ( 2.908627838312458636, 128.6773137178985280, -15.53471296425188442 ) ) ;
#23454=CARTESIAN_POINT ( 'NONE',  ( 8.962234695871762469, 52.96018628210144641, -8.715434833791931624 ) ) ;
#23462=CARTESIAN_POINT ( 'NONE',  ( -6.840914352312096547, 57.56018628210145494, 6.594114490232313663 ) ) ;
#23465=CARTESIAN_POINT ( 'NONE',  ( -11.48171059495397373, 96.08518628210146062, -4.944772684328680334 ) ) ;
#23477=CARTESIAN_POINT ( 'NONE',  ( -0.1745138560722763466, 109.9898137178985706, -12.50000000000000355 ) ) ;
#23478=CARTESIAN_POINT ( 'NONE',  ( -6.932735513423968321, 115.3476862821014635, -10.69584247140445221 ) ) ;
#23484=CARTESIAN_POINT ( 'NONE',  ( 11.08355503943118769, 85.83981371789856496, 10.83675517735179028 ) ) ;
#23489=CARTESIAN_POINT ( 'NONE',  ( -5.529263428287297444, 72.32731371789854791, -7.954856959092311719 ) ) ;
#23494=CARTESIAN_POINT ( 'NONE',  ( -8.962234695871565293, 44.43981371789855217, -8.715434833792128799 ) ) ;
#23496=CARTESIAN_POINT ( 'NONE',  ( -4.944772684328673229, 102.9851862821014663, 11.48171059495397728 ) ) ;
#23503=CARTESIAN_POINT ( 'NONE',  ( -3.257655550457281723, 75.09768628210143504, 15.46528703574804986 ) ) ;
#23505=CARTESIAN_POINT ( 'NONE',  ( -6.932735513423968321, 4.947686282101432020, -10.69584247140445221 ) ) ;
#23507=CARTESIAN_POINT ( 'NONE',  ( 5.233372021372432847, 119.9476862821014294, 8.152565276336710909 ) ) ;
#23510=CARTESIAN_POINT ( 'NONE',  ( -3.257655550457281723, 19.89768628210143930, 15.46528703574804986 ) ) ;
#23515=CARTESIAN_POINT ( 'NONE',  ( 6.594114490232313663, 36.86018628210144499, 6.840914352312096547 ) ) ;
#23522=CARTESIAN_POINT ( 'NONE',  ( -0.1745138560723084320, 36.38981371789855501, -9.500000000000005329 ) ) ;
#23527=CARTESIAN_POINT ( 'NONE',  ( -7.228626920338836470, 44.72731371789855359, -10.49813415416005213 ) ) ;
#23529=CARTESIAN_POINT ( 'NONE',  ( 11.48171059495408208, 10.51481371789855856, -4.944772684328420986 ) ) ;
#23547=CARTESIAN_POINT ( 'NONE',  ( 3.257655550456945548, 13.10231371789855181, 15.46528703574811736 ) ) ;
#23550=CARTESIAN_POINT ( 'NONE',  ( -8.710071997420127943, 132.8851862821014436, -3.796722387233380402 ) ) ;
#23552=CARTESIAN_POINT ( 'NONE',  ( 7.228626920339068285, 25.07268628210144712, -10.49813415415989581 ) ) ;
#23557=CARTESIAN_POINT ( 'NONE',  ( -5.233372021372430183, 23.34768628210144570, -8.152565276336710909 ) ) ;
#23564=CARTESIAN_POINT ( 'NONE',  ( 9.465287035748106703, 93.60231371789855359, -2.064181346179063237 ) ) ;
#23569=CARTESIAN_POINT ( 'NONE',  ( -12.46528703574811558, 107.4023137178985650, 2.660918448318004170 ) ) ;
#23573=CARTESIAN_POINT ( 'NONE',  ( 12.50000000000000355, 75.48981371789855643, -0.1745138560722771515 ) ) ;
#23581=CARTESIAN_POINT ( 'NONE',  ( -12.53471296425194836, 40.02268628210143930, 2.311890736173176641 ) ) ;
#23582=EDGE_CURVE ( 'NONE', #33833, #1210, #11900, .T. ) ;
#23587=CARTESIAN_POINT ( 'NONE',  ( 2.311890736173452865, 101.0773137178985621, -12.53471296425189152 ) ) ;
#23592=CARTESIAN_POINT ( 'NONE',  ( -15.53471296425188442, 71.17731371789855643, -2.908627838312459080 ) ) ;
#23595=CARTESIAN_POINT ( 'NONE',  ( -6.422845572874366304, 142.9999999999996305, 10.72508787064079172 ) ) ;
#23596=CARTESIAN_POINT ( 'NONE',  ( -12.46528703574805697, 95.79768628210143788, -2.660918448318280838 ) ) ;
#23597=CARTESIAN_POINT ( 'NONE',  ( -2.908627838312119351, 51.52268628210144641, -15.53471296425195369 ) ) ;
#23599=CARTESIAN_POINT ( 'NONE',  ( 8.632099005475504683, 64.74768628210144072, 13.23911966647218996 ) ) ;
#23605=CARTESIAN_POINT ( 'NONE',  ( 7.228626920339068285, 34.27268628210144641, -10.49813415415989581 ) ) ;
#23606=CARTESIAN_POINT ( 'NONE',  ( -6.594114490232312775, 4.660186282101435928, -6.840914352312096547 ) ) ;
#23620=CARTESIAN_POINT ( 'NONE',  ( 4.944772684328679446, 52.38518628210145067, -11.48171059495397373 ) ) ;
#23629=CARTESIAN_POINT ( 'NONE',  ( -8.962234695871760692, 94.36018628210145209, 8.715434833791933400 ) ) ;
#23630=CARTESIAN_POINT ( 'NONE',  ( -0.1745138560722442889, 17.98981371789853867, -15.50000000000000533 ) ) ;
#23637=CARTESIAN_POINT ( 'NONE',  ( -5.233372021372612259, 14.25231371789853618, 8.152565276336593669 ) ) ;
#23644=CARTESIAN_POINT ( 'NONE',  ( 8.632099005475788900, 138.4523137178985621, -13.23911966647199812 ) ) ;
#23647=CARTESIAN_POINT ( 'NONE',  ( -6.932735513423968321, 50.94768628210144357, -10.69584247140445221 ) ) ;
#23653=CARTESIAN_POINT ( 'NONE',  ( -8.843639120294326972, 67.33518628210143220, 3.474262827703335166 ) ) ;
#23656=CARTESIAN_POINT ( 'NONE',  ( 11.48171059495397728, 91.48518628210145209, 4.944772684328674117 ) ) ;
#23668=CARTESIAN_POINT ( 'NONE',  ( -12.50000000000000355, 107.6898137178985735, 0.1745138560722786503 ) ) ;
#23669=CARTESIAN_POINT ( 'NONE',  ( -10.69584247140444866, 131.4476862821014720, 6.932735513423972762 ) ) ;
#23674=CARTESIAN_POINT ( 'NONE',  ( -6.092822981423666739, 72.61481371789855643, -14.25334919248795096 ) ) ;
#23677=CARTESIAN_POINT ( 'NONE',  ( -9.534712964251941258, 95.22268628210143504, 1.715153634034234154 ) ) ;
#23679=CARTESIAN_POINT ( 'NONE',  ( 7.954856959092311719, 83.82731371789856212, -5.529263428287300108 ) ) ;
#23683=CARTESIAN_POINT ( 'NONE',  ( 10.69584247140429589, 39.55231371789855643, 6.932735513424201024 ) ) ;
#23685=CARTESIAN_POINT ( 'NONE',  ( -2.311890736173176641, 106.7226862821014635, -12.53471296425194836 ) ) ;
#23691=CARTESIAN_POINT ( 'NONE',  ( -2.908627838312119351, 88.32268628210142936, -15.53471296425195369 ) ) ;
#23696=CARTESIAN_POINT ( 'NONE',  ( 7.954856959092191815, 119.3726862821014265, 5.529263428287477744 ) ) ;
#23699=CARTESIAN_POINT ( 'NONE',  ( 8.632099005475504683, 9.547686282101452093, 13.23911966647218996 ) ) ;
#23711=CARTESIAN_POINT ( 'NONE',  ( -7.954856959092309943, 24.02731371789854364, 5.529263428287300108 ) ) ;
#23715=CARTESIAN_POINT ( 'NONE',  ( 2.660918448318003282, 49.90231371789855075, 12.46528703574811558 ) ) ;
#23718=CARTESIAN_POINT ( 'NONE',  ( -11.61527771782809282, 7.064813717898549505, -4.622313124798832717 ) ) ;
#23735=CARTESIAN_POINT ( 'NONE',  ( 8.632099005475788900, 9.652313717898541867, -13.23911966647199812 ) ) ;
#23738=CARTESIAN_POINT ( 'NONE',  ( 8.843639120294328748, 136.3351862821014606, -3.474262827703334722 ) ) ;
#23740=CARTESIAN_POINT ( 'NONE',  ( 0.1745138560725515708, 33.41018628210144925, -12.50000000000000355 ) ) ;
#23744=CARTESIAN_POINT ( 'NONE',  ( 5.770363421893814682, 129.4351862821014549, 14.38691631536207183 ) ) ;
#23746=CARTESIAN_POINT ( 'NONE',  ( 3.796722387233182339, 141.6148137178985849, 8.710071997420207879 ) ) ;
#23753=CARTESIAN_POINT ( 'NONE',  ( 8.843639120294245259, 76.06481371789855928, 3.474262827703527901 ) ) ;
#23757=CARTESIAN_POINT ( 'NONE',  ( -4.944772684328424539, 91.01481371789856212, -11.48171059495408031 ) ) ;
#23761=CARTESIAN_POINT ( 'NONE',  ( 7.228626920338837358, 67.72731371789856780, 10.49813415416005036 ) ) ;
#23769=CARTESIAN_POINT ( 'NONE',  ( 4.944772684328679446, 33.98518628210143788, -11.48171059495397373 ) ) ;
#23776=CARTESIAN_POINT ( 'NONE',  ( 12.53471296425189330, 94.17731371789857064, 2.311890736173451977 ) ) ;
#23782=CARTESIAN_POINT ( 'NONE',  ( 11.08355503943118769, 58.23981371789854222, 10.83675517735179028 ) ) ;
#23785=CARTESIAN_POINT ( 'NONE',  ( 8.962234695871762469, 89.76018628210144357, -8.715434833791931624 ) ) ;
#23786=CARTESIAN_POINT ( 'NONE',  ( 0.1745138560725837118, 42.61018628210144499, -15.50000000000000533 ) ) ;
#23789=CARTESIAN_POINT ( 'NONE',  ( -14.38691631536207183, 48.93518628210144072, 5.770363421893814682 ) ) ;
#23795=CARTESIAN_POINT ( 'NONE',  ( -12.50000000000000355, 21.91018628210143859, -0.1745138560725492671 ) ) ;
#23798=CARTESIAN_POINT ( 'NONE',  ( 6.840914352311949109, 141.0398137178985678, 6.594114490232462877 ) ) ;
#23808=CARTESIAN_POINT ( 'NONE',  ( -8.715434833791929847, 41.46018628210144641, -8.962234695871762469 ) ) ;
#23816=CARTESIAN_POINT ( 'NONE',  ( 12.46528703574805874, 91.19768628210145778, 2.660918448318279950 ) ) ;
#23817=CARTESIAN_POINT ( 'NONE',  ( -14.25334919248795096, 15.11481371789854933, 6.092822981423662299 ) ) ;
#23823=CARTESIAN_POINT ( 'NONE',  ( -3.796722387233185003, 8.214813717898532985, -8.710071997420207879 ) ) ;
#23830=CARTESIAN_POINT ( 'NONE',  ( -15.50000000000000533, 135.2898137178985394, 0.1745138560722471477 ) ) ;
#23834=CARTESIAN_POINT ( 'NONE',  ( -2.311890736173176641, 42.32268628210145067, -12.53471296425194836 ) ) ;
#23838=CARTESIAN_POINT ( 'NONE',  ( 10.83675517735155225, 110.4601862821014606, 11.08355503943142573 ) ) ;
#23843=CARTESIAN_POINT ( 'NONE',  ( -5.529263428287477744, 66.47268628210146346, 7.954856959092191815 ) ) ;
#23848=CARTESIAN_POINT ( 'NONE',  ( -2.660918448318275509, 102.6976862821014720, 12.46528703574805874 ) ) ;
#23860=CARTESIAN_POINT ( 'NONE',  ( 8.715434833792128799, 111.1398137178985621, -8.962234695871567070 ) ) ;
#23861=CARTESIAN_POINT ( 'NONE',  ( 12.53471296425194659, 109.0226862821014606, -2.311890736173178418 ) ) ;
#23865=CARTESIAN_POINT ( 'NONE',  ( -15.53471296425188442, 80.37731371789853085, -2.908627838312459080 ) ) ;
#23868=CARTESIAN_POINT ( 'NONE',  ( 5.233372021372432847, 92.34768628210142083, 8.152565276336710909 ) ) ;
#23872=CARTESIAN_POINT ( 'NONE',  ( -9.534712964251895073, 71.17731371789855643, -1.715153634034446428 ) ) ;
#23875=CARTESIAN_POINT ( 'NONE',  ( -5.529263428287297444, 118.3273137178985763, -7.954856959092311719 ) ) ;
#23877=CARTESIAN_POINT ( 'NONE',  ( 7.228626920338837358, 49.32731371789855501, 10.49813415416005036 ) ) ;
#23879=CARTESIAN_POINT ( 'NONE',  ( 10.69584247140445221, 99.24768628210146915, -6.932735513423970097 ) ) ;
#23882=CARTESIAN_POINT ( 'NONE',  ( -6.932735513423968321, 133.7476862821014549, -10.69584247140445221 ) ) ;
#23884=CARTESIAN_POINT ( 'NONE',  ( 3.257655550457285720, 88.89768628210146062, -15.46528703574804986 ) ) ;
#23889=CARTESIAN_POINT ( 'NONE',  ( 9.465287035748067623, 109.5976862821014493, 2.064181346179272847 ) ) ;
#23891=CARTESIAN_POINT ( 'NONE',  ( -10.83675517735155047, 13.86018628210145032, -11.08355503943142750 ) ) ;
#23902=CARTESIAN_POINT ( 'NONE',  ( -3.796722387233185003, 26.61481371789854933, -8.710071997420207879 ) ) ;
#23907=CARTESIAN_POINT ( 'NONE',  ( 8.962234695871567070, 21.43981371789854862, 8.715434833792127023 ) ) ;
#23909=CARTESIAN_POINT ( 'NONE',  ( 15.50000000000000533, 139.8898137178985621, -0.1745138560722452326 ) ) ;
#23927=CARTESIAN_POINT ( 'NONE',  ( -10.83675517735155047, 133.4601862821014606, -11.08355503943142750 ) ) ;
#23929=CARTESIAN_POINT ( 'NONE',  ( 3.796722387233379514, 125.9851862821014521, -8.710071997420127943 ) ) ;
#23931=CARTESIAN_POINT ( 'NONE',  ( 10.49813415415989581, 36.57268628210145067, 7.228626920339068285 ) ) ;
#23935=CARTESIAN_POINT ( 'NONE',  ( -3.257655550457281723, 121.0976862821014635, 15.46528703574804986 ) ) ;
#23937=CARTESIAN_POINT ( 'NONE',  ( -9.500000000000005329, 3.510186282101451560, -0.1745138560725176813 ) ) ;
#23943=CARTESIAN_POINT ( 'NONE',  ( -9.465287035748106703, 70.60231371789853938, 2.064181346179061460 ) ) ;
#23948=CARTESIAN_POINT ( 'NONE',  ( 7.228626920338837358, 86.12731371789855928, 10.49813415416005036 ) ) ;
#23952=CARTESIAN_POINT ( 'NONE',  ( -12.46528703574811558, 52.20231371789855501, 2.660918448318003726 ) ) ;
#23959=CARTESIAN_POINT ( 'NONE',  ( -12.46528703574805697, 31.39768628210144641, -2.660918448318280838 ) ) ;
#23966=CARTESIAN_POINT ( 'NONE',  ( 11.48171059495408208, 93.31481371789855928, -4.944772684328420986 ) ) ;
#23972=CARTESIAN_POINT ( 'NONE',  ( 5.770363421894130873, 64.56481371789854506, -14.38691631536193860 ) ) ;
#23975=CARTESIAN_POINT ( 'NONE',  ( -12.53471296425194836, 86.02268628210146062, 2.311890736173176641 ) ) ;
#23976=CARTESIAN_POINT ( 'NONE',  ( 8.927990412390657937, 25.07268628210145067, -13.04141134922759804 ) ) ;
#23980=CARTESIAN_POINT ( 'NONE',  ( -3.257655550457281723, 47.49768628210145494, 15.46528703574804986 ) ) ;
#23987=CARTESIAN_POINT ( 'NONE',  ( -10.49813415415989581, 13.57268628210145600, -7.228626920339068285 ) ) ;
#23989=CARTESIAN_POINT ( 'NONE',  ( -1.715153634034442431, 133.2773137178985507, 9.534712964251900402 ) ) ;
#23998=CARTESIAN_POINT ( 'NONE',  ( -2.660918448318275509, 47.49768628210144783, 12.46528703574805874 ) ) ;
#24006=CARTESIAN_POINT ( 'NONE',  ( 0.1745138560725515708, 97.81018628210144072, -12.50000000000000355 ) ) ;
#24007=CARTESIAN_POINT ( 'NONE',  ( 13.23911966647199812, 21.15231371789855430, 8.632099005475788900 ) ) ;
#24014=CARTESIAN_POINT ( 'NONE',  ( 4.622313124798831829, 138.1648137178985678, -11.61527771782809282 ) ) ;
#24020=CARTESIAN_POINT ( 'NONE',  ( -15.53471296425188442, 117.1773137178985706, -2.908627838312459080 ) ) ;
#24024=CARTESIAN_POINT ( 'NONE',  ( -0.1745138560725500443, 28.81018628210144072, 12.50000000000000355 ) ) ;
#24028=CARTESIAN_POINT ( 'NONE',  ( 14.25334919248782661, 100.6851862821014834, 6.092822981423971385 ) ) ;
#24031=CARTESIAN_POINT ( 'NONE',  ( 2.064181346179272847, 52.09768628210144925, -9.465287035748065847 ) ) ;
#24034=CARTESIAN_POINT ( 'NONE',  ( 4.944772684328679446, 79.98518628210145209, -11.48171059495397373 ) ) ;
#24046=CARTESIAN_POINT ( 'NONE',  ( -8.962234695871565293, 99.63981371789856212, -8.715434833792128799 ) ) ;
#24047=CARTESIAN_POINT ( 'NONE',  ( 7.228626920339069173, 107.8726862821014549, -10.49813415415989404 ) ) ;
#24052=CARTESIAN_POINT ( 'NONE',  ( 15.46528703574811736, 75.20231371789854791, -3.257655550456947768 ) ) ;
#24055=CARTESIAN_POINT ( 'NONE',  ( 5.529263428287477744, 107.8726862821014549, -7.954856959092191815 ) ) ;
#24058=CARTESIAN_POINT ( 'NONE',  ( 1.715153634034445762, 64.27731371789853654, -9.534712964251895073 ) ) ;
#24060=CARTESIAN_POINT ( 'NONE',  ( -1.715153634034442431, 114.8773137178985735, 9.534712964251900402 ) ) ;
#24062=CARTESIAN_POINT ( 'NONE',  ( -12.53471296425189152, 34.37731371789855217, -2.311890736173453753 ) ) ;
#24065=CARTESIAN_POINT ( 'NONE',  ( 11.48171059495397728, 82.28518628210146346, 4.944772684328674117 ) ) ;
#24069=CARTESIAN_POINT ( 'NONE',  ( 13.23911966647218996, 90.04768628210145209, -8.632099005475504683 ) ) ;
#24074=CARTESIAN_POINT ( 'NONE',  ( 0.1745138560725194299, 107.0101862821014578, -9.500000000000005329 ) ) ;
#24076=CARTESIAN_POINT ( 'NONE',  ( 8.715434833791931624, 128.8601862821014663, 8.962234695871760692 ) ) ;
#24087=CARTESIAN_POINT ( 'NONE',  ( -0.1745138560723084320, 17.98981371789853867, -9.500000000000005329 ) ) ;
#24092=CARTESIAN_POINT ( 'NONE',  ( 2.660918448318003282, 31.50231371789854862, 12.46528703574811558 ) ) ;
#24094=CARTESIAN_POINT ( 'NONE',  ( 0.1745138560722461762, 132.9898137178985564, 15.50000000000000533 ) ) ;
#24103=CARTESIAN_POINT ( 'NONE',  ( -10.49813415415989581, 133.1726862821014663, -7.228626920339068285 ) ) ;
#24116=CARTESIAN_POINT ( 'NONE',  ( -8.927990412390661490, 130.8726862821014834, 13.04141134922759804 ) ) ;
#24118=CARTESIAN_POINT ( 'NONE',  ( -5.529263428287477744, 130.8726862821014834, 7.954856959092191815 ) ) ;
#24120=CARTESIAN_POINT ( 'NONE',  ( -12.53471296425194836, 21.62268628210144072, 2.311890736173176641 ) ) ;
#24124=CARTESIAN_POINT ( 'NONE',  ( 10.83675517735155225, 128.8601862821014663, 11.08355503943142573 ) ) ;
#24126=CARTESIAN_POINT ( 'NONE',  ( -1.715153634034442431, 142.4773137178985678, 9.534712964251900402 ) ) ;
#24133=CARTESIAN_POINT ( 'NONE',  ( -7.954856959092309943, 70.02731371789855075, 5.529263428287300108 ) ) ;
#24138=CARTESIAN_POINT ( 'NONE',  ( -7.228626920338836470, 72.32731371789854791, -10.49813415416005213 ) ) ;
#24142=CARTESIAN_POINT ( 'NONE',  ( -12.46528703574811558, 43.00231371789854506, 2.660918448318003726 ) ) ;
#24146=CARTESIAN_POINT ( 'NONE',  ( 10.49813415415989581, 18.17268628210144854, 7.228626920339068285 ) ) ;
#24150=CARTESIAN_POINT ( 'NONE',  ( 12.53471296425189330, 84.97731371789855359, 2.311890736173451977 ) ) ;
#24155=CARTESIAN_POINT ( 'NONE',  ( -14.25334919248795096, 61.11481371789854933, 6.092822981423662299 ) ) ;
#24158=CARTESIAN_POINT ( 'NONE',  ( -4.944772684328673229, 84.58518628210146062, 11.48171059495397728 ) ) ;
#24159=CARTESIAN_POINT ( 'NONE',  ( -11.08355503943142573, 20.76018628210144001, 10.83675517735155402 ) ) ;
#24163=CARTESIAN_POINT ( 'NONE',  ( 15.50000000000000533, 44.91018628210144215, 0.1745138560725827404 ) ) ;
#24170=CARTESIAN_POINT ( 'NONE',  ( -10.69584247140444866, 21.04768628210144854, 6.932735513423972762 ) ) ;
#24172=CARTESIAN_POINT ( 'NONE',  ( -7.954856959092309943, 125.2273137178985394, 5.529263428287300108 ) ) ;
#24177=CARTESIAN_POINT ( 'NONE',  ( 10.69584247140429589, 131.5523137178985849, 6.932735513424201024 ) ) ;
#24182=CARTESIAN_POINT ( 'NONE',  ( -11.61527771782819940, 58.13518628210144357, 4.622313124798574258 ) ) ;
#24190=CARTESIAN_POINT ( 'NONE',  ( -6.932735513423968321, 78.54768628210146630, -10.69584247140445221 ) ) ;
#24191=CARTESIAN_POINT ( 'NONE',  ( -11.08355503943118592, 16.83981371789855430, -10.83675517735179383 ) ) ;
#24198=CARTESIAN_POINT ( 'NONE',  ( 11.61527771782809637, 140.4648137178985792, 4.622313124798827388 ) ) ;
#24204=CARTESIAN_POINT ( 'NONE',  ( -2.908627838312453306, 105.6773137178985706, 15.53471296425188797 ) ) ;
#24207=CARTESIAN_POINT ( 'NONE',  ( 8.962234695871762469, 34.56018628210144783, -8.715434833791931624 ) ) ;
#24212=CARTESIAN_POINT ( 'NONE',  ( 5.770363421893814682, 101.8351862821014606, 14.38691631536207183 ) ) ;
#24215=CARTESIAN_POINT ( 'NONE',  ( -9.500000000000005329, 40.31018628210145494, -0.1745138560725176813 ) ) ;
#24219=CARTESIAN_POINT ( 'NONE',  ( 10.69584247140445221, 71.64768628210146062, -6.932735513423970097 ) ) ;
#24222=CARTESIAN_POINT ( 'NONE',  ( -8.710071997420127943, 40.88518628210145067, -3.796722387233380402 ) ) ;
#24233=CARTESIAN_POINT ( 'NONE',  ( -2.311890736173448424, 105.6773137178985564, 12.53471296425189330 ) ) ;
#24234=CARTESIAN_POINT ( 'NONE',  ( 4.622313124798573369, 101.8351862821014464, 11.61527771782819940 ) ) ;
#24240=CARTESIAN_POINT ( 'NONE',  ( 10.83675517735179206, 83.53981371789856780, -11.08355503943118769 ) ) ;
#24244=CARTESIAN_POINT ( 'NONE',  ( -9.500000000000005329, 95.51018628210147199, -0.1745138560725176813 ) ) ;
#24247=CARTESIAN_POINT ( 'NONE',  ( -5.233372021372612259, 60.25231371789854506, 8.152565276336593669 ) ) ;
#24249=CARTESIAN_POINT ( 'NONE',  ( 6.840914352311949109, 113.4398137178985593, 6.594114490232462877 ) ) ;
#24251=CARTESIAN_POINT ( 'NONE',  ( 8.962234695871567070, 30.63981371789854791, 8.715434833792127023 ) ) ;
#24254=CARTESIAN_POINT ( 'NONE',  ( -11.48171059495397373, 86.88518628210145778, -4.944772684328680334 ) ) ;
#24263=CARTESIAN_POINT ( 'NONE',  ( -9.500000000000005329, 104.7101862821014606, -0.1745138560725176813 ) ) ;
#24265=CARTESIAN_POINT ( 'NONE',  ( 2.311890736173175753, 138.9226862821014663, 12.53471296425194836 ) ) ;
#24266=CARTESIAN_POINT ( 'NONE',  ( -6.804952097069882910, 143.0000000000000284, 9.842932490202064955 ) ) ;
#24277=CARTESIAN_POINT ( 'NONE',  ( -6.840914352311947333, 16.83981371789855430, -6.594114490232462877 ) ) ;
#24282=CARTESIAN_POINT ( 'NONE',  ( 11.48171059495408208, 28.91481371789854293, -4.944772684328420986 ) ) ;
#24284=CARTESIAN_POINT ( 'NONE',  ( -8.927990412390371944, 136.7273137178985110, -13.04141134922778988 ) ) ;
#24292=CARTESIAN_POINT ( 'NONE',  ( -2.660918448318275509, 130.2976862821014379, 12.46528703574805874 ) ) ;
#24299=CARTESIAN_POINT ( 'NONE',  ( 8.715434833791931624, 128.8601862821014663, 8.962234695871760692 ) ) ;
#24303=CARTESIAN_POINT ( 'NONE',  ( -15.50000000000000533, 141.5101862821014720, -0.1745138560725808530 ) ) ;
#24305=CARTESIAN_POINT ( 'NONE',  ( 6.840914352312096547, 117.3601862821014663, -6.594114490232313663 ) ) ;
#24308=CARTESIAN_POINT ( 'NONE',  ( 12.50000000000000355, 26.51018628210144357, 0.1745138560725507937 ) ) ;
#24312=CARTESIAN_POINT ( 'NONE',  ( -5.770363421893818234, 115.6351862821014436, -14.38691631536207005 ) ) ;
#24314=CARTESIAN_POINT ( 'NONE',  ( 3.474262827703335166, 9.835186282101449962, 8.843639120294326972 ) ) ;
#24322=CARTESIAN_POINT ( 'NONE',  ( 8.710071997420211432, 74.91481371789855359, -3.796722387233181895 ) ) ;
#24325=CARTESIAN_POINT ( 'NONE',  ( -8.962234695871565293, 72.03981371789855359, -8.715434833792128799 ) ) ;
#24329=CARTESIAN_POINT ( 'NONE',  ( 10.69584247140429589, 48.75231371789854506, 6.932735513424201024 ) ) ;
#24334=CARTESIAN_POINT ( 'NONE',  ( -12.46528703574805697, 12.99768628210143362, -2.660918448318280838 ) ) ;
#24340=CARTESIAN_POINT ( 'NONE',  ( 12.50000000000000355, 93.88981371789856212, -0.1745138560722771515 ) ) ;
#24345=CARTESIAN_POINT ( 'NONE',  ( 3.257655550456945548, 49.90231371789854364, 15.46528703574811736 ) ) ;
#24348=CARTESIAN_POINT ( 'NONE',  ( 10.69584247140445221, 80.84768628210144925, -6.932735513423970097 ) ) ;
#24349=CARTESIAN_POINT ( 'NONE',  ( -3.257655550457281723, 19.89768628210143930, 15.46528703574804986 ) ) ;
#24354=CARTESIAN_POINT ( 'NONE',  ( -0.1745138560725817967, 56.41018628210145636, 15.50000000000000533 ) ) ;
#24359=CARTESIAN_POINT ( 'NONE',  ( 11.61527771782819940, 25.93518628210143717, -4.622313124798573369 ) ) ;
#24361=CARTESIAN_POINT ( 'NONE',  ( 8.710071997420211432, 139.3148137178985451, -3.796722387233181895 ) ) ;
#24365=CARTESIAN_POINT ( 'NONE',  ( 8.715434833792128799, 129.5398137178985678, -8.962234695871567070 ) ) ;
#24371=CARTESIAN_POINT ( 'NONE',  ( 10.49813415415989581, 45.77268628210144641, 7.228626920339069173 ) ) ;
#24379=CARTESIAN_POINT ( 'NONE',  ( -12.53471296425194836, 76.82268628210145778, 2.311890736173176641 ) ) ;
#24380=CARTESIAN_POINT ( 'NONE',  ( 8.927990412390371944, 12.52731371789855963, 13.04141134922778811 ) ) ;
#24386=CARTESIAN_POINT ( 'NONE',  ( -7.228626920338836470, 136.7273137178985678, -10.49813415416005213 ) ) ;
#24391=CARTESIAN_POINT ( 'NONE',  ( -3.257655550456946880, 109.7023137178985479, -15.46528703574811736 ) ) ;
#24394=CARTESIAN_POINT ( 'NONE',  ( 10.69584247140445221, 34.84768628210143504, -6.932735513423970097 ) ) ;
#24398=CARTESIAN_POINT ( 'NONE',  ( -10.83675517735155047, 105.8601862821014379, -11.08355503943142750 ) ) ;
#24402=CARTESIAN_POINT ( 'NONE',  ( 1.715153634034233487, 37.72268628210143504, 9.534712964251941258 ) ) ;
#24406=CARTESIAN_POINT ( 'NONE',  ( -4.622313124798576922, 78.83518628210146062, -11.61527771782819762 ) ) ;
#24409=CARTESIAN_POINT ( 'NONE',  ( -8.152565276336710909, 48.64768628210144641, 5.233372021372435512 ) ) ;
#24421=CARTESIAN_POINT ( 'NONE',  ( -8.715434833792127023, 78.93981371789855928, 8.962234695871568846 ) ) ;
#24422=CARTESIAN_POINT ( 'NONE',  ( 10.69584247140445221, 108.4476862821014578, -6.932735513423970097 ) ) ;
#24427=CARTESIAN_POINT ( 'NONE',  ( 5.770363421894130873, 82.96481371789856496, -14.38691631536193860 ) ) ;
#24430=CARTESIAN_POINT ( 'NONE',  ( -3.474262827703337830, 97.23518628210146630, -8.843639120294326972 ) ) ;
#24432=CARTESIAN_POINT ( 'NONE',  ( -1.715153634034442431, 50.47731371789854649, 9.534712964251900402 ) ) ;
#24435=CARTESIAN_POINT ( 'NONE',  ( -2.064181346179062349, 109.7023137178985479, -9.465287035748106703 ) ) ;
#24437=CARTESIAN_POINT ( 'NONE',  ( -11.61527771782809282, 34.66481371789854649, -4.622313124798832717 ) ) ;
#24438=CARTESIAN_POINT ( 'NONE',  ( 11.61527771782819940, 81.13518628210145778, -4.622313124798573369 ) ) ;
#24445=DIRECTION ( 'NONE',  ( 1.045431693899523378E-14, 0.1163425707149433469, -0.9932091452657081376 ) ) ;
#24447=CARTESIAN_POINT ( 'NONE',  ( 3.796722387233379514, 89.18518628210145494, -8.710071997420127943 ) ) ;
#24448=CARTESIAN_POINT ( 'NONE',  ( 11.48171059495397728, 137.4851862821014663, 4.944772684328674117 ) ) ;
#24461=CARTESIAN_POINT ( 'NONE',  ( -8.152565276336593669, 25.75231371789854506, -5.233372021372610483 ) ) ;
#24468=CARTESIAN_POINT ( 'NONE',  ( -12.50000000000000355, 24.88981371789854435, 0.1745138560722786503 ) ) ;
#24470=CARTESIAN_POINT ( 'NONE',  ( -14.25334919248795096, 125.5148137178985763, 6.092822981423662299 ) ) ;
#24477=CARTESIAN_POINT ( 'NONE',  ( 6.932735513423970097, 129.1476862821014890, 10.69584247140445044 ) ) ;
#24484=CARTESIAN_POINT ( 'NONE',  ( -12.46528703574805697, 132.5976862821014777, -2.660918448318280838 ) ) ;
#24488=CARTESIAN_POINT ( 'NONE',  ( 6.092822981423978490, 135.1851862821014549, -14.25334919248782306 ) ) ;
#24491=CARTESIAN_POINT ( 'NONE',  ( 3.796722387233379514, 116.7851862821014635, -8.710071997420127943 ) ) ;
#24493=CARTESIAN_POINT ( 'NONE',  ( 11.48171059495397728, 8.685186282101437172, 4.944772684328674117 ) ) ;
#24498=CARTESIAN_POINT ( 'NONE',  ( -13.23911966647218463, 113.0476862821014663, 8.632099005475506459 ) ) ;
#24500=CARTESIAN_POINT ( 'NONE',  ( 8.843639120294245259, 140.4648137178985507, 3.474262827703527901 ) ) ;
#24505=CARTESIAN_POINT ( 'NONE',  ( 0.1745138560723095977, 68.58981371789855075, 9.500000000000005329 ) ) ;
#24508=CARTESIAN_POINT ( 'NONE',  ( 8.962234695871567070, 85.83981371789856496, 8.715434833792127023 ) ) ;
#24510=CARTESIAN_POINT ( 'NONE',  ( -7.145391844330089448, 143.0000000000000284, 10.79229366378071298 ) ) ;
#24512=CARTESIAN_POINT ( 'NONE',  ( -2.311890736173448424, 50.47731371789855359, 12.53471296425189330 ) ) ;
#24516=CARTESIAN_POINT ( 'NONE',  ( 4.622313124798573369, 19.03518628210144925, 11.61527771782819940 ) ) ;
#24520=CARTESIAN_POINT ( 'NONE',  ( 4.944772684328420986, 77.21481371789855075, 11.48171059495408208 ) ) ;
#24526=CARTESIAN_POINT ( 'NONE',  ( 14.25334919248795451, 56.51481371789856212, -6.092822981423661410 ) ) ;
#24529=CARTESIAN_POINT ( 'NONE',  ( -11.61527771782819940, 76.53518628210146346, 4.622313124798574258 ) ) ;
#24530=CARTESIAN_POINT ( 'NONE',  ( 0.1745138560725837118, 24.21018628210144996, -15.50000000000000533 ) ) ;
#24535=CARTESIAN_POINT ( 'NONE',  ( -6.092822981423970496, 56.98518628210145209, 14.25334919248782661 ) ) ;
#24540=CARTESIAN_POINT ( 'NONE',  ( -8.962234695871760692, 20.76018628210144001, 8.715434833791933400 ) ) ;
#24543=CARTESIAN_POINT ( 'NONE',  ( 6.594114490232462877, 129.5398137178985678, -6.840914352311949109 ) ) ;
#24547=CARTESIAN_POINT ( 'NONE',  ( -8.962234695871565293, 127.2398137178985564, -8.715434833792128799 ) ) ;
#24554=CARTESIAN_POINT ( 'NONE',  ( 12.46528703574805874, 35.99768628210144072, 2.660918448318279950 ) ) ;
#24562=CARTESIAN_POINT ( 'NONE',  ( -8.962234695871760692, 85.16018628210144925, 8.715434833791933400 ) ) ;
#24563=CARTESIAN_POINT ( 'NONE',  ( -15.46528703574804986, 132.5976862821014493, -3.257655550457287497 ) ) ;
#24567=CARTESIAN_POINT ( 'NONE',  ( 1.715153634034445762, 9.077313717898549683, -9.534712964251895073 ) ) ;
#24575=CARTESIAN_POINT ( 'NONE',  ( 15.46528703574811736, 121.2023137178985479, -3.257655550456947768 ) ) ;
#24579=CARTESIAN_POINT ( 'NONE',  ( 0.1745138560725515708, 134.6101862821014663, -12.50000000000000355 ) ) ;
#24582=CARTESIAN_POINT ( 'NONE',  ( 15.53471296425195369, 99.82268628210142936, -2.908627838312120684 ) ) ;
#24585=CARTESIAN_POINT ( 'NONE',  ( -3.474262827703337830, 42.03518628210144925, -8.843639120294326972 ) ) ;
#24589=CARTESIAN_POINT ( 'NONE',  ( 6.932735513423970097, 83.14768628210144641, 10.69584247140445044 ) ) ;
#24592=CARTESIAN_POINT ( 'NONE',  ( 6.840914352312096547, 43.76018628210144357, -6.594114490232313663 ) ) ;
#24602=STYLED_ITEM('',(#37542),#21172);
#24603=CARTESIAN_POINT ( 'NONE',  ( 2.660918448318002838, 77.50231371789855928, 12.46528703574811558 ) ) ;
#24604=CARTESIAN_POINT ( 'NONE',  ( -0.1745138560725500443, 84.01018628210145778, 12.50000000000000355 ) ) ;
#24609=CARTESIAN_POINT ( 'NONE',  ( -14.25334919248795096, 61.11481371789854933, 6.092822981423662299 ) ) ;
#24616=CARTESIAN_POINT ( 'NONE',  ( -9.465287035748106703, 61.40231371789855785, 2.064181346179061460 ) ) ;
#24618=CARTESIAN_POINT ( 'NONE',  ( -1.715153634034442431, 105.6773137178985706, 9.534712964251900402 ) ) ;
#24620=CARTESIAN_POINT ( 'NONE',  ( -10.69584247140429412, 25.75231371789854506, -6.932735513424201024 ) ) ;
#24621=CARTESIAN_POINT ( 'NONE',  ( 12.53471296425194836, 81.42268628210145209, -2.311890736173178418 ) ) ;
#24629=CARTESIAN_POINT ( 'NONE',  ( -1.715153634034234598, 88.32268628210142936, -9.534712964251941258 ) ) ;
#24631=CARTESIAN_POINT ( 'NONE',  ( -4.622313124798576922, 134.0351862821014493, -11.61527771782819762 ) ) ;
#24641=CARTESIAN_POINT ( 'NONE',  ( -6.932735513424201912, 143.0523137178985564, 10.69584247140429412 ) ) ;
#24646=CARTESIAN_POINT ( 'NONE',  ( 11.61527771782809637, 30.06481371789855572, 4.622313124798827388 ) ) ;
#24648=CARTESIAN_POINT ( 'NONE',  ( -14.38691631536193860, 108.2648137178985621, -5.770363421894132649 ) ) ;
#24654=CARTESIAN_POINT ( 'NONE',  ( 10.69584247140445221, 136.0476862821014379, -6.932735513423970097 ) ) ;
#24662=CARTESIAN_POINT ( 'NONE',  ( -7.228626920339069173, 140.0726862821014720, 10.49813415415989581 ) ) ;
#24667=CARTESIAN_POINT ( 'NONE',  ( 15.53471296425195369, 127.4226862821014521, -2.908627838312120684 ) ) ;
#24669=CARTESIAN_POINT ( 'NONE',  ( -2.064181346179269738, 111.8976862821014606, 9.465287035748067623 ) ) ;
#24671=CARTESIAN_POINT ( 'NONE',  ( -6.932735513423968321, 14.14768628210144463, -10.69584247140445221 ) ) ;
#24675=CARTESIAN_POINT ( 'NONE',  ( -7.954856959092191815, 77.97268628210142083, -5.529263428287477744 ) ) ;
#24677=CARTESIAN_POINT ( 'NONE',  ( -0.1745138560723084320, 128.3898137178985621, -9.500000000000005329 ) ) ;
#24683=CARTESIAN_POINT ( 'NONE',  ( -8.843639120294245259, 62.26481371789854791, -3.474262827703533230 ) ) ;
#24686=CARTESIAN_POINT ( 'NONE',  ( -6.932735513424201912, 87.85231371789856780, 10.69584247140429412 ) ) ;
#24691=CARTESIAN_POINT ( 'NONE',  ( -11.48171059495408208, 42.71481371789855075, 4.944772684328421875 ) ) ;
#24695=CARTESIAN_POINT ( 'NONE',  ( 8.715434833791931624, 27.66018628210144215, 8.962234695871760692 ) ) ;
#24701=CARTESIAN_POINT ( 'NONE',  ( 0.1745138560722779009, 68.58981371789856496, 12.50000000000000355 ) ) ;
#24707=CARTESIAN_POINT ( 'NONE',  ( -8.927990412390371944, 44.72731371789853938, -13.04141134922778988 ) ) ;
#24710=CARTESIAN_POINT ( 'NONE',  ( -8.715434833791929847, 69.06018628210145494, -8.962234695871762469 ) ) ;
#24711=CARTESIAN_POINT ( 'NONE',  ( -8.927990412390661490, 29.67268628210143788, 13.04141134922759804 ) ) ;
#24716=CARTESIAN_POINT ( 'NONE',  ( -8.927990412390661490, 38.87268628210144072, 13.04141134922759804 ) ) ;
#24723=CARTESIAN_POINT ( 'NONE',  ( -9.465287035748106703, 125.8023137178985706, 2.064181346179061460 ) ) ;
#24729=CARTESIAN_POINT ( 'NONE',  ( 12.50000000000000355, 139.8898137178985621, -0.1745138560722771515 ) ) ;
#24735=CARTESIAN_POINT ( 'NONE',  ( 6.932735513423970097, 27.94768628210144001, 10.69584247140445044 ) ) ;
#24744=CARTESIAN_POINT ( 'NONE',  ( 12.46528703574805874, 72.79768628210146630, 2.660918448318279950 ) ) ;
#24745=CARTESIAN_POINT ( 'NONE',  ( -15.50000000000000533, 6.489813717898557321, 0.1745138560722471477 ) ) ;
#24751=CARTESIAN_POINT ( 'NONE',  ( 4.944772684328420986, 123.2148137178985650, 11.48171059495408208 ) ) ;
#24756=CARTESIAN_POINT ( 'NONE',  ( 13.23911966647199812, 122.3523137178985394, 8.632099005475788900 ) ) ;
#24760=CARTESIAN_POINT ( 'NONE',  ( -2.660918448318275509, 130.2976862821014379, 12.46528703574805874 ) ) ;
#24761=CARTESIAN_POINT ( 'NONE',  ( -5.770363421893818234, 78.83518628210146062, -14.38691631536207005 ) ) ;
#24764=CARTESIAN_POINT ( 'NONE',  ( 5.770363421893814682, 92.63518628210147199, 14.38691631536207183 ) ) ;
#24768=CARTESIAN_POINT ( 'NONE',  ( 8.152565276336714462, 44.04768628210143788, -5.233372021372432847 ) ) ;
#24773=CARTESIAN_POINT ( 'NONE',  ( -8.715434833791929847, 69.06018628210145494, -8.962234695871762469 ) ) ;
#24776=CARTESIAN_POINT ( 'NONE',  ( 8.710071997420127943, 36.28518628210144215, 3.796722387233375073 ) ) ;
#24786=CARTESIAN_POINT ( 'NONE',  ( 11.48171059495408208, 84.11481371789855643, -4.944772684328420986 ) ) ;
#24787=CARTESIAN_POINT ( 'NONE',  ( -7.228626920339070061, 94.07268628210145778, 10.49813415415989404 ) ) ;
#24792=CARTESIAN_POINT ( 'NONE',  ( 5.770363421894130873, 64.56481371789854506, -14.38691631536193860 ) ) ;
#24798=CARTESIAN_POINT ( 'NONE',  ( 1.715153634034445762, 36.67731371789854933, -9.534712964251895073 ) ) ;
#24800=CARTESIAN_POINT ( 'NONE',  ( 9.465287035748106703, 102.8023137178985422, -2.064181346179063237 ) ) ;
#24802=CARTESIAN_POINT ( 'NONE',  ( -12.46528703574811558, 24.60231371789854649, 2.660918448318003726 ) ) ;
#24803=CARTESIAN_POINT ( 'NONE',  ( -8.962234695871760692, 75.96018628210144641, 8.715434833791933400 ) ) ;
#24812=CARTESIAN_POINT ( 'NONE',  ( 8.843639120294328748, 90.33518628210144641, -3.474262827703334722 ) ) ;
#24814=CARTESIAN_POINT ( 'NONE',  ( 0.1745138560725515708, 125.4101862821014635, -12.50000000000000355 ) ) ;
#24825=CARTESIAN_POINT ( 'NONE',  ( 8.962234695871567070, 131.8398137178985792, 8.715434833792127023 ) ) ;
#24833=CARTESIAN_POINT ( 'NONE',  ( 10.83675517735179206, 111.1398137178985621, -11.08355503943118769 ) ) ;
#24841=CARTESIAN_POINT ( 'NONE',  ( -10.49813415415989581, 123.9726862821014493, -7.228626920339068285 ) ) ;
#24849=CARTESIAN_POINT ( 'NONE',  ( -12.53471296425194836, 132.0226862821014606, 2.311890736173176641 ) ) ;
#24857=CARTESIAN_POINT ( 'NONE',  ( 15.46528703574804986, 127.9976862821014265, 3.257655550457285720 ) ) ;
#24859=CARTESIAN_POINT ( 'NONE',  ( 2.660918448318279950, 15.29768628210143078, -12.46528703574805697 ) ) ;
#24863=CARTESIAN_POINT ( 'NONE',  ( 3.474262827703335166, 74.23518628210142367, 8.843639120294326972 ) ) ;
#24865=CARTESIAN_POINT ( 'NONE',  ( 2.064181346179061460, 132.7023137178985337, 9.465287035748106703 ) ) ;
#24871=CARTESIAN_POINT ( 'NONE',  ( -5.529263428287297444, 63.12731371789852375, -7.954856959092311719 ) ) ;
#24875=CARTESIAN_POINT ( 'NONE',  ( -11.48171059495408208, 70.31481371789854506, 4.944772684328421875 ) ) ;
#24877=CARTESIAN_POINT ( 'NONE',  ( -8.668585281157772826, 143.0000000000000568, 10.14709209106742627 ) ) ;
#24879=CARTESIAN_POINT ( 'NONE',  ( -10.69584247140429412, 34.95231371789854791, -6.932735513424201024 ) ) ;
#24884=CARTESIAN_POINT ( 'NONE',  ( -8.962234695871760692, 20.76018628210144001, 8.715434833791933400 ) ) ;
#24889=CARTESIAN_POINT ( 'NONE',  ( -2.660918448318004614, 72.90231371789855075, -12.46528703574811558 ) ) ;
#24895=CARTESIAN_POINT ( 'NONE',  ( -15.53471296425188442, 43.57731371789854080, -2.908627838312459080 ) ) ;
#24897=CARTESIAN_POINT ( 'NONE',  ( 2.311890736173175753, 65.32268628210144357, 12.53471296425194836 ) ) ;
#24898=CARTESIAN_POINT ( 'NONE',  ( 6.092822981423978490, 6.385186282101440902, -14.25334919248782306 ) ) ;
#24902=CARTESIAN_POINT ( 'NONE',  ( 14.38691631536207538, 25.93518628210144072, -5.770363421893813793 ) ) ;
#24909=CARTESIAN_POINT ( 'NONE',  ( 1.715153634034445762, 110.2773137178985650, -9.534712964251895073 ) ) ;
#24913=EDGE_CURVE ( 'NONE', #1210, #21615, #27208, .T. ) ;
#24914=CARTESIAN_POINT ( 'NONE',  ( 6.932735513424201024, 138.4523137178985621, -10.69584247140429412 ) ) ;
#24920=CARTESIAN_POINT ( 'NONE',  ( -0.1745138560725500443, 38.01018628210144357, 12.50000000000000355 ) ) ;
#24928=CARTESIAN_POINT ( 'NONE',  ( 6.932735513423970097, 73.94768628210145778, 10.69584247140445044 ) ) ;
#24929=CARTESIAN_POINT ( 'NONE',  ( 14.25334919248795451, 10.51481371789855679, -6.092822981423661410 ) ) ;
#24934=CARTESIAN_POINT ( 'NONE',  ( -12.46528703574811558, 116.6023137178985678, 2.660918448318003726 ) ) ;
#24939=CARTESIAN_POINT ( 'NONE',  ( 14.25334919248795451, 93.31481371789855928, -6.092822981423661410 ) ) ;
#24942=CARTESIAN_POINT ( 'NONE',  ( -4.944772684328673229, 130.5851862821014606, 11.48171059495397728 ) ) ;
#24943=CARTESIAN_POINT ( 'NONE',  ( 3.257655550457285720, 61.29768628210142367, -15.46528703574804986 ) ) ;
#24946=CARTESIAN_POINT ( 'NONE',  ( 8.927990412390657937, 89.47268628210143504, -13.04141134922759804 ) ) ;
#24949=CARTESIAN_POINT ( 'NONE',  ( -9.465287035748065847, 31.39768628210144286, -2.064181346179273735 ) ) ;
#24953=CARTESIAN_POINT ( 'NONE',  ( 6.932735513423970097, 55.54768628210144499, 10.69584247140445044 ) ) ;
#24956=CARTESIAN_POINT ( 'NONE',  ( -1.715153634034234598, 23.92268628210143788, -9.534712964251941258 ) ) ;
#24965=CARTESIAN_POINT ( 'NONE',  ( -11.48171059495408208, 88.71481371789855075, 4.944772684328421875 ) ) ;
#24966=CARTESIAN_POINT ( 'NONE',  ( 6.932735513423970097, 92.34768628210144925, 10.69584247140445044 ) ) ;
#24971=CARTESIAN_POINT ( 'NONE',  ( 8.927990412390371944, 58.52731371789855785, 13.04141134922778811 ) ) ;
#24976=CARTESIAN_POINT ( 'NONE',  ( -8.843639120294245259, 43.86481371789854933, -3.474262827703533230 ) ) ;
#24979=CARTESIAN_POINT ( 'NONE',  ( 3.474262827703532341, 92.16481371789855359, -8.843639120294245259 ) ) ;
#24981=CARTESIAN_POINT ( 'NONE',  ( -11.48171059495408208, 15.11481371789855110, 4.944772684328421875 ) ) ;
#24984=CARTESIAN_POINT ( 'NONE',  ( -11.61527771782819940, 58.13518628210144357, 4.622313124798574258 ) ) ;
#24994=CARTESIAN_POINT ( 'NONE',  ( 9.500000000000005329, 100.1101862821014521, 0.1745138560725188748 ) ) ;
#24997=CARTESIAN_POINT ( 'NONE',  ( 8.962234695871762469, 117.3601862821014521, -8.715434833791931624 ) ) ;
#25010=CARTESIAN_POINT ( 'NONE',  ( 4.944772684328420986, 141.6148137178985849, 11.48171059495408208 ) ) ;
#25016=CARTESIAN_POINT ( 'NONE',  ( -4.622313124798826500, 13.96481371789853831, 11.61527771782809637 ) ) ;
#25018=CARTESIAN_POINT ( 'NONE',  ( -8.927990412390371944, 118.3273137178985763, -13.04141134922778988 ) ) ;
#25024=CARTESIAN_POINT ( 'NONE',  ( 12.46528703574805874, 109.5976862821014493, 2.660918448318279950 ) ) ;
#25030=CARTESIAN_POINT ( 'NONE',  ( -12.50000000000000355, 132.3101862821014549, -0.1745138560725492671 ) ) ;
#25034=APPLICATION_CONTEXT ( 'automotive_design' ) ;
#25037=CARTESIAN_POINT ( 'NONE',  ( 13.23911966647218996, 126.8476862821014635, -8.632099005475504683 ) ) ;
#25040=CARTESIAN_POINT ( 'NONE',  ( -11.48171059495397373, 4.085186282101443744, -4.944772684328680334 ) ) ;
#25045=CARTESIAN_POINT ( 'NONE',  ( -5.529263428287477744, 84.87268628210145494, 7.954856959092191815 ) ) ;
#25048=CARTESIAN_POINT ( 'NONE',  ( -8.710071997420207879, 134.7148137178985507, 3.796722387233182339 ) ) ;
#25055=CARTESIAN_POINT ( 'NONE',  ( -5.233372021372612259, 60.25231371789854506, 8.152565276336593669 ) ) ;
#25059=CARTESIAN_POINT ( 'NONE',  ( -12.46528703574811558, 61.40231371789855785, 2.660918448318004170 ) ) ;
#25063=CARTESIAN_POINT ( 'NONE',  ( 8.715434833792128799, 37.53981371789855359, -8.962234695871567070 ) ) ;
#25066=CARTESIAN_POINT ( 'NONE',  ( -6.932735513423968321, 4.947686282101432909, -10.69584247140445221 ) ) ;
#25073=CARTESIAN_POINT ( 'NONE',  ( -8.715434833792127023, 60.53981371789856070, 8.962234695871568846 ) ) ;
#25078=CARTESIAN_POINT ( 'NONE',  ( 8.632099005475788900, 46.45231371789854791, -13.23911966647199812 ) ) ;
#25080=CARTESIAN_POINT ( 'NONE',  ( 4.944772684328679446, 24.78518628210143859, -11.48171059495397373 ) ) ;
#25082=CARTESIAN_POINT ( 'NONE',  ( -4.622313124798576922, 69.63518628210145778, -11.61527771782819762 ) ) ;
#25083=CARTESIAN_POINT ( 'NONE',  ( 8.632099005475504683, 9.547686282101452093, 13.23911966647218996 ) ) ;
#25087=CARTESIAN_POINT ( 'NONE',  ( -15.46528703574804986, 31.39768628210144286, -3.257655550457287497 ) ) ;
#25095=CARTESIAN_POINT ( 'NONE',  ( -3.474262827703527901, 105.9648137178985650, 8.843639120294245259 ) ) ;
#25100=CARTESIAN_POINT ( 'NONE',  ( 10.49813415416005213, 120.6273137178985593, -7.228626920338837358 ) ) ;
#25107=CARTESIAN_POINT ( 'NONE',  ( 11.61527771782819940, 25.93518628210143717, -4.622313124798573369 ) ) ;
#25115=CARTESIAN_POINT ( 'NONE',  ( -12.46528703574805697, 58.99768628210144783, -2.660918448318280838 ) ) ;
#25116=CARTESIAN_POINT ( 'NONE',  ( -5.770363421893818234, 134.0351862821014493, -14.38691631536207005 ) ) ;
#25123=CARTESIAN_POINT ( 'NONE',  ( 2.311890736173452865, 119.4773137178985678, -12.53471296425189152 ) ) ;
#25129=CARTESIAN_POINT ( 'NONE',  ( -3.257655550456946880, 100.5023137178985451, -15.46528703574811736 ) ) ;
#25134=CARTESIAN_POINT ( 'NONE',  ( 11.61527771782819940, 127.1351862821014578, -4.622313124798573369 ) ) ;
#25135=CARTESIAN_POINT ( 'NONE',  ( -14.38691631536207183, 67.33518628210143220, 5.770363421893814682 ) ) ;
#25139=CARTESIAN_POINT ( 'NONE',  ( 13.23911966647218996, 80.84768628210143504, -8.632099005475504683 ) ) ;
#25142=CARTESIAN_POINT ( 'NONE',  ( -5.233372021372430183, 14.14768628210144286, -8.152565276336710909 ) ) ;
#25146=CARTESIAN_POINT ( 'NONE',  ( 0.1745138560725515708, 61.01018628210145067, -12.50000000000000355 ) ) ;
#25149=CARTESIAN_POINT ( 'NONE',  ( -8.710071997420127943, 22.48518628210144499, -3.796722387233380402 ) ) ;
#25160=CARTESIAN_POINT ( 'NONE',  ( 11.61527771782809637, 85.26481371789856212, 4.622313124798827388 ) ) ;
#25161=CARTESIAN_POINT ( 'NONE',  ( 10.49813415415989581, 82.57268628210145778, 7.228626920339069173 ) ) ;
#25167=CARTESIAN_POINT ( 'NONE',  ( -14.38691631536193860, 53.06481371789855928, -5.770363421894132649 ) ) ;
#25174=CARTESIAN_POINT ( 'NONE',  ( -8.152565276336593669, 34.95231371789854080, -5.233372021372610483 ) ) ;
#25177=CARTESIAN_POINT ( 'NONE',  ( -9.500000000000005329, 89.28981371789856780, 0.1745138560723101806 ) ) ;
#25179=CARTESIAN_POINT ( 'NONE',  ( -7.228626920338836470, 7.927313717898537782, -10.49813415416005213 ) ) ;
#25180=CARTESIAN_POINT ( 'NONE',  ( 10.49813415415989581, 73.37268628210144072, 7.228626920339068285 ) ) ;
#25188=CARTESIAN_POINT ( 'NONE',  ( -5.233372021372430183, 96.94768628210147199, -8.152565276336710909 ) ) ;
#25191=CARTESIAN_POINT ( 'NONE',  ( 4.944772684328679446, 107.5851862821014464, -11.48171059495397373 ) ) ;
#25203=CARTESIAN_POINT ( 'NONE',  ( -2.660918448318004614, 137.3023137178985564, -12.46528703574811558 ) ) ;
#25212=CARTESIAN_POINT ( 'NONE',  ( 15.50000000000000533, 121.4898137178985564, -0.1745138560722452326 ) ) ;
#25217=CARTESIAN_POINT ( 'NONE',  ( 4.944772684328679446, 107.5851862821014464, -11.48171059495397373 ) ) ;
#25224=CARTESIAN_POINT ( 'NONE',  ( -8.715434833791929847, 115.0601862821014549, -8.962234695871762469 ) ) ;
#25229=CARTESIAN_POINT ( 'NONE',  ( -5.770363421893818234, 115.6351862821014436, -14.38691631536207005 ) ) ;
#25232=CARTESIAN_POINT ( 'NONE',  ( -4.944772684328673229, 20.18518628210144783, 11.48171059495397728 ) ) ;
#25236=CARTESIAN_POINT ( 'NONE',  ( 2.064181346179272847, 88.89768628210146062, -9.465287035748065847 ) ) ;
#25243=CARTESIAN_POINT ( 'NONE',  ( -6.594114490232462877, 51.33981371789855785, 6.840914352311949109 ) ) ;
#25248=CARTESIAN_POINT ( 'NONE',  ( -4.622313124798826500, 69.16481371789855359, 11.61527771782809637 ) ) ;
#25252=CARTESIAN_POINT ( 'NONE',  ( -4.944772684328424539, 26.61481371789854578, -11.48171059495408031 ) ) ;
#25262=CARTESIAN_POINT ( 'NONE',  ( -7.228626920338836470, 72.32731371789854791, -10.49813415416005213 ) ) ;
#25267=CARTESIAN_POINT ( 'NONE',  ( 15.50000000000000533, 38.68981371789855217, -0.1745138560722452326 ) ) ;
#25270=CARTESIAN_POINT ( 'NONE',  ( -2.660918448318275509, 19.89768628210143575, 12.46528703574805874 ) ) ;
#25271=CARTESIAN_POINT ( 'NONE',  ( -2.311890736173176641, 60.72268628210144925, -12.53471296425194836 ) ) ;
#25272=CARTESIAN_POINT ( 'NONE',  ( 11.08355503943142750, 6.960186282101432198, -10.83675517735155225 ) ) ;
#25276=CARTESIAN_POINT ( 'NONE',  ( 14.25334919248782661, 36.28518628210144215, 6.092822981423971385 ) ) ;
#25282=CARTESIAN_POINT ( 'NONE',  ( -10.69584247140444866, 11.84768628210144925, 6.932735513423972762 ) ) ;
#25284=CARTESIAN_POINT ( 'NONE',  ( 6.594114490232462877, 111.1398137178985621, -6.840914352311949109 ) ) ;
#25289=CARTESIAN_POINT ( 'NONE',  ( 11.61527771782809637, 112.8648137178985564, 4.622313124798827388 ) ) ;
#25292=DIRECTION ( 'NONE',  ( -1.045431693899523221E-14, -0.1163425707149444432, 0.9932091452657080266 ) ) ;
#25302=CARTESIAN_POINT ( 'NONE',  ( -10.69584247140444866, 67.04768628210145209, 6.932735513423972762 ) ) ;
#25308=CARTESIAN_POINT ( 'NONE',  ( -12.50000000000000355, 116.8898137178985621, 0.1745138560722786503 ) ) ;
#25314=CARTESIAN_POINT ( 'NONE',  ( 6.092822981423662299, 86.41481371789855359, 14.25334919248795096 ) ) ;
#25319=CARTESIAN_POINT ( 'NONE',  ( -2.660918448318275509, 121.0976862821014635, 12.46528703574805874 ) ) ;
#25320=EDGE_CURVE ( 'NONE', #21615, #33833, #15280, .T. ) ;
#25321=CARTESIAN_POINT ( 'NONE',  ( 8.927990412390657937, 71.07268628210144357, -13.04141134922759804 ) ) ;
#25324=CARTESIAN_POINT ( 'NONE',  ( 8.632099005475504683, 83.14768628210143220, 13.23911966647218996 ) ) ;
#25327=CARTESIAN_POINT ( 'NONE',  ( -9.500000000000005329, 21.91018628210143859, -0.1745138560725176813 ) ) ;
#25331=CARTESIAN_POINT ( 'NONE',  ( -8.715434833791929847, 59.86018628210145209, -8.962234695871762469 ) ) ;
#25335=CARTESIAN_POINT ( 'NONE',  ( -3.474262827703337830, 32.83518628210143930, -8.843639120294326972 ) ) ;
#25348=CARTESIAN_POINT ( 'NONE',  ( 2.660918448318279950, 79.69768628210144357, -12.46528703574805874 ) ) ;
#25352=CARTESIAN_POINT ( 'NONE',  ( -10.83675517735179028, 51.33981371789855785, 11.08355503943118947 ) ) ;
#25358=CARTESIAN_POINT ( 'NONE',  ( 5.233372021372610483, 46.45231371789854791, -8.152565276336593669 ) ) ;
#25360=CARTESIAN_POINT ( 'NONE',  ( -1.715153634034442431, 96.47731371789852517, 9.534712964251900402 ) ) ;
#25362=CARTESIAN_POINT ( 'NONE',  ( -12.50000000000000355, 6.489813717898557321, 0.1745138560722786503 ) ) ;
#25363=CARTESIAN_POINT ( 'NONE',  ( -8.962234695871760692, 66.76018628210145778, 8.715434833791933400 ) ) ;
#25371=CARTESIAN_POINT ( 'NONE',  ( -1.715153634034234598, 69.92268628210143788, -9.534712964251941258 ) ) ;
#25373=CARTESIAN_POINT ( 'NONE',  ( -2.311890736173176641, 106.7226862821014635, -12.53471296425194836 ) ) ;
#25386=CARTESIAN_POINT ( 'NONE',  ( 12.50000000000000355, 139.8898137178985621, -0.1745138560722771515 ) ) ;
#25387=CARTESIAN_POINT ( 'NONE',  ( -4.622313124798576922, 134.0351862821014493, -11.61527771782819762 ) ) ;
#25392=CARTESIAN_POINT ( 'NONE',  ( 12.46528703574811558, 10.80231371789855466, -2.660918448318005947 ) ) ;
#25394=CARTESIAN_POINT ( 'NONE',  ( 2.908627838312458636, 119.4773137178985678, -15.53471296425188442 ) ) ;
#25399=CARTESIAN_POINT ( 'NONE',  ( -8.715434833791929847, 105.8601862821014521, -8.962234695871762469 ) ) ;
#25406=CARTESIAN_POINT ( 'NONE',  ( 11.48171059495397728, 128.2851862821014493, 4.944772684328674117 ) ) ;
#25411=CARTESIAN_POINT ( 'NONE',  ( 6.092822981423978490, 116.7851862821014635, -14.25334919248782306 ) ) ;
#25412=CARTESIAN_POINT ( 'NONE',  ( 10.69584247140445221, 7.247686282101428290, -6.932735513423970097 ) ) ;
#25415=CARTESIAN_POINT ( 'NONE',  ( 9.534712964251941258, 136.6226862821014549, -1.715153634034235708 ) ) ;
#25421=CARTESIAN_POINT ( 'NONE',  ( 9.500000000000005329, 72.51018628210145778, 0.1745138560725188748 ) ) ;
#25428=CARTESIAN_POINT ( 'NONE',  ( 5.529263428287300108, 49.32731371789854791, 7.954856959092309943 ) ) ;
#25433=CARTESIAN_POINT ( 'NONE',  ( 8.962234695871567070, 67.43981371789855928, 8.715434833792127023 ) ) ;
#25436=CARTESIAN_POINT ( 'NONE',  ( 4.622313124798831829, 27.76481371789854435, -11.61527771782809282 ) ) ;
#25450=CARTESIAN_POINT ( 'NONE',  ( -0.1745138560722442889, 36.38981371789855501, -15.50000000000000533 ) ) ;
#25452=CARTESIAN_POINT ( 'NONE',  ( 11.61527771782819940, 16.73518628210143788, -4.622313124798573369 ) ) ;
#25454=CARTESIAN_POINT ( 'NONE',  ( 10.49813415415989581, 73.37268628210144072, 7.228626920339068285 ) ) ;
#25456=CARTESIAN_POINT ( 'NONE',  ( -2.908627838312119351, 14.72268628210143859, -15.53471296425195369 ) ) ;
#25460=CARTESIAN_POINT ( 'NONE',  ( 11.08355503943142750, 6.960186282101432198, -10.83675517735155225 ) ) ;
#25467=CARTESIAN_POINT ( 'NONE',  ( 6.932735513423970097, 9.547686282101453870, 10.69584247140445044 ) ) ;
#25469=CARTESIAN_POINT ( 'NONE',  ( 0.1745138560723095977, 105.3898137178985479, 9.500000000000005329 ) ) ;
#25474=CARTESIAN_POINT ( 'NONE',  ( 6.932735513424201024, 110.8523137178985536, -10.69584247140429412 ) ) ;
#25477=CARTESIAN_POINT ( 'NONE',  ( -12.50000000000000355, 143.0000000000000284, -1.353084311261909534E-13 ) ) ;
#25487=CARTESIAN_POINT ( 'NONE',  ( -7.228626920339069173, 66.47268628210144925, 10.49813415415989581 ) ) ;
#25494=CARTESIAN_POINT ( 'NONE',  ( -6.932735513424201912, 115.4523137178985621, 10.69584247140429412 ) ) ;
#25500=CARTESIAN_POINT ( 'NONE',  ( 11.08355503943118769, 85.83981371789856496, 10.83675517735179028 ) ) ;
#25504=CARTESIAN_POINT ( 'NONE',  ( -0.1745138560725500443, 120.8101862821014691, 12.50000000000000355 ) ) ;
#25505=CARTESIAN_POINT ( 'NONE',  ( -0.1745138560725817967, 56.41018628210145636, 15.50000000000000533 ) ) ;
#25508=CARTESIAN_POINT ( 'NONE',  ( 3.257655550457285720, 79.69768628210141515, -15.46528703574804986 ) ) ;
#25510=CARTESIAN_POINT ( 'NONE',  ( -8.843639120294326972, 21.33518628210144641, 3.474262827703335166 ) ) ;
#25514=CARTESIAN_POINT ( 'NONE',  ( 12.53471296425194836, 63.02268628210145351, -2.311890736173178418 ) ) ;
#25517=CARTESIAN_POINT ( 'NONE',  ( -3.474262827703337830, 23.63518628210144357, -8.843639120294326972 ) ) ;
#25529=CARTESIAN_POINT ( 'NONE',  ( 7.228626920339069173, 71.07268628210144357, -10.49813415415989404 ) ) ;
#25535=CARTESIAN_POINT ( 'NONE',  ( 5.770363421894130873, 36.96481371789853654, -14.38691631536193860 ) ) ;
#25541=CARTESIAN_POINT ( 'NONE',  ( 2.064181346179061460, 40.70231371789854791, 9.465287035748106703 ) ) ;
#25544=CARTESIAN_POINT ( 'NONE',  ( -5.529263428287297444, 90.72731371789855359, -7.954856959092311719 ) ) ;
#25546=CARTESIAN_POINT ( 'NONE',  ( 2.311890736173452865, 18.27731371789853299, -12.53471296425189152 ) ) ;
#25548=CARTESIAN_POINT ( 'NONE',  ( -12.46528703574805697, 68.19768628210144357, -2.660918448318280838 ) ) ;
#25550=DIRECTION ( 'NONE',  ( -1.045431693899523221E-14, -0.1163425707149444432, 0.9932091452657080266 ) ) ;
#25555=CARTESIAN_POINT ( 'NONE',  ( 6.594114490232313663, 73.66018628210144925, 6.840914352312096547 ) ) ;
#25558=CARTESIAN_POINT ( 'NONE',  ( 11.48171059495397728, 109.8851862821014436, 4.944772684328674117 ) ) ;
#25570=CARTESIAN_POINT ( 'NONE',  ( -8.715434833792127023, 124.9398137178985593, 8.962234695871568846 ) ) ;
#25571=CARTESIAN_POINT ( 'NONE',  ( -11.48171059495397373, 132.8851862821014720, -4.944772684328680334 ) ) ;
#25575=CARTESIAN_POINT ( 'NONE',  ( -6.932735513424201912, 14.25231371789853441, 10.69584247140429412 ) ) ;
#25576=CARTESIAN_POINT ( 'NONE',  ( -15.50000000000000533, 98.48981371789855643, 0.1745138560722471477 ) ) ;
#25583=CARTESIAN_POINT ( 'NONE',  ( -2.660918448318275509, 121.0976862821014635, 12.46528703574805874 ) ) ;
#25589=CARTESIAN_POINT ( 'NONE',  ( -4.622313124798576922, 115.6351862821014578, -11.61527771782819762 ) ) ;
#25594=CARTESIAN_POINT ( 'NONE',  ( 13.23911966647218996, 99.24768628210145494, -8.632099005475504683 ) ) ;
#25596=CARTESIAN_POINT ( 'NONE',  ( 0.1745138560725515708, 24.21018628210144641, -12.50000000000000355 ) ) ;
#25598=CARTESIAN_POINT ( 'NONE',  ( 5.529263428287477744, 135.4726862821014777, -7.954856959092191815 ) ) ;
#25604=CARTESIAN_POINT ( 'NONE',  ( 6.594114490232313663, 64.46018628210146062, 6.840914352312096547 ) ) ;
#25611=CARTESIAN_POINT ( 'NONE',  ( -7.954856959092309943, 33.22731371789855359, 5.529263428287300108 ) ) ;
#25615=CARTESIAN_POINT ( 'NONE',  ( 12.46528703574811558, 56.80231371789857064, -2.660918448318005947 ) ) ;
#25618=CARTESIAN_POINT ( 'NONE',  ( 2.311890736173452865, 36.67731371789854933, -12.53471296425189152 ) ) ;
#25621=CARTESIAN_POINT ( 'NONE',  ( 7.228626920339068285, 6.672686282101436106, -10.49813415415989581 ) ) ;
#25634=CARTESIAN_POINT ( 'NONE',  ( -6.092822981423666739, 17.41481371789854649, -14.25334919248795096 ) ) ;
#25637=CARTESIAN_POINT ( 'NONE',  ( 5.233372021372432847, 138.3476862821014208, 8.152565276336710909 ) ) ;
#25638=CARTESIAN_POINT ( 'NONE',  ( -8.715434833791929847, 41.46018628210144641, -8.962234695871762469 ) ) ;
#25643=CARTESIAN_POINT ( 'NONE',  ( 14.25334919248782661, 17.88518628210143646, 6.092822981423971385 ) ) ;
#25651=CARTESIAN_POINT ( 'NONE',  ( 9.534712964251900402, 112.5773137178985479, 1.715153634034445540 ) ) ;
#25658=CARTESIAN_POINT ( 'NONE',  ( 4.944772684328420986, 123.2148137178985650, 11.48171059495408208 ) ) ;
#25673=CARTESIAN_POINT ( 'NONE',  ( -2.311890736173176641, 60.72268628210144925, -12.53471296425194836 ) ) ;
#25682=CARTESIAN_POINT ( 'NONE',  ( 11.61527771782809637, 103.6648137178985678, 4.622313124798827388 ) ) ;
#25688=CARTESIAN_POINT ( 'NONE',  ( -13.04141134922778456, 97.62731371789854506, 8.927990412390377273 ) ) ;
#25692=CARTESIAN_POINT ( 'NONE',  ( 10.69584247140445221, 99.24768628210146915, -6.932735513423970097 ) ) ;
#25693=CARTESIAN_POINT ( 'NONE',  ( 3.257655550457285720, 70.49768628210145494, -15.46528703574804986 ) ) ;
#25695=CARTESIAN_POINT ( 'NONE',  ( -8.632099005475501130, 60.14768628210144641, -13.23911966647218996 ) ) ;
#25697=CARTESIAN_POINT ( 'NONE',  ( 5.233372021372432847, 18.74768628210143362, 8.152565276336710909 ) ) ;
#25701=CARTESIAN_POINT ( 'NONE',  ( 8.962234695871762469, 52.96018628210144641, -8.715434833791931624 ) ) ;
#25704=CARTESIAN_POINT ( 'NONE',  ( 9.500000000000005329, 17.31018628210144428, 0.1745138560725188748 ) ) ;
#25715=CARTESIAN_POINT ( 'NONE',  ( 0.1745138560725515708, 70.21018628210144641, -12.50000000000000355 ) ) ;
#25720=CARTESIAN_POINT ( 'NONE',  ( -15.46528703574811736, 33.80231371789854222, 3.257655550456946436 ) ) ;
#25727=CARTESIAN_POINT ( 'NONE',  ( -8.710071997420207879, 24.31481371789855217, 3.796722387233182339 ) ) ;
#25733=CARTESIAN_POINT ( 'NONE',  ( 0.1745138560722779009, 13.38981371789854613, 12.50000000000000355 ) ) ;
#25735=CARTESIAN_POINT ( 'NONE',  ( 12.53471296425194836, 63.02268628210145351, -2.311890736173178418 ) ) ;
#25742=CARTESIAN_POINT ( 'NONE',  ( -8.152565276336710909, 85.44768628210142936, 5.233372021372435512 ) ) ;
#25744=CARTESIAN_POINT ( 'NONE',  ( 12.50000000000000355, 109.3101862821014549, 0.1745138560725507937 ) ) ;
#25756=CARTESIAN_POINT ( 'NONE',  ( 12.53471296425189330, 121.7773137178985792, 2.311890736173451977 ) ) ;
#25757=CARTESIAN_POINT ( 'NONE',  ( -7.228626920339070061, 121.6726862821014521, 10.49813415415989404 ) ) ;
#25762=CARTESIAN_POINT ( 'NONE',  ( 15.50000000000000533, 103.0898137178985792, -0.1745138560722452326 ) ) ;
#25764=CARTESIAN_POINT ( 'NONE',  ( 10.49813415415989581, 91.77268628210144641, 7.228626920339068285 ) ) ;
#25767=CARTESIAN_POINT ( 'NONE',  ( 11.61527771782819940, 117.9351862821014549, -4.622313124798573369 ) ) ;
#25772=CARTESIAN_POINT ( 'NONE',  ( -12.53471296425194836, 113.6226862821014407, 2.311890736173176641 ) ) ;
#25779=CARTESIAN_POINT ( 'NONE',  ( -8.632099005475501130, 106.1476862821014322, -13.23911966647218996 ) ) ;
#25780=CARTESIAN_POINT ( 'NONE',  ( -11.61527771782819940, 21.33518628210144641, 4.622313124798574258 ) ) ;
#25783=CARTESIAN_POINT ( 'NONE',  ( 5.233372021372432847, 138.3476862821014208, 8.152565276336710909 ) ) ;
#25788=CARTESIAN_POINT ( 'NONE',  ( -9.465287035748065847, 68.19768628210142936, -2.064181346179273735 ) ) ;
#25795=CARTESIAN_POINT ( 'NONE',  ( -7.954856959092309943, 42.42731371789855643, 5.529263428287300108 ) ) ;
#25800=CARTESIAN_POINT ( 'NONE',  ( 10.49813415416005213, 37.82731371789854791, -7.228626920338837358 ) ) ;
#25803=CARTESIAN_POINT ( 'NONE',  ( -2.908627838312453306, 142.4773137178985678, 15.53471296425188797 ) ) ;
#25813=( NAMED_UNIT ( * ) SI_UNIT ( $, .STERADIAN. ) SOLID_ANGLE_UNIT ( ) );
#25822=CARTESIAN_POINT ( 'NONE',  ( 2.908627838312458636, 27.47731371789854649, -15.53471296425188442 ) ) ;
#25824=CARTESIAN_POINT ( 'NONE',  ( 7.228626920339068285, 15.87268628210144961, -10.49813415415989581 ) ) ;
#25825=CARTESIAN_POINT ( 'NONE',  ( 4.944772684328679446, 43.18518628210144072, -11.48171059495397373 ) ) ;
#25836=CARTESIAN_POINT ( 'NONE',  ( 9.534712964251900402, 94.17731371789857064, 1.715153634034445540 ) ) ;
#25844=CARTESIAN_POINT ( 'NONE',  ( -11.61527771782809282, 117.4648137178985650, -4.622313124798832717 ) ) ;
#25849=CARTESIAN_POINT ( 'NONE',  ( 7.228626920338837358, 58.52731371789855785, 10.49813415416005036 ) ) ;
#25858=CARTESIAN_POINT ( 'NONE',  ( 8.962234695871762469, 62.16018628210144215, -8.715434833791931624 ) ) ;
#25864=CARTESIAN_POINT ( 'NONE',  ( -6.932735513424201912, 97.05231371789857064, 10.69584247140429412 ) ) ;
#25870=CARTESIAN_POINT ( 'NONE',  ( -2.908627838312453306, 68.87731371789855928, 15.53471296425188797 ) ) ;
#25875=CARTESIAN_POINT ( 'NONE',  ( 4.944772684328679446, 107.5851862821014464, -11.48171059495397373 ) ) ;
#25876=CARTESIAN_POINT ( 'NONE',  ( -10.83675517735155047, 50.66018628210144925, -11.08355503943142750 ) ) ;
#25879=CARTESIAN_POINT ( 'NONE',  ( -13.23911966647218463, 57.84768628210144925, 8.632099005475506459 ) ) ;
#25885=CARTESIAN_POINT ( 'NONE',  ( 4.622313124798573369, 46.63518628210145067, 11.61527771782819940 ) ) ;
#25888=CARTESIAN_POINT ( 'NONE',  ( -3.796722387233375073, 10.98518628210143433, 8.710071997420127943 ) ) ;
#25899=CARTESIAN_POINT ( 'NONE',  ( 8.715434833791931624, 64.46018628210146062, 8.962234695871760692 ) ) ;
#25907=CARTESIAN_POINT ( 'NONE',  ( -10.83675517735179028, 32.93981371789854506, 11.08355503943118947 ) ) ;
#25914=CARTESIAN_POINT ( 'NONE',  ( 9.500000000000005329, 20.28981371789855004, -0.1745138560723090149 ) ) ;
#25919=CARTESIAN_POINT ( 'NONE',  ( -2.908627838312453306, 133.2773137178985507, 15.53471296425188797 ) ) ;
#25922=CARTESIAN_POINT ( 'NONE',  ( 4.622313124798573369, 37.43518628210144783, 11.61527771782819940 ) ) ;
#25930=CARTESIAN_POINT ( 'NONE',  ( 5.233372021372432847, 73.94768628210142936, 8.152565276336710909 ) ) ;
#25933=CARTESIAN_POINT ( 'NONE',  ( 12.46528703574805874, 100.3976862821014464, 2.660918448318279950 ) ) ;
#25945=CARTESIAN_POINT ( 'NONE',  ( 6.932735513424201024, 120.0523137178985564, -10.69584247140429412 ) ) ;
#25946=CARTESIAN_POINT ( 'NONE',  ( 10.49813415415989581, 119.3726862821014549, 7.228626920339069173 ) ) ;
#25952=CARTESIAN_POINT ( 'NONE',  ( 2.908627838312458636, 101.0773137178985479, -15.53471296425188442 ) ) ;
#25956=CARTESIAN_POINT ( 'NONE',  ( 8.843639120294245259, 76.06481371789855928, 3.474262827703527901 ) ) ;
#25959=CARTESIAN_POINT ( 'NONE',  ( -7.228626920338836470, 53.92731371789854933, -10.49813415416005213 ) ) ;
#25961=CARTESIAN_POINT ( 'NONE',  ( 4.622313124798573369, 111.0351862821014635, 11.61527771782819940 ) ) ;
#25966=CARTESIAN_POINT ( 'NONE',  ( -13.23911966647218463, 94.64768628210147483, 8.632099005475506459 ) ) ;
#25967=CARTESIAN_POINT ( 'NONE',  ( -11.48171059495397373, 22.48518628210144499, -4.944772684328680334 ) ) ;
#25970=CARTESIAN_POINT ( 'NONE',  ( -3.796722387233375073, 130.5851862821014606, 8.710071997420127943 ) ) ;
#25973=CARTESIAN_POINT ( 'NONE',  ( 8.843639120294328748, 71.93518628210142651, -3.474262827703334722 ) ) ;
#25982=CARTESIAN_POINT ( 'NONE',  ( -6.840914352311947333, 35.23981371789855643, -6.594114490232462877 ) ) ;
#25987=CARTESIAN_POINT ( 'NONE',  ( 11.61527771782809637, 39.26481371789855501, 4.622313124798827388 ) ) ;
#25990=CARTESIAN_POINT ( 'NONE',  ( 11.08355503943118769, 141.0398137178985678, 10.83675517735179028 ) ) ;
#26007=CARTESIAN_POINT ( 'NONE',  ( 8.632099005475788900, 18.85231371789855359, -13.23911966647199812 ) ) ;
#26009=CARTESIAN_POINT ( 'NONE',  ( -12.46528703574805697, 3.797686282101447652, -2.660918448318280838 ) ) ;
#26010=CARTESIAN_POINT ( 'NONE',  ( 11.48171059495397728, 54.68518628210144783, 4.944772684328674117 ) ) ;
#26021=CARTESIAN_POINT ( 'NONE',  ( 8.152565276336593669, 94.75231371789854506, 5.233372021372610483 ) ) ;
#26028=CARTESIAN_POINT ( 'NONE',  ( 4.622313124798831829, 101.3648137178985564, -11.61527771782809282 ) ) ;
#26032=CARTESIAN_POINT ( 'NONE',  ( 2.311890736173452865, 64.27731371789855075, -12.53471296425189152 ) ) ;
#26043=CARTESIAN_POINT ( 'NONE',  ( 6.932735513423970097, 37.14768628210143930, 10.69584247140445044 ) ) ;
#26049=CARTESIAN_POINT ( 'NONE',  ( -2.311890736173448424, 96.47731371789855359, 12.53471296425189330 ) ) ;
#26054=CARTESIAN_POINT ( 'NONE',  ( 14.25334919248795451, 84.11481371789855643, -6.092822981423661410 ) ) ;
#26058=CARTESIAN_POINT ( 'NONE',  ( -6.932735513423968321, 106.1476862821014606, -10.69584247140445221 ) ) ;
#26059=CARTESIAN_POINT ( 'NONE',  ( -15.50000000000000533, 49.51018628210145067, -0.1745138560725808530 ) ) ;
#26063=CARTESIAN_POINT ( 'NONE',  ( 8.927990412390657937, 71.07268628210144357, -13.04141134922759804 ) ) ;
#26070=CARTESIAN_POINT ( 'NONE',  ( -11.61527771782819940, 39.73518628210144499, 4.622313124798574258 ) ) ;
#26073=CARTESIAN_POINT ( 'NONE',  ( 7.954856959092191815, 8.972686282101431487, 5.529263428287477744 ) ) ;
#26083=CARTESIAN_POINT ( 'NONE',  ( 4.944772684328679446, 70.78518628210144925, -11.48171059495397373 ) ) ;
#26090=CARTESIAN_POINT ( 'NONE',  ( -14.25334919248795096, 33.51481371789854791, 6.092822981423662299 ) ) ;
#26097=CARTESIAN_POINT ( 'NONE',  ( -7.954856959092309943, 24.02731371789854364, 5.529263428287300108 ) ) ;
#26102=CARTESIAN_POINT ( 'NONE',  ( -13.23911966647199812, 126.9523137178985621, -8.632099005475788900 ) ) ;
#26104=CARTESIAN_POINT ( 'NONE',  ( -8.962234695871760692, 39.16018628210144215, 8.715434833791933400 ) ) ;
#26111=CARTESIAN_POINT ( 'NONE',  ( -0.1745138560725182642, 84.01018628210145778, 9.500000000000005329 ) ) ;
#26114=CARTESIAN_POINT ( 'NONE',  ( -12.50000000000000355, 86.31018628210145494, -0.1745138560725492671 ) ) ;
#26126=CARTESIAN_POINT ( 'NONE',  ( 10.69584247140429589, 113.1523137178985650, 6.932735513424201024 ) ) ;
#26127=CARTESIAN_POINT ( 'NONE',  ( -10.49813415415989404, 123.9726862821014493, -7.228626920339069173 ) ) ;
#26133=CARTESIAN_POINT ( 'NONE',  ( -15.46528703574811736, 89.00231371789853085, 3.257655550456946436 ) ) ;
#26138=CARTESIAN_POINT ( 'NONE',  ( 6.840914352311949109, 67.43981371789855928, 6.594114490232462877 ) ) ;
#26142=CARTESIAN_POINT ( 'NONE',  ( -10.49813415416004858, 42.42731371789855643, 7.228626920338839135 ) ) ;
#26144=CARTESIAN_POINT ( 'NONE',  ( 10.49813415415989581, 100.9726862821014635, 7.228626920339068285 ) ) ;
#26150=CARTESIAN_POINT ( 'NONE',  ( -14.38691631536207183, 94.93518628210146915, 5.770363421893814682 ) ) ;
#26151=CARTESIAN_POINT ( 'NONE',  ( -8.962234695871760692, 11.56018628210145316, 8.715434833791933400 ) ) ;
#26154=CARTESIAN_POINT ( 'NONE',  ( 8.710071997420127943, 128.2851862821014493, 3.796722387233375073 ) ) ;
#26159=CARTESIAN_POINT ( 'NONE',  ( -6.594114490232312775, 69.06018628210144072, -6.840914352312096547 ) ) ;
#26166=CARTESIAN_POINT ( 'NONE',  ( -2.064181346179062349, 45.30231371789854933, -9.465287035748106703 ) ) ;
#26171=CARTESIAN_POINT ( 'NONE',  ( -4.944772684328424539, 35.81481371789854506, -11.48171059495408031 ) ) ;
#26174=CARTESIAN_POINT ( 'NONE',  ( 4.622313124798831829, 18.56481371789855928, -11.61527771782809282 ) ) ;
#26188=CARTESIAN_POINT ( 'NONE',  ( 3.257655550456945548, 22.30231371789854933, 15.46528703574811736 ) ) ;
#26190=CARTESIAN_POINT ( 'NONE',  ( 11.61527771782819940, 7.535186282101452804, -4.622313124798573369 ) ) ;
#26192=CARTESIAN_POINT ( 'NONE',  ( 12.53471296425194836, 44.62268628210144783, -2.311890736173178418 ) ) ;
#26204=CARTESIAN_POINT ( 'NONE',  ( 1.715153634034445762, 91.87731371789854506, -9.534712964251895073 ) ) ;
#26210=CARTESIAN_POINT ( 'NONE',  ( -11.48171059495408208, 107.1148137178985564, 4.944772684328421875 ) ) ;
#26213=CARTESIAN_POINT ( 'NONE',  ( -4.944772684328424539, 72.61481371789855643, -11.48171059495408031 ) ) ;
#26222=CARTESIAN_POINT ( 'NONE',  ( 12.53471296425194836, 35.42268628210144499, -2.311890736173178418 ) ) ;
#26227=CARTESIAN_POINT ( 'NONE',  ( 8.962234695871567070, 104.2398137178985564, 8.715434833792127023 ) ) ;
#26232=CARTESIAN_POINT ( 'NONE',  ( 11.08355503943118769, 76.63981371789854791, 10.83675517735179028 ) ) ;
#26236=CARTESIAN_POINT ( 'NONE',  ( -0.1745138560725500443, 102.4101862821014493, 12.50000000000000355 ) ) ;
#26237=CARTESIAN_POINT ( 'NONE',  ( 6.092822981423978490, 52.38518628210145778, -14.25334919248782306 ) ) ;
#26242=CARTESIAN_POINT ( 'NONE',  ( 11.08355503943142750, 71.36018628210143788, -10.83675517735155225 ) ) ;
#26248=CARTESIAN_POINT ( 'NONE',  ( 7.228626920339068285, 43.47268628210144925, -10.49813415415989581 ) ) ;
#26251=CARTESIAN_POINT ( 'NONE',  ( -8.152565276336710909, 11.84768628210144747, 5.233372021372435512 ) ) ;
#26263=CARTESIAN_POINT ( 'NONE',  ( -10.49813415415989404, 68.77268628210144641, -7.228626920339069173 ) ) ;
#26270=CARTESIAN_POINT ( 'NONE',  ( 6.092822981423662299, 31.21481371789855430, 14.25334919248795096 ) ) ;
#26278=CARTESIAN_POINT ( 'NONE',  ( 8.843639120294245259, 20.86481371789854578, 3.474262827703527901 ) ) ;
#26285=CARTESIAN_POINT ( 'NONE',  ( -15.53471296425188442, 126.3773137178985309, -2.908627838312459080 ) ) ;
#26287=CARTESIAN_POINT ( 'NONE',  ( -2.660918448318275509, 47.49768628210144783, 12.46528703574805874 ) ) ;
#26293=CARTESIAN_POINT ( 'NONE',  ( 7.954856959092191815, 54.97268628210144215, 5.529263428287477744 ) ) ;
#26296=CARTESIAN_POINT ( 'NONE',  ( 8.715434833791931624, 101.2601862821014578, 8.962234695871760692 ) ) ;
#26309=CARTESIAN_POINT ( 'NONE',  ( -0.1745138560722763466, 128.3898137178985621, -12.50000000000000355 ) ) ;
#26310=CARTESIAN_POINT ( 'NONE',  ( 2.660918448318279950, 116.4976862821014549, -12.46528703574805874 ) ) ;
#26316=CARTESIAN_POINT ( 'NONE',  ( 3.257655550456945548, 86.70231371789851949, 15.46528703574811736 ) ) ;
#26321=CARTESIAN_POINT ( 'NONE',  ( -5.233372021372612259, 69.45231371789853370, 8.152565276336593669 ) ) ;
#26325=CARTESIAN_POINT ( 'NONE',  ( 11.48171059495408208, 47.31481371789855928, -4.944772684328420986 ) ) ;
#26327=CARTESIAN_POINT ( 'NONE',  ( -12.46528703574805697, 104.9976862821014691, -2.660918448318280838 ) ) ;
#26330=CARTESIAN_POINT ( 'NONE',  ( -12.50000000000000355, 141.5101862821014720, -0.1745138560725492671 ) ) ;
#26332=CARTESIAN_POINT ( 'NONE',  ( -8.927990412390661490, 103.2726862821014322, 13.04141134922759804 ) ) ;
#26336=CARTESIAN_POINT ( 'NONE',  ( 8.710071997420127943, 109.8851862821014720, 3.796722387233375073 ) ) ;
#26339=CARTESIAN_POINT ( 'NONE',  ( 0.1745138560725837118, 15.01018628210143291, -15.50000000000000533 ) ) ;
#26343=CARTESIAN_POINT ( 'NONE',  ( -5.233372021372430183, 60.14768628210144641, -8.152565276336710909 ) ) ;
#26351=CARTESIAN_POINT ( 'NONE',  ( 5.233372021372610483, 37.25231371789855217, -8.152565276336593669 ) ) ;
#26355=CARTESIAN_POINT ( 'NONE',  ( 7.228626920338837358, 49.32731371789855501, 10.49813415416005036 ) ) ;
#26357=CARTESIAN_POINT ( 'NONE',  ( -8.715434833792127023, 14.53981371789855892, 8.962234695871568846 ) ) ;
#26368=PRESENTATION_STYLE_ASSIGNMENT (( #1157 ) ) ;
#26375=CARTESIAN_POINT ( 'NONE',  ( -8.632099005475794229, 14.25231371789853618, 13.23911966647199812 ) ) ;
#26377=CARTESIAN_POINT ( 'NONE',  ( 6.594114490232313663, 128.8601862821014663, 6.840914352312096547 ) ) ;
#26379=CARTESIAN_POINT ( 'NONE',  ( 7.228626920339068285, 52.67268628210144499, -10.49813415415989581 ) ) ;
#26385=CARTESIAN_POINT ( 'NONE',  ( 5.529263428287477744, 15.87268628210144605, -7.954856959092191815 ) ) ;
#26394=CARTESIAN_POINT ( 'NONE',  ( 0.1745138560723095977, 86.98981371789857064, 9.500000000000005329 ) ) ;
#26400=CARTESIAN_POINT ( 'NONE',  ( 7.228626920338837358, 104.5273137178985507, 10.49813415416005036 ) ) ;
#26404=CARTESIAN_POINT ( 'NONE',  ( -0.1745138560722763466, 63.98981371789854933, -12.50000000000000355 ) ) ;
#26410=CARTESIAN_POINT ( 'NONE',  ( 7.228626920339068285, 43.47268628210144925, -10.49813415415989581 ) ) ;
#26414=CARTESIAN_POINT ( 'NONE',  ( 12.46528703574811558, 112.0023137178985735, -2.660918448318005503 ) ) ;
#26420=CARTESIAN_POINT ( 'NONE',  ( 8.632099005475788900, 74.05231371789854222, -13.23911966647199812 ) ) ;
#26424=CARTESIAN_POINT ( 'NONE',  ( -8.715434833791929847, 96.66018628210146346, -8.962234695871762469 ) ) ;
#26425=CARTESIAN_POINT ( 'NONE',  ( 15.53471296425195369, 44.62268628210144783, -2.908627838312120684 ) ) ;
#26428=CARTESIAN_POINT ( 'NONE',  ( 14.25334919248782661, 63.88518628210145778, 6.092822981423971385 ) ) ;
#26435=CARTESIAN_POINT ( 'NONE',  ( 8.962234695871762469, 34.56018628210144783, -8.715434833791931624 ) ) ;
#26439=CARTESIAN_POINT ( 'NONE',  ( 8.710071997420127943, 8.685186282101437172, 3.796722387233375073 ) ) ;
#26450=CARTESIAN_POINT ( 'NONE',  ( 0.1745138560725515708, 42.61018628210144499, -12.50000000000000355 ) ) ;
#26456=CARTESIAN_POINT ( 'NONE',  ( -4.622313124798576922, 97.23518628210145209, -11.61527771782819762 ) ) ;
#26457=CARTESIAN_POINT ( 'NONE',  ( -15.53471296425188442, 25.17731371789854933, -2.908627838312459080 ) ) ;
#26463=CARTESIAN_POINT ( 'NONE',  ( -9.500000000000005329, 24.88981371789854080, 0.1745138560723101806 ) ) ;
#26470=CARTESIAN_POINT ( 'NONE',  ( 15.53471296425188797, 130.9773137178985394, 2.908627838312457747 ) ) ;
#26473=CARTESIAN_POINT ( 'NONE',  ( 12.50000000000000355, 44.91018628210144215, 0.1745138560725507937 ) ) ;
#26480=CARTESIAN_POINT ( 'NONE',  ( 6.594114490232313663, 64.46018628210146062, 6.840914352312096547 ) ) ;
#26484=CARTESIAN_POINT ( 'NONE',  ( -2.311890736173176641, 88.32268628210144357, -12.53471296425194836 ) ) ;
#26496=CARTESIAN_POINT ( 'NONE',  ( 11.48171059495408208, 102.5148137178985621, -4.944772684328420986 ) ) ;
#26497=CARTESIAN_POINT ( 'NONE',  ( -12.46528703574805874, 114.1976862821014578, -2.660918448318280838 ) ) ;
#26503=CARTESIAN_POINT ( 'NONE',  ( 2.908627838312458636, 73.47731371789855359, -15.53471296425188442 ) ) ;
#26506=CARTESIAN_POINT ( 'NONE',  ( -0.1745138560725182642, 102.4101862821014493, 9.500000000000005329 ) ) ;
#26509=CARTESIAN_POINT ( 'NONE',  ( -1.715153634034442431, 78.07731371789854791, 9.534712964251900402 ) ) ;
#26513=CARTESIAN_POINT ( 'NONE',  ( 12.53471296425189330, 48.17731371789854933, 2.311890736173451977 ) ) ;
#26515=CARTESIAN_POINT ( 'NONE',  ( -10.49813415415989581, 105.5726862821014578, -7.228626920339068285 ) ) ;
#26521=CARTESIAN_POINT ( 'NONE',  ( -6.092822981423970496, 84.58518628210146062, 14.25334919248782661 ) ) ;
#26525=CARTESIAN_POINT ( 'NONE',  ( 2.064181346179272847, 107.2976862821014521, -9.465287035748065847 ) ) ;
#26527=CARTESIAN_POINT ( 'NONE',  ( 15.46528703574804986, 17.59768628210143504, 3.257655550457285720 ) ) ;
#26539=CARTESIAN_POINT ( 'NONE',  ( -8.710071997420207879, 15.11481371789854933, 3.796722387233182339 ) ) ;
#26544=CARTESIAN_POINT ( 'NONE',  ( 4.944772684328420986, 49.61481371789855643, 11.48171059495408208 ) ) ;
#26546=CARTESIAN_POINT ( 'NONE',  ( -6.932735513424201912, 14.25231371789853441, 10.69584247140429412 ) ) ;
#26564=CARTESIAN_POINT ( 'NONE',  ( 13.04141134922759804, 137.7726862821014606, 8.927990412390657937 ) ) ;
#26566=CARTESIAN_POINT ( 'NONE',  ( -9.534712964251941258, 132.0226862821014322, 1.715153634034234154 ) ) ;
#26568=CARTESIAN_POINT ( 'NONE',  ( -6.932735513423968321, 32.54768628210144499, -10.69584247140445221 ) ) ;
#26572=CARTESIAN_POINT ( 'NONE',  ( 3.257655550457285720, 125.6976862821014578, -15.46528703574804986 ) ) ;
#26574=CARTESIAN_POINT ( 'NONE',  ( 9.534712964251900402, 140.1773137178985564, 1.715153634034445540 ) ) ;
#26581=CARTESIAN_POINT ( 'NONE',  ( 9.500000000000005329, 93.88981371789856212, -0.1745138560723090149 ) ) ;
#26586=CARTESIAN_POINT ( 'NONE',  ( -0.1745138560722763466, 91.58981371789856496, -12.50000000000000355 ) ) ;
#26590=CARTESIAN_POINT ( 'NONE',  ( 8.715434833792128799, 65.13981371789854791, -8.962234695871567070 ) ) ;
#26597=CARTESIAN_POINT ( 'NONE',  ( -0.1745138560725500443, 38.01018628210144357, 12.50000000000000355 ) ) ;
#26604=CARTESIAN_POINT ( 'NONE',  ( -12.46528703574811558, 79.80231371789857064, 2.660918448318003726 ) ) ;
#26611=CARTESIAN_POINT ( 'NONE',  ( -0.1745138560722442889, 63.98981371789855643, -15.50000000000000533 ) ) ;
#26614=CARTESIAN_POINT ( 'NONE',  ( -2.311890736173176641, 79.12268628210145494, -12.53471296425194836 ) ) ;
#26615=CARTESIAN_POINT ( 'NONE',  ( -2.908627838312119351, 42.32268628210145067, -15.53471296425195369 ) ) ;
#26618=CARTESIAN_POINT ( 'NONE',  ( 6.092822981423978490, 52.38518628210145778, -14.25334919248782306 ) ) ;
#26624=CARTESIAN_POINT ( 'NONE',  ( 11.61527771782819940, 16.73518628210143788, -4.622313124798573369 ) ) ;
#26625=CARTESIAN_POINT ( 'NONE',  ( 0.1745138560723095977, 142.1898137178985451, 9.500000000000005329 ) ) ;
#26636=CARTESIAN_POINT ( 'NONE',  ( 11.48171059495397728, 45.48518628210145209, 4.944772684328674117 ) ) ;
#26645=CARTESIAN_POINT ( 'NONE',  ( 2.311890736173175753, 102.1226862821014691, 12.53471296425194836 ) ) ;
#26646=CARTESIAN_POINT ( 'NONE',  ( -8.632099005475794229, 14.25231371789853618, 13.23911966647199812 ) ) ;
#26652=CARTESIAN_POINT ( 'NONE',  ( -11.61527771782809282, 135.8648137178985849, -4.622313124798832717 ) ) ;
#26659=CARTESIAN_POINT ( 'NONE',  ( 8.632099005475788900, 129.2523137178985451, -13.23911966647199812 ) ) ;
#26662=CARTESIAN_POINT ( 'NONE',  ( 8.715434833791931624, 46.06018628210144072, 8.962234695871760692 ) ) ;
#26666=CARTESIAN_POINT ( 'NONE',  ( 15.50000000000000533, 109.3101862821014549, 0.1745138560725827404 ) ) ;
#26669=CARTESIAN_POINT ( 'NONE',  ( -9.500000000000005329, 49.51018628210145067, -0.1745138560725176813 ) ) ;
#26672=CARTESIAN_POINT ( 'NONE',  ( 10.49813415415989581, 100.9726862821014635, 7.228626920339068285 ) ) ;
#26685=CARTESIAN_POINT ( 'NONE',  ( -10.49813415416004858, 106.8273137178985479, 7.228626920338839135 ) ) ;
#26686=CARTESIAN_POINT ( 'NONE',  ( 10.49813415415989581, 110.1726862821014521, 7.228626920339069173 ) ) ;
#26688=ORIENTED_EDGE ( 'NONE', *, *, #14814, .F. ) ;
#26691=CARTESIAN_POINT ( 'NONE',  ( -15.53471296425188442, 71.17731371789855643, -2.908627838312459080 ) ) ;
#26694=CARTESIAN_POINT ( 'NONE',  ( 6.840914352312096547, 108.1601862821014635, -6.594114490232313663 ) ) ;
#26696=CARTESIAN_POINT ( 'NONE',  ( -9.500000000000005329, 80.08981371789856496, 0.1745138560723101806 ) ) ;
#26698=CARTESIAN_POINT ( 'NONE',  ( -9.500000000000005329, 107.6898137178985735, 0.1745138560723101806 ) ) ;
#26700=CARTESIAN_POINT ( 'NONE',  ( -8.962234695871565293, 53.63981371789855501, -8.715434833792128799 ) ) ;
#26703=CARTESIAN_POINT ( 'NONE',  ( 11.61527771782819940, 99.53518628210144925, -4.622313124798573369 ) ) ;
#26706=CARTESIAN_POINT ( 'NONE',  ( 8.962234695871762469, 135.7601862821014720, -8.715434833791931624 ) ) ;
#26708=CARTESIAN_POINT ( 'NONE',  ( 14.25334919248782661, 82.28518628210146346, 6.092822981423971385 ) ) ;
#26711=DIRECTION ( 'NONE',  ( 0.000000000000000000, 0.9932091452657081376, 0.1163425707149433469 ) ) ;
#26713=CARTESIAN_POINT ( 'NONE',  ( 9.465287035748067623, 118.7976862821014521, 2.064181346179272847 ) ) ;
#26715=CARTESIAN_POINT ( 'NONE',  ( -15.53471296425195369, 12.42268628210144144, 2.908627838312118019 ) ) ;
#26726=CARTESIAN_POINT ( 'NONE',  ( 3.796722387233182339, 22.01481371789855501, 8.710071997420207879 ) ) ;
#26731=CARTESIAN_POINT ( 'NONE',  ( 0.1745138560722779009, 31.78981371789854649, 12.50000000000000355 ) ) ;
#26733=CARTESIAN_POINT ( 'NONE',  ( 10.83675517735179206, 129.5398137178985678, -11.08355503943118769 ) ) ;
#26754=CARTESIAN_POINT ( 'NONE',  ( -2.908627838312119351, 134.3226862821014436, -15.53471296425195369 ) ) ;
#26757=CARTESIAN_POINT ( 'NONE',  ( 5.233372021372432847, 129.1476862821014322, 8.152565276336710909 ) ) ;
#26759=CARTESIAN_POINT ( 'NONE',  ( -4.622313124798576922, 23.63518628210144357, -11.61527771782819762 ) ) ;
#26763=CARTESIAN_POINT ( 'NONE',  ( 10.83675517735155225, 119.6601862821014635, 11.08355503943142573 ) ) ;
#26765=CARTESIAN_POINT ( 'NONE',  ( 7.954856959092311719, 139.0273137178985507, -5.529263428287300108 ) ) ;
#26772=CARTESIAN_POINT ( 'NONE',  ( -8.152565276336593669, 71.75231371789854506, -5.233372021372610483 ) ) ;
#26776=CARTESIAN_POINT ( 'NONE',  ( 4.944772684328420986, 104.8148137178985593, 11.48171059495408208 ) ) ;
#26781=CARTESIAN_POINT ( 'NONE',  ( -8.962234695871565293, 53.63981371789855501, -8.715434833792128799 ) ) ;
#26784=ORIENTED_EDGE ( 'NONE', *, *, #14814, .T. ) ;
#26788=CARTESIAN_POINT ( 'NONE',  ( 8.962234695871762469, 43.76018628210144357, -8.715434833791931624 ) ) ;
#26795=CARTESIAN_POINT ( 'NONE',  ( 10.69584247140429589, 76.35231371789855359, 6.932735513424201024 ) ) ;
#26800=CARTESIAN_POINT ( 'NONE',  ( 2.908627838312458636, 64.27731371789853654, -15.53471296425188442 ) ) ;
#26804=CARTESIAN_POINT ( 'NONE',  ( -6.932735513423968321, 87.74768628210145494, -10.69584247140445221 ) ) ;
#26805=CARTESIAN_POINT ( 'NONE',  ( 6.092822981423978490, 33.98518628210143788, -14.25334919248782306 ) ) ;
#26809=CARTESIAN_POINT ( 'NONE',  ( 11.08355503943142750, 43.76018628210144357, -10.83675517735155225 ) ) ;
#26815=CARTESIAN_POINT ( 'NONE',  ( -4.622313124798576922, 14.43518628210144250, -11.61527771782819762 ) ) ;
#26817=CARTESIAN_POINT ( 'NONE',  ( 8.843639120294245259, 122.0648137178985877, 3.474262827703527901 ) ) ;
#26828=CARTESIAN_POINT ( 'NONE',  ( -4.944772684328673229, 47.78518628210144925, 11.48171059495397728 ) ) ;
#26837=CARTESIAN_POINT ( 'NONE',  ( -8.715434833791929847, 87.46018628210144641, -8.962234695871762469 ) ) ;
#26838=CARTESIAN_POINT ( 'NONE',  ( 15.53471296425188797, 20.57731371789854435, 2.908627838312457747 ) ) ;
#26844=CARTESIAN_POINT ( 'NONE',  ( 10.69584247140429589, 131.5523137178985564, 6.932735513424201024 ) ) ;
#26851=CARTESIAN_POINT ( 'NONE',  ( 15.50000000000000533, 121.4898137178985564, -0.1745138560722452326 ) ) ;
#26854=CARTESIAN_POINT ( 'NONE',  ( -2.311890736173176641, 33.12268628210144072, -12.53471296425194836 ) ) ;
#26858=CARTESIAN_POINT ( 'NONE',  ( -13.04141134922759804, 96.37268628210144072, -8.927990412390657937 ) ) ;
#26861=CARTESIAN_POINT ( 'NONE',  ( -9.534712964251941258, 49.22268628210144215, 1.715153634034234154 ) ) ;
#26865=CARTESIAN_POINT ( 'NONE',  ( -10.69584247140444866, 76.24768628210144072, 6.932735513423972762 ) ) ;
#26878=CARTESIAN_POINT ( 'NONE',  ( 10.69584247140429589, 103.9523137178985621, 6.932735513424201024 ) ) ;
#26879=CARTESIAN_POINT ( 'NONE',  ( -12.46528703574805874, 95.79768628210145209, -2.660918448318280838 ) ) ;
#26884=CARTESIAN_POINT ( 'NONE',  ( 0.1745138560722461762, 68.58981371789855075, 15.50000000000000533 ) ) ;
#26887=CARTESIAN_POINT ( 'NONE',  ( 8.152565276336714462, 108.4476862821014294, -5.233372021372432847 ) ) ;
#26889=CARTESIAN_POINT ( 'NONE',  ( 6.932735513423970097, 110.7476862821014549, 10.69584247140445044 ) ) ;
#26891=CARTESIAN_POINT ( 'NONE',  ( 6.594114490232462877, 55.93981371789855217, -6.840914352311949109 ) ) ;
#26894=CARTESIAN_POINT ( 'NONE',  ( -3.474262827703527901, 105.9648137178985650, 8.843639120294245259 ) ) ;
#26896=CARTESIAN_POINT ( 'NONE',  ( 4.622313124798831829, 36.96481371789854364, -11.61527771782809282 ) ) ;
#26898=CARTESIAN_POINT ( 'NONE',  ( 11.48171059495397728, 109.8851862821014436, 4.944772684328674117 ) ) ;
#26903=CARTESIAN_POINT ( 'NONE',  ( -13.23911966647218463, 85.44768628210142936, 8.632099005475506459 ) ) ;
#26908=CARTESIAN_POINT ( 'NONE',  ( 9.500000000000005329, 109.3101862821014549, 0.1745138560725188748 ) ) ;
#26910=CARTESIAN_POINT ( 'NONE',  ( -0.1745138560725500443, 130.0101862821014436, 12.50000000000000355 ) ) ;
#26919=CARTESIAN_POINT ( 'NONE',  ( 6.594114490232462877, 19.13981371789855146, -6.840914352311949109 ) ) ;
#26924=CARTESIAN_POINT ( 'NONE',  ( 12.53471296425189330, 29.77731371789854720, 2.311890736173451533 ) ) ;
#26926=CARTESIAN_POINT ( 'NONE',  ( 6.092822981423662299, 132.4148137178985678, 14.25334919248795096 ) ) ;
#26933=CARTESIAN_POINT ( 'NONE',  ( -8.715434833791929847, 133.4601862821014606, -8.962234695871762469 ) ) ;
#26944=CARTESIAN_POINT ( 'NONE',  ( -15.46528703574804986, 132.5976862821014493, -3.257655550457287497 ) ) ;
#26946=CARTESIAN_POINT ( 'NONE',  ( -9.465287035748065847, 123.3976862821014606, -2.064181346179273735 ) ) ;
#26948=CARTESIAN_POINT ( 'NONE',  ( -12.50000000000000355, 21.91018628210143859, -0.1745138560725492671 ) ) ;
#26952=CARTESIAN_POINT ( 'NONE',  ( 8.632099005475504683, 129.1476862821014322, 13.23911966647218996 ) ) ;
#26954=CARTESIAN_POINT ( 'NONE',  ( 2.064181346179061460, 141.9023137178985507, 9.465287035748106703 ) ) ;
#26961=CARTESIAN_POINT ( 'NONE',  ( 8.152565276336593669, 76.35231371789853938, 5.233372021372610483 ) ) ;
#26966=CARTESIAN_POINT ( 'NONE',  ( -2.660918448318005058, 82.10231371789855359, -12.46528703574811558 ) ) ;
#26968=CARTESIAN_POINT ( 'NONE',  ( -11.32995696862643875, 142.9999999999997442, 7.763613995393375156 ) ) ;
#26970=CARTESIAN_POINT ( 'NONE',  ( 8.962234695871567070, 49.03981371789854649, 8.715434833792127023 ) ) ;
#26978=CARTESIAN_POINT ( 'NONE',  ( -4.944772684328673229, 29.38518628210144712, 11.48171059495397728 ) ) ;
#26984=CARTESIAN_POINT ( 'NONE',  ( -7.228626920338836470, 90.72731371789853938, -10.49813415416005213 ) ) ;
#26988=CARTESIAN_POINT ( 'NONE',  ( -0.1745138560722442889, 54.78981371789855359, -15.50000000000000533 ) ) ;
#26992=CARTESIAN_POINT ( 'NONE',  ( -10.69584247140444866, 85.44768628210144357, 6.932735513423972762 ) ) ;
#26993=CARTESIAN_POINT ( 'NONE',  ( -14.38691631536207183, 21.33518628210144641, 5.770363421893814682 ) ) ;
#26999=CARTESIAN_POINT ( 'NONE',  ( 13.23911966647218996, 44.04768628210143788, -8.632099005475504683 ) ) ;
#27006=CARTESIAN_POINT ( 'NONE',  ( 7.228626920339068285, 25.07268628210144712, -10.49813415415989581 ) ) ;
#27008=CARTESIAN_POINT ( 'NONE',  ( -8.152565276336593669, 126.9523137178985621, -5.233372021372610483 ) ) ;
#27015=CARTESIAN_POINT ( 'NONE',  ( 0.1745138560722779009, 132.9898137178985564, 12.50000000000000355 ) ) ;
#27020=CARTESIAN_POINT ( 'NONE',  ( -2.660918448318275509, 56.69768628210145067, 12.46528703574805874 ) ) ;
#27028=CARTESIAN_POINT ( 'NONE',  ( 8.962234695871762469, 98.96018628210146062, -8.715434833791931624 ) ) ;
#27029=CARTESIAN_POINT ( 'NONE',  ( 14.25334919248795451, 19.71481371789854720, -6.092822981423661410 ) ) ;
#27036=CARTESIAN_POINT ( 'NONE',  ( -12.46528703574811558, 144.2023137178985621, 2.660918448318003726 ) ) ;
#27042=CARTESIAN_POINT ( 'NONE',  ( -13.04141134922778456, 106.8273137178985479, 8.927990412390377273 ) ) ;
#27047=CARTESIAN_POINT ( 'NONE',  ( -12.46528703574805697, 22.19768628210145067, -2.660918448318280838 ) ) ;
#27051=CARTESIAN_POINT ( 'NONE',  ( 15.50000000000000533, 100.1101862821014521, 0.1745138560725827404 ) ) ;
#27054=CARTESIAN_POINT ( 'NONE',  ( 3.796722387233379514, 61.58518628210146062, -8.710071997420127943 ) ) ;
#27058=CARTESIAN_POINT ( 'NONE',  ( 12.53471296425194836, 72.22268628210143504, -2.311890736173178418 ) ) ;
#27061=CARTESIAN_POINT ( 'NONE',  ( -9.534712964251941258, 40.02268628210144641, 1.715153634034234154 ) ) ;
#27072=CARTESIAN_POINT ( 'NONE',  ( -10.49813415416004858, 97.62731371789855928, 7.228626920338839135 ) ) ;
#27073=CARTESIAN_POINT ( 'NONE',  ( -12.53471296425194659, 113.6226862821014549, 2.311890736173176641 ) ) ;
#27079=CARTESIAN_POINT ( 'NONE',  ( 14.25334919248795451, 84.11481371789855643, -6.092822981423661410 ) ) ;
#27082=CARTESIAN_POINT ( 'NONE',  ( 3.796722387233379514, 98.38518628210145778, -8.710071997420127943 ) ) ;
#27084=CARTESIAN_POINT ( 'NONE',  ( 7.954856959092311719, 65.42731371789857064, -5.529263428287300108 ) ) ;
#27088=CARTESIAN_POINT ( 'NONE',  ( 9.500000000000005329, 121.4898137178985564, -0.1745138560723090149 ) ) ;
#27090=CARTESIAN_POINT ( 'NONE',  ( 2.660918448318002838, 22.30231371789854933, 12.46528703574811558 ) ) ;
#27092=CARTESIAN_POINT ( 'NONE',  ( 0.1745138560725515708, 88.61018628210146630, -12.50000000000000355 ) ) ;
#27098=CARTESIAN_POINT ( 'NONE',  ( -8.715434833791929847, 4.660186282101435928, -8.962234695871762469 ) ) ;
#27101=CARTESIAN_POINT ( 'NONE',  ( 5.233372021372432847, 110.7476862821014691, 8.152565276336710909 ) ) ;
#27103=CARTESIAN_POINT ( 'NONE',  ( -12.53471296425194836, 132.0226862821014606, 2.311890736173176641 ) ) ;
#27114=CARTESIAN_POINT ( 'NONE',  ( 6.594114490232462877, 28.33981371789855430, -6.840914352311949109 ) ) ;
#27119=CARTESIAN_POINT ( 'NONE',  ( -8.715434833792127023, 23.73981371789854578, 8.962234695871568846 ) ) ;
#27121=CARTESIAN_POINT ( 'NONE',  ( 8.632099005475788900, 129.2523137178985451, -13.23911966647199812 ) ) ;
#27127=CARTESIAN_POINT ( 'NONE',  ( -8.962234695871760692, 140.3601862821014379, 8.715434833791933400 ) ) ;
#27133=CARTESIAN_POINT ( 'NONE',  ( 6.932735513423970097, 129.1476862821014890, 10.69584247140445044 ) ) ;
#27137=CARTESIAN_POINT ( 'NONE',  ( 2.908627838312458636, 9.077313717898549683, -15.53471296425188442 ) ) ;
#27139=CARTESIAN_POINT ( 'NONE',  ( -6.840914352312096547, 131.1601862821014777, 6.594114490232313663 ) ) ;
#27141=CARTESIAN_POINT ( 'NONE',  ( -11.61527771782819940, 30.53518628210144570, 4.622313124798574258 ) ) ;
#27144=UNCERTAINTY_MEASURE_WITH_UNIT (LENGTH_MEASURE( 1.000000000000000082E-05 ), #6853, 'distance_accuracy_value', 'NONE');
#27148=CARTESIAN_POINT ( 'NONE',  ( -15.50000000000000533, 123.1101862821014663, -0.1745138560725808530 ) ) ;
#27150=CARTESIAN_POINT ( 'NONE',  ( -6.840914352311947333, 136.4398137178985735, -6.594114490232462877 ) ) ;
#27157=CARTESIAN_POINT ( 'NONE',  ( 3.796722387233182339, 77.21481371789855075, 8.710071997420207879 ) ) ;
#27160=CARTESIAN_POINT ( 'NONE',  ( 6.932735513424201024, 74.05231371789855643, -10.69584247140429412 ) ) ;
#27164=CARTESIAN_POINT ( 'NONE',  ( -4.944772684328424539, 54.21481371789854364, -11.48171059495408031 ) ) ;
#27168=CARTESIAN_POINT ( 'NONE',  ( 7.228626920339068285, 15.87268628210144961, -10.49813415415989581 ) ) ;
#27173=CARTESIAN_POINT ( 'NONE',  ( -4.944772684328424539, 81.81481371789855928, -11.48171059495408031 ) ) ;
#27178=CARTESIAN_POINT ( 'NONE',  ( -5.770363421894122880, 50.76481371789856212, 14.38691631536194393 ) ) ;
#27181=CARTESIAN_POINT ( 'NONE',  ( 4.944772684328679446, 89.18518628210145494, -11.48171059495397373 ) ) ;
#27182=CARTESIAN_POINT ( 'NONE',  ( -8.927990412390661490, 20.47268628210143859, 13.04141134922759804 ) ) ;
#27186=CARTESIAN_POINT ( 'NONE',  ( 13.04141134922759804, 45.77268628210144641, 8.927990412390657937 ) ) ;
#27192=CARTESIAN_POINT ( 'NONE',  ( 4.622313124798573369, 28.23518628210144854, 11.61527771782819940 ) ) ;
#27194=CARTESIAN_POINT ( 'NONE',  ( 3.796722387233182339, 132.4148137178985678, 8.710071997420207879 ) ) ;
#27198=CARTESIAN_POINT ( 'NONE',  ( 11.48171059495408208, 130.1148137178985564, -4.944772684328420986 ) ) ;
#27206=CARTESIAN_POINT ( 'NONE',  ( -8.962234695871760692, 48.36018628210145209, 8.715434833791933400 ) ) ;
#27208=B_SPLINE_CURVE_WITH_KNOTS ( 'NONE', 3,
 ( #7085, #4220, #35869, #15798, #36058, #27348, #12949, #21306, #24510, #9911, #6887, #24877, #36242, #18839, #15422, #30194, #21671, #26968, #15989, #9542, #32655, #4406, #7449, #12573 ),
 .UNSPECIFIED., .F., .F.,
 ( 4, 2, 2, 2, 2, 2, 2, 2, 2, 2, 2, 4 ),
 ( 0.01193646315038279955, 0.01204987972134695558, 0.01216329629231111160, 0.01239012943423942539, 0.01284379571809604950, 0.01375112828580929251, 0.01556579342123577854, 0.01647312598894901808, 0.01738045855666225936, 0.01919512369208874192, 0.02282445396294170009, 0.02645378423379465826 ),
 .UNSPECIFIED. ) ;
#27215=CARTESIAN_POINT ( 'NONE',  ( 12.53471296425194836, 72.22268628210143504, -2.311890736173178418 ) ) ;
#27216=CARTESIAN_POINT ( 'NONE',  ( -14.38691631536193860, 16.26481371789853370, -5.770363421894132649 ) ) ;
#27222=CARTESIAN_POINT ( 'NONE',  ( 6.594114490232462877, 9.939813717898537959, -6.840914352311949109 ) ) ;
#27229=CARTESIAN_POINT ( 'NONE',  ( 13.04141134922778988, 120.6273137178985451, -8.927990412390371944 ) ) ;
#27233=CARTESIAN_POINT ( 'NONE',  ( 6.932735513423970097, 18.74768628210143717, 10.69584247140445044 ) ) ;
#27238=CARTESIAN_POINT ( 'NONE',  ( 5.770363421893814682, 111.0351862821014635, 14.38691631536207183 ) ) ;
#27241=CARTESIAN_POINT ( 'NONE',  ( 7.954856959092191815, 36.57268628210144357, 5.529263428287477744 ) ) ;
#27245=CARTESIAN_POINT ( 'NONE',  ( 12.50000000000000355, 72.51018628210145778, 0.1745138560725507937 ) ) ;
#27248=CARTESIAN_POINT ( 'NONE',  ( 6.840914352312096547, 52.96018628210144641, -6.594114490232313663 ) ) ;
#27258=CARTESIAN_POINT ( 'NONE',  ( -4.622313124798826500, 105.9648137178985650, 11.61527771782809637 ) ) ;
#27259=CARTESIAN_POINT ( 'NONE',  ( -11.48171059495397373, 105.2851862821014493, -4.944772684328680334 ) ) ;
#27264=CARTESIAN_POINT ( 'NONE',  ( 6.092822981423662299, 68.01481371789854791, 14.25334919248795096 ) ) ;
#27267=CARTESIAN_POINT ( 'NONE',  ( -2.064181346179269738, 93.49768628210142651, 9.465287035748067623 ) ) ;
#27269=CARTESIAN_POINT ( 'NONE',  ( 6.594114490232462877, 65.13981371789854791, -6.840914352311949109 ) ) ;
#27271=CARTESIAN_POINT ( 'NONE',  ( 5.233372021372610483, 110.8523137178985252, -8.152565276336593669 ) ) ;
#27273=CARTESIAN_POINT ( 'NONE',  ( 12.53471296425189330, 38.97731371789855359, 2.311890736173451977 ) ) ;
#27274=CARTESIAN_POINT ( 'NONE',  ( 12.50000000000000355, 81.71018628210144641, 0.1745138560725507937 ) ) ;
#27280=PLANE ( 'NONE',  #12181 ) ;
#27282=CARTESIAN_POINT ( 'NONE',  ( -8.843639120294326972, 104.1351862821014720, 3.474262827703335166 ) ) ;
#27284=CARTESIAN_POINT ( 'NONE',  ( 10.69584247140445221, 136.0476862821014379, -6.932735513423970097 ) ) ;
#27285=CARTESIAN_POINT ( 'NONE',  ( -6.439089545781193635, 143.0000000000000284, 10.42254124200965748 ) ) ;
#27297=CARTESIAN_POINT ( 'NONE',  ( -6.840914352311947333, 26.03981371789855714, -6.594114490232462877 ) ) ;
#27302=CARTESIAN_POINT ( 'NONE',  ( -7.228626920338836470, 26.32731371789855146, -10.49813415416005213 ) ) ;
#27305=CARTESIAN_POINT ( 'NONE',  ( -11.08355503943118592, 127.2398137178985422, -10.83675517735179383 ) ) ;
#27312=CARTESIAN_POINT ( 'NONE',  ( 4.944772684328679446, 135.1851862821014549, -11.48171059495397373 ) ) ;
#27325=CARTESIAN_POINT ( 'NONE',  ( 5.770363421893814682, 129.4351862821014549, 14.38691631536207183 ) ) ;
#27328=CARTESIAN_POINT ( 'NONE',  ( 5.529263428287477744, 117.0726862821014294, -7.954856959092191815 ) ) ;
#27330=CARTESIAN_POINT ( 'NONE',  ( 6.932735513423970097, 18.74768628210143717, 10.69584247140445044 ) ) ;
#27333=CARTESIAN_POINT ( 'NONE',  ( -15.53471296425195369, 113.6226862821014549, 2.908627838312118019 ) ) ;
#27335=CARTESIAN_POINT ( 'NONE',  ( 8.710071997420127943, 8.685186282101437172, 3.796722387233375073 ) ) ;
#27342=CARTESIAN_POINT ( 'NONE',  ( 6.594114490232462877, 74.33981371789855075, -6.840914352311949109 ) ) ;
#27346=CARTESIAN_POINT ( 'NONE',  ( 0.1745138560722779009, 77.78981371789855359, 12.50000000000000355 ) ) ;
#27348=CARTESIAN_POINT ( 'NONE',  ( -6.693455383991767427, 142.9999999999999147, 10.84641480984770467 ) ) ;
#27350=CARTESIAN_POINT ( 'NONE',  ( 8.715434833792128799, 55.93981371789855217, -8.962234695871567070 ) ) ;
#27354=CARTESIAN_POINT ( 'NONE',  ( -7.228626920339069173, 29.67268628210144499, 10.49813415415989581 ) ) ;
#27359=CARTESIAN_POINT ( 'NONE',  ( 10.49813415416005213, 83.82731371789856212, -7.228626920338837358 ) ) ;
#27364=CARTESIAN_POINT ( 'NONE',  ( -15.50000000000000533, 61.68981371789855928, 0.1745138560722471477 ) ) ;
#27367=CARTESIAN_POINT ( 'NONE',  ( -11.48171059495397373, 77.68518628210145494, -4.944772684328680334 ) ) ;
#27368=CARTESIAN_POINT ( 'NONE',  ( 5.770363421893814682, 19.03518628210144570, 14.38691631536207183 ) ) ;
#27372=CARTESIAN_POINT ( 'NONE',  ( -14.38691631536207183, 39.73518628210145209, 5.770363421893814682 ) ) ;
#27378=CARTESIAN_POINT ( 'NONE',  ( -0.1745138560725500443, 28.81018628210144072, 12.50000000000000355 ) ) ;
#27380=CARTESIAN_POINT ( 'NONE',  ( -9.500000000000005329, 135.2898137178985394, 0.1745138560723101806 ) ) ;
#27384=CARTESIAN_POINT ( 'NONE',  ( -7.228626920338836470, 127.5273137178985792, -10.49813415416005213 ) ) ;
#27390=CARTESIAN_POINT ( 'NONE',  ( -10.49813415415989404, 31.97268628210143859, -7.228626920339069173 ) ) ;
#27398=CARTESIAN_POINT ( 'NONE',  ( 12.50000000000000355, 81.71018628210144641, 0.1745138560725507937 ) ) ;
#27399=CARTESIAN_POINT ( 'NONE',  ( 0.1745138560725837118, 134.6101862821014947, -15.50000000000000533 ) ) ;
#27405=CARTESIAN_POINT ( 'NONE',  ( 0.1745138560722779009, 142.1898137178985735, 12.50000000000000355 ) ) ;
#27411=CARTESIAN_POINT ( 'NONE',  ( -10.83675517735179028, 115.7398137178985564, 11.08355503943118947 ) ) ;
#27419=CARTESIAN_POINT ( 'NONE',  ( -8.927990412390661490, 103.2726862821014322, 13.04141134922759804 ) ) ;
#27423=CARTESIAN_POINT ( 'NONE',  ( -5.529263428287477744, 48.07268628210143646, 7.954856959092191815 ) ) ;
#27427=CARTESIAN_POINT ( 'NONE',  ( 8.715434833791931624, 73.66018628210144925, 8.962234695871760692 ) ) ;
#27430=CARTESIAN_POINT ( 'NONE',  ( -1.715153634034234598, 51.52268628210144641, -9.534712964251941258 ) ) ;
#27442=CARTESIAN_POINT ( 'NONE',  ( 4.622313124798831829, 82.96481371789856496, -11.61527771782809282 ) ) ;
#27443=CARTESIAN_POINT ( 'NONE',  ( -2.311890736173176641, 97.52268628210144641, -12.53471296425194659 ) ) ;
#27449=CARTESIAN_POINT ( 'NONE',  ( -3.257655550456946880, 63.70231371789854791, -15.46528703574811736 ) ) ;
#27453=( BOUNDED_SURFACE ( )  B_SPLINE_SURFACE ( 3, 2, ( 
 ( #26330, #9284, #3593, #11747, #366, #181, #9471, #35048, #9096, #20858, #20665, #13023, #32211, #6437, #18010, #34864, #6249, #15157, #8904, #17827, #26706, #737, #7338, #35421, #24579, #12308, #36131, #23882, #21046, #32584, #18200, #6624, #10172, #33298, #18911, #31381, #2191, #4663, #24942, #24760, #13210, #13955, #37057, #36310, #16059, #16801, #34037, #16246, #13772, #5037, #25134, #19469, #4851, #21932, #31015, #22118, #10914, #27607, #36689, #5224, #1822, #10727, #30828, #1639, #10359, #19289, #33479, #27795, #7522, #13391, #34222, #25319, #25504, #19095, #11104, #36499, #30647, #36869, #8081, #16430, #16617, #22490, #33666, #10542, #19656, #7707, #27977, #2007, #13581, #22678, #8266, #22302, #33854, #28344, #31198, #7895, #2380, #28160, #19839, #8816, #31748, #11291, #20390, #11472, #274, #5401, #14502, #5777, #14321, #20759, #458, #11650, #34775, #14687, #17725, #2748, #16981, #17356, #25875, #23042, #28898, #34588, #2933, #26058, #86, #20198, #23226, #31931, #5963, #17542, #17171, #29077, #3120, #37423, #9191, #32114, #26236, #22860, #9002, #8630, #11838, #23408, #28524, #2566, #6150, #14136, #29266, #25692, #34957, #28713, #20572, #3306, #8447, #37241, #14877, #34409, #26424, #12027, #20016, #23596, #31561, #35138, #5585, #32866, #6914, #36078, #18485, #29647, #3684, #15817, #21139, #9564, #15064, #32677, #15628, #21514, #32485, #18292, #35702, #17915, #23785, #10122, #27181, #15252, #35324, #29834, #643, #26804, #6344, #6719, #835, #12403, #3870, #23975, #15443, #26992, #1020, #12593, #24158, #21327, #9752, #30025, #6532, #4057, #1206, #35519, #32303, #33059, #12778, #12213, #35890, #24348, #9933, #7105, #29459, #3493, #18674, #26614, #30216, #9378, #4242, #18106, #27367, #1397, #20952, #12972, #24529, #13155, #19417, #28111, #27558, #22438, #16010, #33618, #31151, #22255, #33806, #25454, #7844, #19047, #30599, #5170, #10488, #36447, #4429, #22067, #4983, #10864, #21876, #7658, #25082, #7284, #24710, #37007, #16566, #4614, #36262, #19235, #1585, #33985, #7469, #30778, #4801, #18858, #10306, #24897, #33245, #33428, #16194, #27744, #2334, #30966, #19602, #21694, #16748, #1773, #13340, #2142, #13722, #16379, #10676, #25271, #27925, #30406, #36823, #1956, #13526, #36637, #8028, #28296, #13905, #31329, #11050, #11793, #29028, #11236, #34725, #39, #20151, #14454, #37373, #16935, #26010, #17123, #5914, #22625, #31698, #11425, #19970, #26379, #6098, #17307, #2882, #20342, #23361, #8769, #34912, #34173, #8217, #34542, #31513, #34357, #11604, #8402, #14274, #8581, #19792, #28848, #5725, #23179, #31884, #17493, #3072, #29219, #37193, #5357, #14642, #26192, #229, #5537, #8957, #14087, #25825, #20528, #28477, #32070, #28660, #2518, #25638, #17682, #3261, #14834, #22808, #2698, #22992, #6867, #9712, #35096, #29415, #33015, #3825, #9145, #15588, #7065, #18442, #23931, #32822, #15403, #978, #20712, #32636, #789, #12166, #12554, #21287, #11979, #23740, #6297, #15017, #26568, #18635, #35473, #9524, #29983, #1168, #597, #27141, #3640, #35278, #30175, #4015, #29604, #17870, #32255, #9336, #20905, #413, #9892, #12740, #21476, #24308, #35851, #15210, #4203, #15780, #23552, #21096, #3447, #32445, #12360, #26759, #6489, #18061, #6676, #18249, #29793, #26948, #24120, #35663, #10084, #31111, #1545, #25232, #1732, #10450, #4388, #4941, #27330, #4579, #22027, #30365, #22398, #22215, #36781, #15968, #33580, #19003, #7618, #13300, #24859, #21653, #10636, #16155, #24671, #27520, #1360, #10826, #16523, #33947, #30925, #13684, #30561, #19560, #28071, #5131, #36407, #12931, #7988, #19194, #27704, #13117, #2105, #24493, #33207, #33393, #36040, #18821, #36223, #7247, #10266, #21841, #7433, #30742, #4763, #16337, #27885, #1916, #13484, #25040, #36596, #33766 ),
 ( #7806, #19382, #37154, #2476, #17266, #14049, #19933, #2656, #13866, #34502, #11383, #25783, #14233, #5684, #23140, #34871, #5320, #25415, #20300, #37333, #22956, #25598, #37500, #19753, #31473, #8543, #36968, #20109, #11195, #11011, #16712, #17452, #34682, #31842, #8727, #5874, #28990, #3031, #25970, #22584, #8179, #11753, #31657, #34129, #14603, #23321, #26154, #28806, #11567, #2843, #14415, #31292, #187, #17080, #28435, #8912, #20487, #5497, #32025, #28259, #16896, #2291, #22769, #34317, #8363, #28619, #32592, #15164, #9478, #32404, #11938, #21054, #12122, #936, #6056, #23507, #9665, #23696, #12315, #26713, #9849, #29176, #32781, #21426, #6816, #17643, #20865, #29368, #744, #6444, #9101, #3218, #21242, #35054, #3779, #12510, #20670, #18392, #372, #18017, #15543, #6631, #18206, #14790, #29747, #3407, #14976, #27101, #29562, #3599, #26336, #23889, #26908, #29942, #6256, #35430, #15353, #32217, #17833, #26525, #24074, #555, #35240, #35619, #9291, #3969, #1125, #12690, #24263, #35806, #27282, #36177, #7020, #7207, #1312, #33161, #13638, #4716, #30877, #10781, #4900, #30319, #10031, #30697, #24994, #10223, #21986, #16294, #1498, #32968, #19148, #21611, #7758, #18958, #21797, #25188, #16482, #15732, #18588, #33718, #13444, #18779, #27842, #33531, #4533, #36363, #33350, #12880, #10411, #13073, #1873, #30130, #16109, #7386, #4343, #4162, #28028, #1685, #24812, #36551, #19339, #15923, #24447, #30513, #27473, #24629, #27660, #13260, #7573, #10592, #22172, #2061, #36741, #35995, #28575, #25742, #34087, #37294, #11156, #19709, #26111, #11525, #31614, #31433, #22729, #31248, #143, #17411, #2614, #14190, #5641, #34638, #5277, #33904, #34276, #16856, #2431, #8319, #14003, #19891, #5455, #17037, #37108, #11342, #22914, #34460, #8503, #8138, #20069, #17225, #28393, #22354, #23094, #28763, #28215, #25930, #25555, #2802, #14374, #7945, #19521, #8683, #31067, #20255, #5090, #37474, #31795, #5833, #28952, #25371, #16669, #2989, #13824, #14559, #2245, #36919, #10966, #22540, #23653, #21197, #12271, #23843, #15499, #35383, #9059, #20630, #32736, #512, #26480, #31987, #12079, #32544, #891, #11894, #35196, #15118, #34825, #3173, #27054, #6586, #32173, #14747, #9245, #17600, #12462, #35016, #20818, #32360, #8868, #6016, #14933, #23282, #23462, #29133, #6210, #29895, #21010, #9620, #11707, #6772, #17782, #26293, #9432, #3736, #6399, #699, #18161, #29325, #20445, #29702, #329, #24031, #17972, #29515, #3925, #18347, #3363, #3556, #35576, #15309, #26669, #26861, #27615, #10178, #4490, #27423, #6975, #16067, #7160, #33486, #1080, #18544, #1830, #32923, #13029, #10552, #1646, #13218, #4859, #24768, #35950, #9989, #22127, #1456, #15879, #21383, #24585, #21941, #27803, #1264, #36137, #36319, #24215, #30084, #16438, #7531, #21570, #4117, #21754, #15690, #13400, #24402, #33305, #7345, #35760, #27241, #4300, #12650, #12835, #33115, #18733, #19296, #10366, #36507, #9805, #33674, #30275, #18918, #19104, #30655, #30469, #4670, #16253, #24949, #7714, #30835, #16627, #3267, #13961, #16809, #9150, #11985, #10736, #27985, #29225, #8961, #28169, #14144, #16990, #37063, #31388, #28350, #33861, #5408, #34044, #23367, #2015, #11110, #2387, #36876, #6305, #23557, #34230, #19846, #37249, #14839, #25327, #13592, #25510, #10922, #8090, #22686, #19664, #8273, #28530, #2573, #5233, #25697, #11798, #34917, #20533, #2199, #32075, #6104, #22497, #32261, #17687, #26385, #7903, #419, #31205, #35101, #20717, #25142, #36696, #22309, #19477, #31023, #5045, #13779, #3646, #984, #6683, #20912, #33213, #33022, #9342, #15594, #24314, #15216, #6495, #17876, #27335, #7073, #1366, #21482, #4209, #21104, #10090, #18641, #29421, #15410, #3455, #36046, #29799, #18255, #32451, #30183, #15024, #12172, #23937 ),
 ( #18069, #12937, #12746, #15787, #29611, #12560, #9529, #24126, #3832, #26954, #23746, #1173, #32642, #4022, #24500, #26574, #603, #35669, #797, #26765, #18449, #12367, #9718, #21293, #35284, #32829, #6874, #29991, #27150, #35857, #9898, #21660, #35480, #4394, #25048, #36413, #10456, #10272, #16343, #13123, #4585, #24865, #15975, #33585, #7438, #30372, #7253, #33772, #36601, #10642, #13490, #22219, #7812, #19388, #27892, #27526, #24677, #4948, #7624, #1551, #30931, #16530, #28077, #22034, #18827, #36231, #21847, #30567, #33399, #1922, #19200, #19010, #16161, #27710, #4770, #1739, #30747, #13306, #21785, #1113, #27088, #21601, #4331, #29732, #18765, #6803, #3766, #33337, #35984, #32768, #9464, #23875, #3957, #12494, #18948, #36166, #9836, #32955, #12868, #15911, #924, #15148, #15531, #24060, #21227, #12679, #18378, #29929, #24249, #35793, #21413, #7008, #30119, #18577, #4150, #15341, #15721, #27271, #35607, #7376, #30307, #24435, #21039, #7195, #1298, #10020, #33150, #3586, #26698, #27459, #729, #1488, #12300, #13061, #26894, #24618, #10212, #6617, #35413, #32576, #18192, #9651, #36907, #36351, #31236, #24800, #4890, #2420, #31056, #5077, #34264, #16657, #27831, #1861, #13993, #19328, #7745, #13251, #30867, #13813, #19696, #30686, #16470, #33892, #16097, #21974, #8308, #25360, #13430, #33519, #28015, #10398, #5266, #16284, #2047, #13626, #27649, #7562, #33705, #4522, #4704, #19137, #24979, #11143, #2233, #28383, #30501, #25544, #36539, #10582, #28204, #22528, #25177, #19509, #10955, #22161, #1676, #34075, #36729, #16844, #10768, #22341, #22720, #37096, #7934, #8125, #20301, #29353, #6428, #171, #358, #23679, #11738, #34667, #726, #3393, #23308, #14399, #28790, #5859, #17628, #32011, #35040, #14962, #26696, #8712, #17249, #12106, #29158, #3201, #31824, #26509, #11550, #34854, #14777, #2827, #11922, #3016, #25956, #8529, #9275, #540, #35226, #20847, #32388, #18002, #29545, #17814, #5669, #37498, #3583, #23489, #23123, #15146, #12298, #23872, #6042, #20095, #9087, #20656, #20284, #26321, #8894, #17437, #32203, #31641, #28975, #14585, #26138, #20472, #6238, #16094, #32952, #18762, #33333, #27084, #27269, #13059, #1110, #24058, #27647, #30305, #12677, #3764, #18189, #32765, #35603, #35411, #7374, #24616, #18945, #1485, #21783, #24247, #1674, #36163, #13248, #7005, #9461, #21037, #9833, #35791, #12491, #10209, #32574, #29730, #3954, #6614, #26891, #21225, #15338, #922, #9649, #30499, #21411, #18575, #6801, #4520, #18376, #30117, #4146, #29925, #15529, #4329, #15719, #1295, #12866, #24432, #35982, #10018, #21599, #33148, #15909, #7192, #27457, #37093, #36349, #21971, #10766, #7742, #10579, #25358, #22159, #28012, #22338, #33516, #5075, #19507, #8123, #13990, #24976, #33890, #28201, #10393, #16281, #2601, #19694, #33703, #27829, #7932, #30683, #25541, #19326, #31053, #2045, #7560, #19135, #13624, #4702, #36537, #1859, #30863, #5439, #34072, #22718, #24798, #34261, #4888, #13428, #22526, #16841, #25174, #13811, #31234, #16468, #36727, #10952, #16655, #11141, #2230, #36903, #17021, #8305, #5264, #28381, #19877, #31419, #2417, #28560, #17207, #23265, #17582, #2972, #20055, #29115, #20237, #9041, #14173, #34809, #14542, #23078, #29498, #9226, #20428, #6002, #23445, #26463, #11509, #25727, #26097, #34624, #31780, #127, #5815, #11692, #8854, #31972, #28937, #3159, #14729, #26278, #310, #25914, #11876, #34998, #8668, #17955, #3346, #20613, #31600, #17765, #17397, #32153, #6193, #37280, #11327, #14914, #22897, #497, #34445, #29306, #37459, #12063, #23637, #28746, #8484, #35180, #5623, #20800, #32342, #2786, #6380, #14360, #15481, #13013, #4100, #15671, #7325, #27222, #874, #12446, #24567, #29876, #18331, #23823, #3909, #9973, #12817, #683, #32527, #36121 ),
 ( #15860, #27036, #1059, #21736, #10161, #35365, #3537, #4283, #27405, #6757, #9416, #6570, #12633, #6959, #24198, #20992, #18527, #9604, #35931, #15102, #35743, #9789, #24014, #18900, #33287, #21366, #32905, #24386, #1437, #35560, #26652, #30065, #21178, #32717, #1247, #21553, #33100, #7143, #18717, #30256, #12253, #18144, #29686, #3720, #15292, #26844, #19277, #27786, #34212, #19647, #2180, #36300, #34026, #10532, #36680, #1997, #8257, #16049, #31189, #30452, #5212, #4470, #7697, #16235, #13570, #30817, #33469, #27596, #8071, #21919, #28149, #36860, #10347, #16789, #24751, #4841, #2371, #31007, #5027, #1627, #16607, #1813, #13381, #13945, #16420, #27967, #13199, #25123, #13762, #28334, #30636, #10718, #33845, #7511, #19085, #4653, #25308, #24934, #36488, #22292, #22108, #25494, #33657, #7884, #19458, #10905, #22479, #37046, #11094, #22668, #23217, #16972, #34947, #26414, #265, #5766, #14677, #34766, #20380, #2557, #14492, #20189, #31552, #31922, #20563, #32105, #5576, #6139, #34399, #8437, #449, #17346, #3111, #17716, #11463, #11641, #8993, #23032, #20006, #12016, #26227, #34579, #25682, #14126, #17162, #28702, #19830, #29255, #3296, #14868, #23399, #23587, #8620, #35129, #31369, #5392, #28889, #28514, #37232, #31738, #2923, #2739, #11280, #22850, #14311, #25864, #37413, #26049, #76, #8808, #5953, #17532, #29066, #11828, #29825, #23776, #24340, #9180, #23966, #3861, #12204, #4233, #4047, #7097, #35314, #15435, #827, #26984, #21130, #6710, #3485, #30017, #35509, #32854, #21506, #20749, #6334, #32668, #29638, #32477, #9745, #6524, #12394, #18281, #17906, #1010, #12584, #24150, #35693, #21317, #15619, #27359, #9369, #29450, #12770, #6904, #18476, #18098, #27173, #20944, #9555, #1197, #15055, #35880, #3674, #26604, #32294, #9922, #33050, #18665, #30206, #15809, #1389, #12962, #24520, #634, #15244, #26795, #8018, #2134, #22428, #1765, #28793, #13713, #14402, #33610, #36070, #17254, #10478, #24889, #13147, #25262, #10114, #30397, #4605, #21685, #27548, #21868, #18850, #2830, #10296, #33977, #22057, #19226, #24701, #36813, #33237, #13331, #30769, #1575, #31645, #30957, #19593, #36253, #4792, #27734, #16370, #7649, #27915, #4420, #19407, #36439, #22246, #10855, #7276, #16001, #1945, #19038, #33421, #36627, #7459, #13516, #25073, #30590, #10667, #33796, #7833, #4975, #16556, #28102, #16184, #5673, #34670, #29549, #9090, #20659, #11742, #9279, #28979, #29162, #32206, #8716, #29356, #20475, #20287, #25959, #26700, #6431, #3588, #32391, #18005, #15150, #731, #35229, #23126, #17440, #21041, #3396, #31828, #12302, #32578, #23877, #11926, #20851, #14965, #26513, #5862, #6242, #26325, #174, #543, #35415, #9466, #23311, #6619, #3019, #14590, #18194, #23494, #29734, #3768, #17631, #17820, #32920, #3205, #26142, #11554, #34857, #14781, #8898, #32014, #6045, #361, #35043, #12109, #23683, #21603, #27273, #12870, #9653, #36168, #30121, #1489, #27651, #26896, #12496, #1300, #35795, #1115, #15913, #12681, #18579, #24437, #24062, #33152, #10022, #35986, #7197, #4333, #21787, #33521, #3959, #35609, #18950, #18767, #30309, #24251, #10214, #18380, #4152, #27461, #21229, #13063, #9838, #32770, #15342, #16099, #33339, #30503, #7378, #4524, #1678, #13253, #24620, #6805, #29931, #10400, #24802, #15533, #36353, #21976, #7564, #19139, #30688, #926, #27090, #21415, #32957, #15723, #7010, #16846, #5444, #17026, #28017, #28566, #19330, #30869, #22902, #2235, #25546, #2605, #33894, #34077, #19882, #7936, #4892, #34450, #37098, #19511, #10584, #24981, #2049, #16472, #4706, #14177, #31424, #25733, #8310, #37284, #31058, #8491, #11332, #20060, #13815, #16286, #27833, #16659, #5080, #13628, #1863, #13432, #36541, #10770, #22163, #33707, #25179, #7747, #36731, #22343, #28206, #25362 ),
 ( #36909, #10957, #22530, #8127, #19698, #31238, #5268, #28385, #2422, #13995, #11146, #22722, #34266, #12260, #3353, #29504, #9423, #3545, #28942, #8673, #29313, #23644, #8859, #20619, #14921, #133, #31604, #17771, #20244, #6387, #17589, #20435, #23830, #15108, #14364, #5630, #32349, #17962, #34816, #25919, #34629, #3164, #35004, #31978, #37464, #9047, #11697, #26470, #17213, #14736, #6007, #2978, #28753, #26659, #318, #23451, #503, #689, #14548, #2791, #29121, #26102, #23271, #26285, #11883, #32159, #6198, #12069, #35187, #9232, #20807, #35371, #11514, #5821, #23084, #31786, #17402, #24756, #10168, #30264, #26851, #24575, #1068, #27229, #30071, #36306, #6575, #21743, #20998, #33292, #32535, #35749, #6762, #4106, #9794, #24020, #18151, #36126, #12451, #18723, #27411, #880, #7333, #15298, #32911, #30459, #21560, #33105, #29692, #7150, #18336, #29884, #4476, #21372, #6965, #3725, #18533, #4290, #18906, #21185, #15678, #24391, #35565, #9611, #32725, #15868, #16055, #3915, #27603, #15488, #1254, #27042, #12823, #35938, #12639, #24204, #1634, #9979, #1443, #13019, #13206, #11100, #4658, #22298, #19836, #10910, #22487, #14132, #34033, #7702, #19285, #31377, #36685, #25129, #30642, #10723, #31194, #37052, #10537, #33850, #13767, #33474, #1818, #25688, #5219, #30824, #13387, #7891, #16242, #22673, #33662, #19465, #31012, #7518, #27791, #13576, #21927, #22114, #24939, #4847, #28520, #19652, #8263, #10354, #5397, #16426, #36494, #8077, #2376, #5033, #36865, #16795, #27972, #19090, #28341, #2003, #34218, #16613, #28155, #2562, #16977, #2186, #25314, #13951, #25500, #2929, #31557, #2743, #8812, #3116, #26054, #5581, #14683, #5772, #32110, #37237, #20386, #82, #8626, #15061, #32300, #5959, #29072, #8998, #12023, #34584, #11287, #11646, #20194, #17352, #23222, #28894, #34771, #31927, #17538, #14497, #26232, #270, #11833, #23404, #11468, #34953, #20568, #31744, #3490, #26420, #6144, #17167, #3302, #17721, #29262, #14872, #22855, #34405, #454, #23592, #23038, #35134, #9186, #20754, #6340, #17910, #14317, #25870, #29455, #8443, #20011, #28708, #37418, #18482, #4238, #29830, #15249, #18855, #21511, #18288, #32482, #9375, #23972, #26800, #26611, #36075, #15814, #10119, #30213, #12968, #3867, #30403, #27364, #4425, #24155, #640, #7281, #1016, #15440, #3681, #1394, #12209, #20949, #32673, #23782, #18103, #12399, #6529, #35320, #832, #24526, #12589, #9750, #35515, #21691, #29643, #26988, #21323, #9560, #33241, #33055, #21136, #6716, #32863, #35698, #6910, #30022, #4052, #15625, #9930, #27178, #12775, #1202, #24345, #35886, #7102, #18671, #1770, #16562, #13336, #19231, #1951, #13152, #33803, #10672, #25078, #13521, #4980, #22434, #34169, #4610, #24707, #19598, #36633, #22251, #24895, #36819, #19044, #30774, #7840, #36259, #19412, #10484, #10302, #16007, #16745, #33981, #31148, #8024, #5167, #28292, #2331, #25267, #21873, #7465, #11046, #30962, #33425, #13902, #22622, #25450, #28108, #10861, #2139, #13719, #30595, #37003, #8214, #4797, #16191, #27741, #19789, #31326, #16375, #36444, #27554, #22064, #1582, #33615, #7654, #27920, #14271, #20708, #409, #11601, #34720, #14637, #17678, #2695, #16932, #5722, #25822, #22989, #28844, #34539, #31693, #2878, #36, #20147, #23175, #31881, #8765, #20339, #17119, #5911, #17303, #37369, #9142, #32067, #26188, #11233, #8953, #8578, #17490, #14451, #5354, #28474, #6095, #2513, #29215, #14084, #26007, #28657, #29025, #3069, #8399, #25634, #20525, #34354, #225, #11789, #22805, #3256, #37190, #23357, #14831, #34909, #26375, #19967, #11974, #11422, #23547, #35093, #31509, #5532, #15012, #32632, #15583, #21470, #32441, #18244, #35659, #17867, #23735, #10079, #27137, #29599, #35274, #29788, #592, #33011, #18056, #3819, #9520, #29412 ),
 ( #24303, #21092, #21282, #4009, #785, #32251, #18437, #20900, #7060, #15396, #6670, #12925, #15776, #26564, #6291, #3443, #12162, #35468, #9329, #6485, #3636, #15205, #24488, #1164, #30171, #26754, #4199, #12354, #23927, #29979, #35846, #26944, #32818, #12736, #973, #12550, #9888, #24116, #18631, #9706, #6862, #36035, #27325, #1353, #21649, #22395, #33944, #24857, #15963, #24667, #30739, #25037, #10449, #27516, #36594, #27700, #16521, #33203, #4760, #22025, #30557, #36964, #16710, #27883, #13482, #30923, #7986, #19000, #7243, #33578, #4575, #1730, #7615, #13298, #19190, #16335, #1913, #36405, #10634, #22212, #33762, #7803, #33390, #19379, #4938, #16151, #25411, #10823, #28069, #1541, #25229, #2103, #13682, #36779, #18817, #30361, #19558, #4385, #31110, #13111, #5129, #7430, #28257, #2287, #36218, #10262, #13863, #21838, #8723, #17448, #16893, #11749, #5317, #22952, #20483, #11563, #23136, #14787, #34678, #8360, #19931, #32021, #37329, #25779, #31289, #11379, #31836, #183, #11191, #34497, #14411, #34126, #2472, #26332, #5869, #31469, #14045, #8539, #28432, #23317, #34314, #20105, #31653, #11007, #29171, #5680, #17261, #25594, #14599, #22581, #37150, #17075, #8176, #22766, #5493, #28614, #19751, #2651, #8906, #28802, #2838, #14228, #26150, #25966, #6932, #20295, #28986, #6052, #3027, #17639, #34866, #3215, #29556, #6626, #12310, #35423, #32213, #21237, #15159, #24069, #13211, #11932, #35050, #23884, #20860, #23691, #931, #35236, #3595, #9473, #9098, #18202, #32587, #21048, #29742, #26903, #6812, #19097, #26521, #20667, #4482, #3775, #15349, #9286, #32776, #3404, #26708, #12505, #6251, #35615, #32399, #17829, #368, #1640, #18387, #16060, #29937, #27608, #24761, #36311, #9660, #29364, #14972, #33480, #10360, #551, #21933, #7523, #30648, #4664, #16247, #23503, #12117, #6439, #18012, #739, #2008, #2382, #28525, #2567, #13582, #14137, #4852, #16431, #8448, #25321, #11105, #25693, #19470, #19657, #5402, #31016, #27978, #20017, #22679, #5038, #33668, #10543, #25135, #36690, #27796, #37242, #16983, #11292, #31382, #22861, #16618, #31563, #34410, #5586, #36870, #10729, #31199, #28161, #22303, #1823, #13392, #37058, #7708, #24943, #7896, #34038, #10915, #36500, #22119, #19290, #30829, #33855, #2192, #13773, #22491, #8082, #5225, #16802, #28345, #13956, #25505, #34223, #8267, #19840, #3121, #87, #2934, #17726, #14503, #20391, #14688, #14322, #34958, #11839, #26237, #275, #6151, #23597, #35325, #5778, #25876, #20760, #23409, #9003, #26059, #459, #20199, #31932, #20573, #37424, #32115, #11651, #11473, #17172, #17916, #35139, #32304, #9192, #6345, #29460, #3494, #26425, #23043, #8632, #12214, #29267, #34589, #15066, #23786, #26615, #3307, #12028, #14878, #644, #31749, #9379, #17543, #28899, #20953, #32486, #28714, #23227, #2749, #17357, #34776, #8817, #5964, #29078, #4430, #35703, #35892, #21695, #9753, #32678, #36263, #1398, #21329, #12404, #26805, #3871, #6721, #6533, #16011, #33246, #27560, #10123, #30407, #32867, #10307, #7285, #21877, #4058, #18107, #24711, #18486, #6915, #21140, #18859, #29649, #836, #12594, #3685, #35520, #12974, #15818, #15253, #9565, #1586, #9934, #23976, #13156, #18293, #24530, #30026, #36079, #21515, #7106, #29835, #1207, #15629, #15444, #18675, #26993, #1021, #24159, #27182, #12779, #24349, #33060, #30217, #27368, #4243, #16380, #4984, #31152, #1957, #36448, #22627, #22439, #27926, #27745, #4616, #33619, #10489, #33429, #25456, #16749, #37008, #5171, #2335, #13527, #34174, #28297, #7470, #33808, #19048, #8218, #7845, #10677, #22068, #13906, #30600, #7659, #25083, #16195, #19237, #36638, #30779, #1774, #22256, #13341, #28112, #25272, #19418, #24898, #4802, #11051, #30967, #33986, #16567, #2143, #13723, #36824, #10866, #8029 ),
 ( #19604, #30349, #33565, #15952, #27127, #1152, #13285, #18618, #7050, #12539, #30160, #13099, #18987, #29968, #15763, #33190, #15383, #21270, #7602, #24654, #12723, #32808, #27312, #35648, #30544, #15571, #1342, #4189, #26933, #24103, #32998, #3807, #36205, #1526, #4561, #10063, #963, #9694, #12913, #24292, #35836, #4373, #9877, #24477, #36023, #6848, #21638, #7233, #18807, #27505, #10249, #21825, #10438, #18424, #3997, #33377, #7416, #16136, #21458, #27688, #1715, #24841, #36392, #22011, #29777, #13667, #27870, #19177, #19919, #37136, #34303, #25583, #11181, #22754, #8347, #28419, #16322, #10622, #14217, #22567, #1902, #31458, #25767, #5481, #5118, #14033, #34114, #19739, #13472, #13852, #19548, #30908, #31277, #17065, #28603, #4928, #2640, #33749, #7789, #37319, #16697, #2459, #11369, #10811, #10996, #22941, #22383, #19367, #34487, #30726, #33933, #25024, #36581, #16510, #28057, #4749, #22201, #2092, #25217, #36768, #7974, #31096, #28245, #2275, #25399, #36949, #8165, #5305, #16883, #20791, #22751, #18137, #17946, #674, #29491, #15095, #22937, #26645, #490, #8526, #15474, #866, #20985, #17061, #15283, #29299, #3529, #32335, #27028, #34300, #12437, #11177, #24006, #8343, #26456, #34483, #6373, #12056, #14214, #19914, #35358, #37316, #35552, #35172, #23629, #29868, #32710, #31455, #5478, #9597, #21170, #14906, #28599, #25764, #12245, #23816, #9220, #2635, #9409, #17758, #6562, #11366, #32518, #29679, #20092, #31638, #6750, #3713, #26837, #18324, #3902, #6185, #3337, #1429, #21546, #18709, #24562, #30249, #16412, #10154, #12626, #7503, #7318, #27590, #18892, #4463, #12810, #16041, #27398, #35924, #4832, #27776, #10341, #6950, #4646, #4276, #30442, #21729, #1052, #24190, #1806, #35736, #13373, #9782, #15851, #24379, #33279, #13006, #4092, #21358, #1619, #32898, #13189, #18519, #30058, #24928, #15664, #36112, #10523, #24744, #36293, #27215, #21912, #9966, #33092, #22101, #33461, #19078, #1239, #30630, #16226, #36481, #7137, #33650, #7689, #19270, #30810, #5760, #11275, #25302, #31001, #25487, #33840, #17155, #13756, #37038, #5206, #13562, #22286, #31183, #1990, #2174, #7877, #28144, #8613, #37227, #25858, #27959, #37406, #36854, #5021, #25673, #20001, #16782, #16966, #22844, #34018, #25115, #22661, #28327, #10898, #2552, #28694, #2731, #22470, #14306, #16601, #8063, #20183, #11085, #34390, #11456, #19640, #19825, #5570, #2365, #13938, #31732, #8432, #34207, #19451, #10710, #8251, #31362, #36673, #23025, #34573, #5386, #31545, #28509, #14119, #9550, #20938, #32663, #14863, #17339, #35503, #29250, #3291, #2917, #35125, #15238, #11636, #23394, #28882, #8802, #3103, #70, #21124, #29060, #26788, #26410, #444, #31916, #32472, #14487, #32101, #12009, #20373, #12390, #12196, #820, #5946, #23581, #8985, #9175, #20743, #32285, #23210, #628, #26597, #18092, #6329, #26043, #34759, #17900, #258, #14672, #29445, #26222, #20557, #3480, #17526, #15049, #23769, #35309, #9363, #6517, #29632, #11823, #34940, #6132, #3668, #23959, #17709, #30012, #27543, #9741, #9918, #27354, #26978, #10108, #1191, #15430, #6704, #7455, #24695, #21863, #13140, #36248, #10291, #33416, #15996, #3853, #35688, #1758, #21679, #1005, #19030, #13325, #30585, #30200, #1570, #33232, #7270, #12579, #18276, #21501, #1384, #21312, #24884, #4601, #16180, #32848, #12956, #35875, #24516, #18661, #4227, #24146, #27729, #36431, #10474, #36065, #6895, #18470, #15804, #27168, #4042, #18846, #15613, #33044, #30391, #12766, #4413, #22051, #29818, #24334, #7092, #2498, #14258, #22242, #4788, #37179, #16734, #28281, #19405, #16921, #36620, #36807, #2320, #16361, #36992, #28095, #27911, #33604, #34341, #14072, #11220, #25621, #22792, #8386, #19956, #5343, #30765, #25066, #28645, #11035, #1940, #31498, #2682 ) ),
 .UNSPECIFIED., .T., .F., .F. ) 
 B_SPLINE_SURFACE_WITH_KNOTS ( ( 4, 3, 4 ),
 ( 3, 2, 2, 2, 2, 2, 2, 2, 2, 2, 2, 2, 2, 2, 2, 2, 2, 2, 2, 2, 2, 2, 2, 2, 2, 2, 2, 2, 2, 2, 2, 2, 2, 2, 2, 2, 2, 2, 2, 2, 2, 2, 2, 2, 2, 2, 2, 2, 2, 2, 2, 2, 2, 2, 2, 2, 2, 2, 2, 2, 2, 2, 2, 2, 2, 2, 2, 2, 2, 2, 2, 2, 2, 2, 2, 2, 2, 2, 2, 2, 2, 2, 2, 2, 2, 2, 2, 2, 2, 2, 2, 2, 2, 2, 2, 2, 2, 2, 2, 2, 2, 2, 2, 2, 2, 2, 2, 2, 2, 2, 2, 2, 2, 2, 2, 2, 2, 2, 2, 2, 2, 2, 2, 2, 2, 2, 2, 2, 2, 2, 2, 2, 2, 2, 2, 2, 2, 2, 2, 2, 2, 2, 2, 2, 2, 2, 2, 2, 2, 2, 2, 2, 2, 2, 2, 2, 2, 2, 2, 2, 2, 2, 2, 2, 2, 2, 2, 2, 2, 2, 2, 2, 2, 2, 2, 2, 2, 2, 2, 2, 2, 2, 2, 2, 2, 2, 2, 2, 2, 2, 2, 2, 2, 2, 2, 2, 2, 2, 2, 2, 2, 2, 2, 2, 2, 2, 2, 2, 2, 2, 2, 2, 2, 2, 2, 2, 2, 2, 2, 2, 2, 2, 2, 2, 2, 2, 2, 2, 2, 2, 2, 2, 2, 2, 2, 2, 2, 2, 2, 2, 3 ),
 ( 0.000000000000000000, 0.5000000000000000000, 1.000000000000000000 ),
 ( 0.000000000000000000, 0.004166666666666666609, 0.008333333333333333218, 0.01250000000000000069, 0.01666666666666666644, 0.02083333333333333218, 0.02500000000000000139, 0.02916666666666666713, 0.03333333333333333287, 0.03749999999999999861, 0.04166666666666666435, 0.04583333333333333010, 0.05000000000000000278, 0.05416666666666666852, 0.05833333333333333426, 0.06250000000000000000, 0.06666666666666666574, 0.07083333333333333148, 0.07499999999999999722, 0.07916666666666666297, 0.08333333333333332871, 0.08749999999999999445, 0.09166666666666666019, 0.09583333333333333981, 0.1000000000000000056, 0.1041666666666666713, 0.1083333333333333370, 0.1125000000000000028, 0.1166666666666666685, 0.1208333333333333343, 0.1250000000000000000, 0.1291666666666666796, 0.1333333333333333315, 0.1375000000000000111, 0.1416666666666666630, 0.1458333333333333426, 0.1499999999999999944, 0.1541666666666666741, 0.1583333333333333259, 0.1625000000000000056, 0.1666666666666666574, 0.1708333333333333370, 0.1749999999999999889, 0.1791666666666666685, 0.1833333333333333204, 0.1875000000000000000, 0.1916666666666666796, 0.1958333333333333315, 0.2000000000000000111, 0.2041666666666666630, 0.2083333333333333426, 0.2124999999999999944, 0.2166666666666666741, 0.2208333333333333259, 0.2250000000000000056, 0.2291666666666666574, 0.2333333333333333370, 0.2374999999999999889, 0.2416666666666666685, 0.2458333333333333204, 0.2500000000000000000, 0.2541666666666666519, 0.2583333333333333592, 0.2625000000000000111, 0.2666666666666666630, 0.2708333333333333148, 0.2750000000000000222, 0.2791666666666666741, 0.2833333333333333259, 0.2874999999999999778, 0.2916666666666666852, 0.2958333333333333370, 0.2999999999999999889, 0.3041666666666666408, 0.3083333333333333481, 0.3125000000000000000, 0.3166666666666666519, 0.3208333333333333592, 0.3250000000000000111, 0.3291666666666666630, 0.3333333333333333148, 0.3375000000000000222, 0.3416666666666666741, 0.3458333333333333259, 0.3499999999999999778, 0.3541666666666666852, 0.3583333333333333370, 0.3624999999999999889, 0.3666666666666666408, 0.3708333333333333481, 0.3750000000000000000, 0.3791666666666666519, 0.3833333333333333592, 0.3875000000000000111, 0.3916666666666666630, 0.3958333333333333148, 0.4000000000000000222, 0.4041666666666666741, 0.4083333333333333259, 0.4124999999999999778, 0.4166666666666666852, 0.4208333333333333370, 0.4249999999999999889, 0.4291666666666666408, 0.4333333333333333481, 0.4375000000000000000, 0.4416666666666666519, 0.4458333333333333592, 0.4500000000000000111, 0.4541666666666666630, 0.4583333333333333148, 0.4625000000000000222, 0.4666666666666666741, 0.4708333333333333259, 0.4749999999999999778, 0.4791666666666666852, 0.4833333333333333370, 0.4874999999999999889, 0.4916666666666666408, 0.4958333333333333481, 0.5000000000000000000, 0.5041666666666666519, 0.5083333333333333037, 0.5124999999999999556, 0.5166666666666667185, 0.5208333333333333703, 0.5250000000000000222, 0.5291666666666666741, 0.5333333333333333259, 0.5374999999999999778, 0.5416666666666666297, 0.5458333333333332815, 0.5500000000000000444, 0.5541666666666666963, 0.5583333333333333481, 0.5625000000000000000, 0.5666666666666666519, 0.5708333333333333037, 0.5749999999999999556, 0.5791666666666667185, 0.5833333333333333703, 0.5875000000000000222, 0.5916666666666666741, 0.5958333333333333259, 0.5999999999999999778, 0.6041666666666666297, 0.6083333333333332815, 0.6125000000000000444, 0.6166666666666666963, 0.6208333333333333481, 0.6250000000000000000, 0.6291666666666666519, 0.6333333333333333037, 0.6374999999999999556, 0.6416666666666667185, 0.6458333333333333703, 0.6500000000000000222, 0.6541666666666666741, 0.6583333333333333259, 0.6624999999999999778, 0.6666666666666666297, 0.6708333333333332815, 0.6750000000000000444, 0.6791666666666666963, 0.6833333333333333481, 0.6875000000000000000, 0.6916666666666666519, 0.6958333333333333037, 0.6999999999999999556, 0.7041666666666667185, 0.7083333333333333703, 0.7125000000000000222, 0.7166666666666666741, 0.7208333333333333259, 0.7249999999999999778, 0.7291666666666666297, 0.7333333333333332815, 0.7375000000000000444, 0.7416666666666666963, 0.7458333333333333481, 0.7500000000000000000, 0.7541666666666666519, 0.7583333333333333037, 0.7624999999999999556, 0.7666666666666667185, 0.7708333333333333703, 0.7750000000000000222, 0.7791666666666666741, 0.7833333333333333259, 0.7874999999999999778, 0.7916666666666666297, 0.7958333333333332815, 0.8000000000000000444, 0.8041666666666666963, 0.8083333333333333481, 0.8125000000000000000, 0.8166666666666666519, 0.8208333333333333037, 0.8249999999999999556, 0.8291666666666667185, 0.8333333333333333703, 0.8375000000000000222, 0.8416666666666666741, 0.8458333333333333259, 0.8499999999999999778, 0.8541666666666666297, 0.8583333333333332815, 0.8625000000000000444, 0.8666666666666666963, 0.8708333333333333481, 0.8750000000000000000, 0.8791666666666666519, 0.8833333333333333037, 0.8874999999999999556, 0.8916666666666667185, 0.8958333333333333703, 0.9000000000000000222, 0.9041666666666666741, 0.9083333333333333259, 0.9124999999999999778, 0.9166666666666666297, 0.9208333333333332815, 0.9250000000000000444, 0.9291666666666666963, 0.9333333333333333481, 0.9375000000000000000, 0.9416666666666666519, 0.9458333333333333037, 0.9499999999999999556, 0.9541666666666667185, 0.9583333333333333703, 0.9625000000000000222, 0.9666666666666666741, 0.9708333333333333259, 0.9749999999999999778, 0.9791666666666666297, 0.9833333333333332815, 0.9875000000000000444, 0.9916666666666666963, 0.9958333333333333481, 1.000000000000000000 ),
 .UNSPECIFIED. ) 
 GEOMETRIC_REPRESENTATION_ITEM ( )  RATIONAL_B_SPLINE_SURFACE ( (
 ( 1.000000000000000000, 0.9807852804032304306, 1.000000000000000000, 0.9807852804032304306, 1.000000000000000000, 0.9807852804032304306, 1.000000000000000000, 0.9807852804032304306, 1.000000000000000000, 0.9807852804032304306, 1.000000000000000000, 0.9807852804032304306, 1.000000000000000000, 0.9807852804032304306, 1.000000000000000000, 0.9807852804032304306, 1.000000000000000000, 0.9807852804032304306, 1.000000000000000000, 0.9807852804032304306, 1.000000000000000000, 0.9807852804032304306, 1.000000000000000000, 0.9807852804032304306, 1.000000000000000000, 0.9807852804032304306, 1.000000000000000000, 0.9807852804032304306, 1.000000000000000000, 0.9807852804032304306, 1.000000000000000000, 0.9807852804032304306, 1.000000000000000000, 0.9807852804032304306, 1.000000000000000000, 0.9807852804032304306, 1.000000000000000000, 0.9807852804032304306, 1.000000000000000000, 0.9807852804032304306, 1.000000000000000000, 0.9807852804032304306, 1.000000000000000000, 0.9807852804032304306, 1.000000000000000000, 0.9807852804032304306, 1.000000000000000000, 0.9807852804032304306, 1.000000000000000000, 0.9807852804032304306, 1.000000000000000000, 0.9807852804032304306, 1.000000000000000000, 0.9807852804032304306, 1.000000000000000000, 0.9807852804032304306, 1.000000000000000000, 0.9807852804032304306, 1.000000000000000000, 0.9807852804032304306, 1.000000000000000000, 0.9807852804032304306, 1.000000000000000000, 0.9807852804032304306, 1.000000000000000000, 0.9807852804032304306, 1.000000000000000000, 0.9807852804032304306, 1.000000000000000000, 0.9807852804032304306, 1.000000000000000000, 0.9807852804032304306, 1.000000000000000000, 0.9807852804032304306, 1.000000000000000000, 0.9807852804032304306, 1.000000000000000000, 0.9807852804032304306, 1.000000000000000000, 0.9807852804032304306, 1.000000000000000000, 0.9807852804032304306, 1.000000000000000000, 0.9807852804032304306, 1.000000000000000000, 0.9807852804032304306, 1.000000000000000000, 0.9807852804032304306, 1.000000000000000000, 0.9807852804032304306, 1.000000000000000000, 0.9807852804032304306, 1.000000000000000000, 0.9807852804032304306, 1.000000000000000000, 0.9807852804032304306, 1.000000000000000000, 0.9807852804032304306, 1.000000000000000000, 0.9807852804032304306, 1.000000000000000000, 0.9807852804032304306, 1.000000000000000000, 0.9807852804032304306, 1.000000000000000000, 0.9807852804032304306, 1.000000000000000000, 0.9807852804032304306, 1.000000000000000000, 0.9807852804032304306, 1.000000000000000000, 0.9807852804032304306, 1.000000000000000000, 0.9807852804032304306, 1.000000000000000000, 0.9807852804032304306, 1.000000000000000000, 0.9807852804032304306, 1.000000000000000000, 0.9807852804032304306, 1.000000000000000000, 0.9807852804032304306, 1.000000000000000000, 0.9807852804032304306, 1.000000000000000000, 0.9807852804032304306, 1.000000000000000000, 0.9807852804032304306, 1.000000000000000000, 0.9807852804032304306, 1.000000000000000000, 0.9807852804032304306, 1.000000000000000000, 0.9807852804032304306, 1.000000000000000000, 0.9807852804032304306, 1.000000000000000000, 0.9807852804032304306, 1.000000000000000000, 0.9807852804032304306, 1.000000000000000000, 0.9807852804032304306, 1.000000000000000000, 0.9807852804032304306, 1.000000000000000000, 0.9807852804032304306, 1.000000000000000000, 0.9807852804032304306, 1.000000000000000000, 0.9807852804032304306, 1.000000000000000000, 0.9807852804032304306, 1.000000000000000000, 0.9807852804032304306, 1.000000000000000000, 0.9807852804032304306, 1.000000000000000000, 0.9807852804032304306, 1.000000000000000000, 0.9807852804032304306, 1.000000000000000000, 0.9807852804032304306, 1.000000000000000000, 0.9807852804032304306, 1.000000000000000000, 0.9807852804032304306, 1.000000000000000000, 0.9807852804032304306, 1.000000000000000000, 0.9807852804032304306, 1.000000000000000000, 0.9807852804032304306, 1.000000000000000000, 0.9807852804032304306, 1.000000000000000000, 0.9807852804032304306, 1.000000000000000000, 0.9807852804032304306, 1.000000000000000000, 0.9807852804032304306, 1.000000000000000000, 0.9807852804032304306, 1.000000000000000000, 0.9807852804032304306, 1.000000000000000000, 0.9807852804032304306, 1.000000000000000000, 0.9807852804032304306, 1.000000000000000000, 0.9807852804032304306, 1.000000000000000000, 0.9807852804032304306, 1.000000000000000000, 0.9807852804032304306, 1.000000000000000000, 0.9807852804032304306, 1.000000000000000000, 0.9807852804032304306, 1.000000000000000000, 0.9807852804032304306, 1.000000000000000000, 0.9807852804032304306, 1.000000000000000000, 0.9807852804032304306, 1.000000000000000000, 0.9807852804032304306, 1.000000000000000000, 0.9807852804032304306, 1.000000000000000000, 0.9807852804032304306, 1.000000000000000000, 0.9807852804032304306, 1.000000000000000000, 0.9807852804032304306, 1.000000000000000000, 0.9807852804032304306, 1.000000000000000000, 0.9807852804032304306, 1.000000000000000000, 0.9807852804032304306, 1.000000000000000000, 0.9807852804032304306, 1.000000000000000000, 0.9807852804032304306, 1.000000000000000000, 0.9807852804032304306, 1.000000000000000000, 0.9807852804032304306, 1.000000000000000000, 0.9807852804032304306, 1.000000000000000000, 0.9807852804032304306, 1.000000000000000000, 0.9807852804032304306, 1.000000000000000000, 0.9807852804032304306, 1.000000000000000000, 0.9807852804032304306, 1.000000000000000000, 0.9807852804032304306, 1.000000000000000000, 0.9807852804032304306, 1.000000000000000000, 0.9807852804032304306, 1.000000000000000000, 0.9807852804032304306, 1.000000000000000000, 0.9807852804032304306, 1.000000000000000000, 0.9807852804032304306, 1.000000000000000000, 0.9807852804032304306, 1.000000000000000000, 0.9807852804032304306, 1.000000000000000000, 0.9807852804032304306, 1.000000000000000000, 0.9807852804032304306, 1.000000000000000000, 0.9807852804032304306, 1.000000000000000000, 0.9807852804032304306, 1.000000000000000000, 0.9807852804032304306, 1.000000000000000000, 0.9807852804032304306, 1.000000000000000000, 0.9807852804032304306, 1.000000000000000000, 0.9807852804032304306, 1.000000000000000000, 0.9807852804032304306, 1.000000000000000000, 0.9807852804032304306, 1.000000000000000000, 0.9807852804032304306, 1.000000000000000000, 0.9807852804032304306, 1.000000000000000000, 0.9807852804032304306, 1.000000000000000000, 0.9807852804032304306, 1.000000000000000000, 0.9807852804032304306, 1.000000000000000000, 0.9807852804032304306, 1.000000000000000000, 0.9807852804032304306, 1.000000000000000000, 0.9807852804032304306, 1.000000000000000000, 0.9807852804032304306, 1.000000000000000000, 0.9807852804032304306, 1.000000000000000000, 0.9807852804032304306, 1.000000000000000000, 0.9807852804032304306, 1.000000000000000000, 0.9807852804032304306, 1.000000000000000000, 0.9807852804032304306, 1.000000000000000000, 0.9807852804032304306, 1.000000000000000000, 0.9807852804032304306, 1.000000000000000000, 0.9807852804032304306, 1.000000000000000000, 0.9807852804032304306, 1.000000000000000000, 0.9807852804032304306, 1.000000000000000000, 0.9807852804032304306, 1.000000000000000000, 0.9807852804032304306, 1.000000000000000000, 0.9807852804032304306, 1.000000000000000000, 0.9807852804032304306, 1.000000000000000000, 0.9807852804032304306, 1.000000000000000000, 0.9807852804032304306, 1.000000000000000000, 0.9807852804032304306, 1.000000000000000000, 0.9807852804032304306, 1.000000000000000000, 0.9807852804032304306, 1.000000000000000000, 0.9807852804032304306, 1.000000000000000000, 0.9807852804032304306, 1.000000000000000000, 0.9807852804032304306, 1.000000000000000000, 0.9807852804032304306, 1.000000000000000000, 0.9807852804032304306, 1.000000000000000000, 0.9807852804032304306, 1.000000000000000000, 0.9807852804032304306, 1.000000000000000000, 0.9807852804032304306, 1.000000000000000000, 0.9807852804032304306, 1.000000000000000000, 0.9807852804032304306, 1.000000000000000000, 0.9807852804032304306, 1.000000000000000000, 0.9807852804032304306, 1.000000000000000000, 0.9807852804032304306, 1.000000000000000000, 0.9807852804032304306, 1.000000000000000000, 0.9807852804032304306, 1.000000000000000000, 0.9807852804032304306, 1.000000000000000000, 0.9807852804032304306, 1.000000000000000000, 0.9807852804032304306, 1.000000000000000000, 0.9807852804032304306, 1.000000000000000000, 0.9807852804032304306, 1.000000000000000000, 0.9807852804032304306, 1.000000000000000000, 0.9807852804032304306, 1.000000000000000000, 0.9807852804032304306, 1.000000000000000000, 0.9807852804032304306, 1.000000000000000000, 0.9807852804032304306, 1.000000000000000000, 0.9807852804032304306, 1.000000000000000000, 0.9807852804032304306, 1.000000000000000000, 0.9807852804032304306, 1.000000000000000000, 0.9807852804032304306, 1.000000000000000000, 0.9807852804032304306, 1.000000000000000000, 0.9807852804032304306, 1.000000000000000000, 0.9807852804032304306, 1.000000000000000000, 0.9807852804032304306, 1.000000000000000000, 0.9807852804032304306, 1.000000000000000000, 0.9807852804032304306, 1.000000000000000000, 0.9807852804032304306, 1.000000000000000000, 0.9807852804032304306, 1.000000000000000000, 0.9807852804032304306, 1.000000000000000000, 0.9807852804032304306, 1.000000000000000000, 0.9807852804032304306, 1.000000000000000000, 0.9807852804032304306, 1.000000000000000000, 0.9807852804032304306, 1.000000000000000000, 0.9807852804032304306, 1.000000000000000000, 0.9807852804032304306, 1.000000000000000000, 0.9807852804032304306, 1.000000000000000000, 0.9807852804032304306, 1.000000000000000000, 0.9807852804032304306, 1.000000000000000000, 0.9807852804032304306, 1.000000000000000000, 0.9807852804032304306, 1.000000000000000000, 0.9807852804032304306, 1.000000000000000000, 0.9807852804032304306, 1.000000000000000000, 0.9807852804032304306, 1.000000000000000000, 0.9807852804032304306, 1.000000000000000000, 0.9807852804032304306, 1.000000000000000000, 0.9807852804032304306, 1.000000000000000000, 0.9807852804032304306, 1.000000000000000000, 0.9807852804032304306, 1.000000000000000000, 0.9807852804032304306, 1.000000000000000000, 0.9807852804032304306, 1.000000000000000000, 0.9807852804032304306, 1.000000000000000000, 0.9807852804032304306, 1.000000000000000000, 0.9807852804032304306, 1.000000000000000000, 0.9807852804032304306, 1.000000000000000000, 0.9807852804032304306, 1.000000000000000000, 0.9807852804032304306, 1.000000000000000000, 0.9807852804032304306, 1.000000000000000000, 0.9807852804032304306, 1.000000000000000000, 0.9807852804032304306, 1.000000000000000000, 0.9807852804032304306, 1.000000000000000000, 0.9807852804032304306, 1.000000000000000000, 0.9807852804032304306, 1.000000000000000000, 0.9807852804032304306, 1.000000000000000000, 0.9807852804032304306, 1.000000000000000000, 0.9807852804032304306, 1.000000000000000000, 0.9807852804032304306, 1.000000000000000000),
 ( 0.3333333333333333703, 0.3269284268010768657, 0.3333333333333333703, 0.3269284268010768657, 0.3333333333333333703, 0.3269284268010768657, 0.3333333333333333703, 0.3269284268010768657, 0.3333333333333333703, 0.3269284268010768657, 0.3333333333333333703, 0.3269284268010768657, 0.3333333333333333703, 0.3269284268010768657, 0.3333333333333333703, 0.3269284268010768657, 0.3333333333333333703, 0.3269284268010768657, 0.3333333333333333703, 0.3269284268010768657, 0.3333333333333333703, 0.3269284268010768657, 0.3333333333333333703, 0.3269284268010768657, 0.3333333333333333703, 0.3269284268010768657, 0.3333333333333333703, 0.3269284268010768657, 0.3333333333333333703, 0.3269284268010768657, 0.3333333333333333703, 0.3269284268010768657, 0.3333333333333333703, 0.3269284268010768657, 0.3333333333333333703, 0.3269284268010768657, 0.3333333333333333703, 0.3269284268010768657, 0.3333333333333333703, 0.3269284268010768657, 0.3333333333333333703, 0.3269284268010768657, 0.3333333333333333703, 0.3269284268010768657, 0.3333333333333333703, 0.3269284268010768657, 0.3333333333333333703, 0.3269284268010768657, 0.3333333333333333703, 0.3269284268010768657, 0.3333333333333333703, 0.3269284268010768657, 0.3333333333333333703, 0.3269284268010768657, 0.3333333333333333703, 0.3269284268010768657, 0.3333333333333333703, 0.3269284268010768657, 0.3333333333333333703, 0.3269284268010768657, 0.3333333333333333703, 0.3269284268010768657, 0.3333333333333333703, 0.3269284268010768657, 0.3333333333333333703, 0.3269284268010768657, 0.3333333333333333703, 0.3269284268010768657, 0.3333333333333333703, 0.3269284268010768657, 0.3333333333333333703, 0.3269284268010768657, 0.3333333333333333703, 0.3269284268010768657, 0.3333333333333333703, 0.3269284268010768657, 0.3333333333333333703, 0.3269284268010768657, 0.3333333333333333703, 0.3269284268010768657, 0.3333333333333333703, 0.3269284268010768657, 0.3333333333333333703, 0.3269284268010768657, 0.3333333333333333703, 0.3269284268010768657, 0.3333333333333333703, 0.3269284268010768657, 0.3333333333333333703, 0.3269284268010768657, 0.3333333333333333703, 0.3269284268010768657, 0.3333333333333333703, 0.3269284268010768657, 0.3333333333333333703, 0.3269284268010768657, 0.3333333333333333703, 0.3269284268010768657, 0.3333333333333333703, 0.3269284268010768657, 0.3333333333333333703, 0.3269284268010768657, 0.3333333333333333703, 0.3269284268010768657, 0.3333333333333333703, 0.3269284268010768657, 0.3333333333333333703, 0.3269284268010768657, 0.3333333333333333703, 0.3269284268010768657, 0.3333333333333333703, 0.3269284268010768657, 0.3333333333333333703, 0.3269284268010768657, 0.3333333333333333703, 0.3269284268010768657, 0.3333333333333333703, 0.3269284268010768657, 0.3333333333333333703, 0.3269284268010768657, 0.3333333333333333703, 0.3269284268010768657, 0.3333333333333333703, 0.3269284268010768657, 0.3333333333333333703, 0.3269284268010768657, 0.3333333333333333703, 0.3269284268010768657, 0.3333333333333333703, 0.3269284268010768657, 0.3333333333333333703, 0.3269284268010768657, 0.3333333333333333703, 0.3269284268010768657, 0.3333333333333333703, 0.3269284268010768657, 0.3333333333333333703, 0.3269284268010768657, 0.3333333333333333703, 0.3269284268010768657, 0.3333333333333333703, 0.3269284268010768657, 0.3333333333333333703, 0.3269284268010768657, 0.3333333333333333703, 0.3269284268010768657, 0.3333333333333333703, 0.3269284268010768657, 0.3333333333333333703, 0.3269284268010768657, 0.3333333333333333703, 0.3269284268010768657, 0.3333333333333333703, 0.3269284268010768657, 0.3333333333333333703, 0.3269284268010768657, 0.3333333333333333703, 0.3269284268010768657, 0.3333333333333333703, 0.3269284268010768657, 0.3333333333333333703, 0.3269284268010768657, 0.3333333333333333703, 0.3269284268010768657, 0.3333333333333333703, 0.3269284268010768657, 0.3333333333333333703, 0.3269284268010768657, 0.3333333333333333703, 0.3269284268010768657, 0.3333333333333333703, 0.3269284268010768657, 0.3333333333333333703, 0.3269284268010768657, 0.3333333333333333703, 0.3269284268010768657, 0.3333333333333333703, 0.3269284268010768657, 0.3333333333333333703, 0.3269284268010768657, 0.3333333333333333703, 0.3269284268010768657, 0.3333333333333333703, 0.3269284268010768657, 0.3333333333333333703, 0.3269284268010768657, 0.3333333333333333703, 0.3269284268010768657, 0.3333333333333333703, 0.3269284268010768657, 0.3333333333333333703, 0.3269284268010768657, 0.3333333333333333703, 0.3269284268010768657, 0.3333333333333333703, 0.3269284268010768657, 0.3333333333333333703, 0.3269284268010768657, 0.3333333333333333703, 0.3269284268010768657, 0.3333333333333333703, 0.3269284268010768657, 0.3333333333333333703, 0.3269284268010768657, 0.3333333333333333703, 0.3269284268010768657, 0.3333333333333333703, 0.3269284268010768657, 0.3333333333333333703, 0.3269284268010768657, 0.3333333333333333703, 0.3269284268010768657, 0.3333333333333333703, 0.3269284268010768657, 0.3333333333333333703, 0.3269284268010768657, 0.3333333333333333703, 0.3269284268010768657, 0.3333333333333333703, 0.3269284268010768657, 0.3333333333333333703, 0.3269284268010768657, 0.3333333333333333703, 0.3269284268010768657, 0.3333333333333333703, 0.3269284268010768657, 0.3333333333333333703, 0.3269284268010768657, 0.3333333333333333703, 0.3269284268010768657, 0.3333333333333333703, 0.3269284268010768657, 0.3333333333333333703, 0.3269284268010768657, 0.3333333333333333703, 0.3269284268010768657, 0.3333333333333333703, 0.3269284268010768657, 0.3333333333333333703, 0.3269284268010768657, 0.3333333333333333703, 0.3269284268010768657, 0.3333333333333333703, 0.3269284268010768657, 0.3333333333333333703, 0.3269284268010768657, 0.3333333333333333703, 0.3269284268010768657, 0.3333333333333333703, 0.3269284268010768657, 0.3333333333333333703, 0.3269284268010768657, 0.3333333333333333703, 0.3269284268010768657, 0.3333333333333333703, 0.3269284268010768657, 0.3333333333333333703, 0.3269284268010768657, 0.3333333333333333703, 0.3269284268010768657, 0.3333333333333333703, 0.3269284268010768657, 0.3333333333333333703, 0.3269284268010768657, 0.3333333333333333703, 0.3269284268010768657, 0.3333333333333333703, 0.3269284268010768657, 0.3333333333333333703, 0.3269284268010768657, 0.3333333333333333703, 0.3269284268010768657, 0.3333333333333333703, 0.3269284268010768657, 0.3333333333333333703, 0.3269284268010768657, 0.3333333333333333703, 0.3269284268010768657, 0.3333333333333333703, 0.3269284268010768657, 0.3333333333333333703, 0.3269284268010768657, 0.3333333333333333703, 0.3269284268010768657, 0.3333333333333333703, 0.3269284268010768657, 0.3333333333333333703, 0.3269284268010768657, 0.3333333333333333703, 0.3269284268010768657, 0.3333333333333333703, 0.3269284268010768657, 0.3333333333333333703, 0.3269284268010768657, 0.3333333333333333703, 0.3269284268010768657, 0.3333333333333333703, 0.3269284268010768657, 0.3333333333333333703, 0.3269284268010768657, 0.3333333333333333703, 0.3269284268010768657, 0.3333333333333333703, 0.3269284268010768657, 0.3333333333333333703, 0.3269284268010768657, 0.3333333333333333703, 0.3269284268010768657, 0.3333333333333333703, 0.3269284268010768657, 0.3333333333333333703, 0.3269284268010768657, 0.3333333333333333703, 0.3269284268010768657, 0.3333333333333333703, 0.3269284268010768657, 0.3333333333333333703, 0.3269284268010768657, 0.3333333333333333703, 0.3269284268010768657, 0.3333333333333333703, 0.3269284268010768657, 0.3333333333333333703, 0.3269284268010768657, 0.3333333333333333703, 0.3269284268010768657, 0.3333333333333333703, 0.3269284268010768657, 0.3333333333333333703, 0.3269284268010768657, 0.3333333333333333703, 0.3269284268010768657, 0.3333333333333333703, 0.3269284268010768657, 0.3333333333333333703, 0.3269284268010768657, 0.3333333333333333703, 0.3269284268010768657, 0.3333333333333333703, 0.3269284268010768657, 0.3333333333333333703, 0.3269284268010768657, 0.3333333333333333703, 0.3269284268010768657, 0.3333333333333333703, 0.3269284268010768657, 0.3333333333333333703, 0.3269284268010768657, 0.3333333333333333703, 0.3269284268010768657, 0.3333333333333333703, 0.3269284268010768657, 0.3333333333333333703, 0.3269284268010768657, 0.3333333333333333703, 0.3269284268010768657, 0.3333333333333333703, 0.3269284268010768657, 0.3333333333333333703, 0.3269284268010768657, 0.3333333333333333703, 0.3269284268010768657, 0.3333333333333333703, 0.3269284268010768657, 0.3333333333333333703, 0.3269284268010768657, 0.3333333333333333703, 0.3269284268010768657, 0.3333333333333333703, 0.3269284268010768657, 0.3333333333333333703, 0.3269284268010768657, 0.3333333333333333703, 0.3269284268010768657, 0.3333333333333333703, 0.3269284268010768657, 0.3333333333333333703, 0.3269284268010768657, 0.3333333333333333703, 0.3269284268010768657, 0.3333333333333333703, 0.3269284268010768657, 0.3333333333333333703, 0.3269284268010768657, 0.3333333333333333703, 0.3269284268010768657, 0.3333333333333333703, 0.3269284268010768657, 0.3333333333333333703, 0.3269284268010768657, 0.3333333333333333703, 0.3269284268010768657, 0.3333333333333333703, 0.3269284268010768657, 0.3333333333333333703, 0.3269284268010768657, 0.3333333333333333703, 0.3269284268010768657, 0.3333333333333333703, 0.3269284268010768657, 0.3333333333333333703, 0.3269284268010768657, 0.3333333333333333703, 0.3269284268010768657, 0.3333333333333333703, 0.3269284268010768657, 0.3333333333333333703, 0.3269284268010768657, 0.3333333333333333703, 0.3269284268010768657, 0.3333333333333333703, 0.3269284268010768657, 0.3333333333333333703, 0.3269284268010768657, 0.3333333333333333703, 0.3269284268010768657, 0.3333333333333333703, 0.3269284268010768657, 0.3333333333333333703, 0.3269284268010768657, 0.3333333333333333703, 0.3269284268010768657, 0.3333333333333333703, 0.3269284268010768657, 0.3333333333333333703, 0.3269284268010768657, 0.3333333333333333703, 0.3269284268010768657, 0.3333333333333333703, 0.3269284268010768657, 0.3333333333333333703, 0.3269284268010768657, 0.3333333333333333703, 0.3269284268010768657, 0.3333333333333333703, 0.3269284268010768657, 0.3333333333333333703, 0.3269284268010768657, 0.3333333333333333703, 0.3269284268010768657, 0.3333333333333333703, 0.3269284268010768657, 0.3333333333333333703, 0.3269284268010768657, 0.3333333333333333703, 0.3269284268010768657, 0.3333333333333333703, 0.3269284268010768657, 0.3333333333333333703, 0.3269284268010768657, 0.3333333333333333703, 0.3269284268010768657, 0.3333333333333333703, 0.3269284268010768657, 0.3333333333333333703, 0.3269284268010768657, 0.3333333333333333703, 0.3269284268010768657, 0.3333333333333333703, 0.3269284268010768657, 0.3333333333333333703, 0.3269284268010768657, 0.3333333333333333703, 0.3269284268010768657, 0.3333333333333333703, 0.3269284268010768657, 0.3333333333333333703, 0.3269284268010768657, 0.3333333333333333703, 0.3269284268010768657, 0.3333333333333333703, 0.3269284268010768657, 0.3333333333333333703, 0.3269284268010768657, 0.3333333333333333703, 0.3269284268010768657, 0.3333333333333333703, 0.3269284268010768657, 0.3333333333333333703, 0.3269284268010768657, 0.3333333333333333703),
 ( 0.3333333333333333703, 0.3269284268010768657, 0.3333333333333333703, 0.3269284268010768657, 0.3333333333333333703, 0.3269284268010768657, 0.3333333333333333703, 0.3269284268010768657, 0.3333333333333333703, 0.3269284268010768657, 0.3333333333333333703, 0.3269284268010768657, 0.3333333333333333703, 0.3269284268010768657, 0.3333333333333333703, 0.3269284268010768657, 0.3333333333333333703, 0.3269284268010768657, 0.3333333333333333703, 0.3269284268010768657, 0.3333333333333333703, 0.3269284268010768657, 0.3333333333333333703, 0.3269284268010768657, 0.3333333333333333703, 0.3269284268010768657, 0.3333333333333333703, 0.3269284268010768657, 0.3333333333333333703, 0.3269284268010768657, 0.3333333333333333703, 0.3269284268010768657, 0.3333333333333333703, 0.3269284268010768657, 0.3333333333333333703, 0.3269284268010768657, 0.3333333333333333703, 0.3269284268010768657, 0.3333333333333333703, 0.3269284268010768657, 0.3333333333333333703, 0.3269284268010768657, 0.3333333333333333703, 0.3269284268010768657, 0.3333333333333333703, 0.3269284268010768657, 0.3333333333333333703, 0.3269284268010768657, 0.3333333333333333703, 0.3269284268010768657, 0.3333333333333333703, 0.3269284268010768657, 0.3333333333333333703, 0.3269284268010768657, 0.3333333333333333703, 0.3269284268010768657, 0.3333333333333333703, 0.3269284268010768657, 0.3333333333333333703, 0.3269284268010768657, 0.3333333333333333703, 0.3269284268010768657, 0.3333333333333333703, 0.3269284268010768657, 0.3333333333333333703, 0.3269284268010768657, 0.3333333333333333703, 0.3269284268010768657, 0.3333333333333333703, 0.3269284268010768657, 0.3333333333333333703, 0.3269284268010768657, 0.3333333333333333703, 0.3269284268010768657, 0.3333333333333333703, 0.3269284268010768657, 0.3333333333333333703, 0.3269284268010768657, 0.3333333333333333703, 0.3269284268010768657, 0.3333333333333333703, 0.3269284268010768657, 0.3333333333333333703, 0.3269284268010768657, 0.3333333333333333703, 0.3269284268010768657, 0.3333333333333333703, 0.3269284268010768657, 0.3333333333333333703, 0.3269284268010768657, 0.3333333333333333703, 0.3269284268010768657, 0.3333333333333333703, 0.3269284268010768657, 0.3333333333333333703, 0.3269284268010768657, 0.3333333333333333703, 0.3269284268010768657, 0.3333333333333333703, 0.3269284268010768657, 0.3333333333333333703, 0.3269284268010768657, 0.3333333333333333703, 0.3269284268010768657, 0.3333333333333333703, 0.3269284268010768657, 0.3333333333333333703, 0.3269284268010768657, 0.3333333333333333703, 0.3269284268010768657, 0.3333333333333333703, 0.3269284268010768657, 0.3333333333333333703, 0.3269284268010768657, 0.3333333333333333703, 0.3269284268010768657, 0.3333333333333333703, 0.3269284268010768657, 0.3333333333333333703, 0.3269284268010768657, 0.3333333333333333703, 0.3269284268010768657, 0.3333333333333333703, 0.3269284268010768657, 0.3333333333333333703, 0.3269284268010768657, 0.3333333333333333703, 0.3269284268010768657, 0.3333333333333333703, 0.3269284268010768657, 0.3333333333333333703, 0.3269284268010768657, 0.3333333333333333703, 0.3269284268010768657, 0.3333333333333333703, 0.3269284268010768657, 0.3333333333333333703, 0.3269284268010768657, 0.3333333333333333703, 0.3269284268010768657, 0.3333333333333333703, 0.3269284268010768657, 0.3333333333333333703, 0.3269284268010768657, 0.3333333333333333703, 0.3269284268010768657, 0.3333333333333333703, 0.3269284268010768657, 0.3333333333333333703, 0.3269284268010768657, 0.3333333333333333703, 0.3269284268010768657, 0.3333333333333333703, 0.3269284268010768657, 0.3333333333333333703, 0.3269284268010768657, 0.3333333333333333703, 0.3269284268010768657, 0.3333333333333333703, 0.3269284268010768657, 0.3333333333333333703, 0.3269284268010768657, 0.3333333333333333703, 0.3269284268010768657, 0.3333333333333333703, 0.3269284268010768657, 0.3333333333333333703, 0.3269284268010768657, 0.3333333333333333703, 0.3269284268010768657, 0.3333333333333333703, 0.3269284268010768657, 0.3333333333333333703, 0.3269284268010768657, 0.3333333333333333703, 0.3269284268010768657, 0.3333333333333333703, 0.3269284268010768657, 0.3333333333333333703, 0.3269284268010768657, 0.3333333333333333703, 0.3269284268010768657, 0.3333333333333333703, 0.3269284268010768657, 0.3333333333333333703, 0.3269284268010768657, 0.3333333333333333703, 0.3269284268010768657, 0.3333333333333333703, 0.3269284268010768657, 0.3333333333333333703, 0.3269284268010768657, 0.3333333333333333703, 0.3269284268010768657, 0.3333333333333333703, 0.3269284268010768657, 0.3333333333333333703, 0.3269284268010768657, 0.3333333333333333703, 0.3269284268010768657, 0.3333333333333333703, 0.3269284268010768657, 0.3333333333333333703, 0.3269284268010768657, 0.3333333333333333703, 0.3269284268010768657, 0.3333333333333333703, 0.3269284268010768657, 0.3333333333333333703, 0.3269284268010768657, 0.3333333333333333703, 0.3269284268010768657, 0.3333333333333333703, 0.3269284268010768657, 0.3333333333333333703, 0.3269284268010768657, 0.3333333333333333703, 0.3269284268010768657, 0.3333333333333333703, 0.3269284268010768657, 0.3333333333333333703, 0.3269284268010768657, 0.3333333333333333703, 0.3269284268010768657, 0.3333333333333333703, 0.3269284268010768657, 0.3333333333333333703, 0.3269284268010768657, 0.3333333333333333703, 0.3269284268010768657, 0.3333333333333333703, 0.3269284268010768657, 0.3333333333333333703, 0.3269284268010768657, 0.3333333333333333703, 0.3269284268010768657, 0.3333333333333333703, 0.3269284268010768657, 0.3333333333333333703, 0.3269284268010768657, 0.3333333333333333703, 0.3269284268010768657, 0.3333333333333333703, 0.3269284268010768657, 0.3333333333333333703, 0.3269284268010768657, 0.3333333333333333703, 0.3269284268010768657, 0.3333333333333333703, 0.3269284268010768657, 0.3333333333333333703, 0.3269284268010768657, 0.3333333333333333703, 0.3269284268010768657, 0.3333333333333333703, 0.3269284268010768657, 0.3333333333333333703, 0.3269284268010768657, 0.3333333333333333703, 0.3269284268010768657, 0.3333333333333333703, 0.3269284268010768657, 0.3333333333333333703, 0.3269284268010768657, 0.3333333333333333703, 0.3269284268010768657, 0.3333333333333333703, 0.3269284268010768657, 0.3333333333333333703, 0.3269284268010768657, 0.3333333333333333703, 0.3269284268010768657, 0.3333333333333333703, 0.3269284268010768657, 0.3333333333333333703, 0.3269284268010768657, 0.3333333333333333703, 0.3269284268010768657, 0.3333333333333333703, 0.3269284268010768657, 0.3333333333333333703, 0.3269284268010768657, 0.3333333333333333703, 0.3269284268010768657, 0.3333333333333333703, 0.3269284268010768657, 0.3333333333333333703, 0.3269284268010768657, 0.3333333333333333703, 0.3269284268010768657, 0.3333333333333333703, 0.3269284268010768657, 0.3333333333333333703, 0.3269284268010768657, 0.3333333333333333703, 0.3269284268010768657, 0.3333333333333333703, 0.3269284268010768657, 0.3333333333333333703, 0.3269284268010768657, 0.3333333333333333703, 0.3269284268010768657, 0.3333333333333333703, 0.3269284268010768657, 0.3333333333333333703, 0.3269284268010768657, 0.3333333333333333703, 0.3269284268010768657, 0.3333333333333333703, 0.3269284268010768657, 0.3333333333333333703, 0.3269284268010768657, 0.3333333333333333703, 0.3269284268010768657, 0.3333333333333333703, 0.3269284268010768657, 0.3333333333333333703, 0.3269284268010768657, 0.3333333333333333703, 0.3269284268010768657, 0.3333333333333333703, 0.3269284268010768657, 0.3333333333333333703, 0.3269284268010768657, 0.3333333333333333703, 0.3269284268010768657, 0.3333333333333333703, 0.3269284268010768657, 0.3333333333333333703, 0.3269284268010768657, 0.3333333333333333703, 0.3269284268010768657, 0.3333333333333333703, 0.3269284268010768657, 0.3333333333333333703, 0.3269284268010768657, 0.3333333333333333703, 0.3269284268010768657, 0.3333333333333333703, 0.3269284268010768657, 0.3333333333333333703, 0.3269284268010768657, 0.3333333333333333703, 0.3269284268010768657, 0.3333333333333333703, 0.3269284268010768657, 0.3333333333333333703, 0.3269284268010768657, 0.3333333333333333703, 0.3269284268010768657, 0.3333333333333333703, 0.3269284268010768657, 0.3333333333333333703, 0.3269284268010768657, 0.3333333333333333703, 0.3269284268010768657, 0.3333333333333333703, 0.3269284268010768657, 0.3333333333333333703, 0.3269284268010768657, 0.3333333333333333703, 0.3269284268010768657, 0.3333333333333333703, 0.3269284268010768657, 0.3333333333333333703, 0.3269284268010768657, 0.3333333333333333703, 0.3269284268010768657, 0.3333333333333333703, 0.3269284268010768657, 0.3333333333333333703, 0.3269284268010768657, 0.3333333333333333703, 0.3269284268010768657, 0.3333333333333333703, 0.3269284268010768657, 0.3333333333333333703, 0.3269284268010768657, 0.3333333333333333703, 0.3269284268010768657, 0.3333333333333333703, 0.3269284268010768657, 0.3333333333333333703, 0.3269284268010768657, 0.3333333333333333703, 0.3269284268010768657, 0.3333333333333333703, 0.3269284268010768657, 0.3333333333333333703, 0.3269284268010768657, 0.3333333333333333703, 0.3269284268010768657, 0.3333333333333333703, 0.3269284268010768657, 0.3333333333333333703, 0.3269284268010768657, 0.3333333333333333703, 0.3269284268010768657, 0.3333333333333333703, 0.3269284268010768657, 0.3333333333333333703, 0.3269284268010768657, 0.3333333333333333703, 0.3269284268010768657, 0.3333333333333333703, 0.3269284268010768657, 0.3333333333333333703, 0.3269284268010768657, 0.3333333333333333703, 0.3269284268010768657, 0.3333333333333333703, 0.3269284268010768657, 0.3333333333333333703, 0.3269284268010768657, 0.3333333333333333703, 0.3269284268010768657, 0.3333333333333333703, 0.3269284268010768657, 0.3333333333333333703, 0.3269284268010768657, 0.3333333333333333703, 0.3269284268010768657, 0.3333333333333333703, 0.3269284268010768657, 0.3333333333333333703, 0.3269284268010768657, 0.3333333333333333703, 0.3269284268010768657, 0.3333333333333333703, 0.3269284268010768657, 0.3333333333333333703, 0.3269284268010768657, 0.3333333333333333703, 0.3269284268010768657, 0.3333333333333333703, 0.3269284268010768657, 0.3333333333333333703, 0.3269284268010768657, 0.3333333333333333703, 0.3269284268010768657, 0.3333333333333333703, 0.3269284268010768657, 0.3333333333333333703, 0.3269284268010768657, 0.3333333333333333703, 0.3269284268010768657, 0.3333333333333333703, 0.3269284268010768657, 0.3333333333333333703, 0.3269284268010768657, 0.3333333333333333703, 0.3269284268010768657, 0.3333333333333333703, 0.3269284268010768657, 0.3333333333333333703, 0.3269284268010768657, 0.3333333333333333703, 0.3269284268010768657, 0.3333333333333333703, 0.3269284268010768657, 0.3333333333333333703, 0.3269284268010768657, 0.3333333333333333703, 0.3269284268010768657, 0.3333333333333333703, 0.3269284268010768657, 0.3333333333333333703, 0.3269284268010768657, 0.3333333333333333703, 0.3269284268010768657, 0.3333333333333333703, 0.3269284268010768657, 0.3333333333333333703, 0.3269284268010768657, 0.3333333333333333703, 0.3269284268010768657, 0.3333333333333333703, 0.3269284268010768657, 0.3333333333333333703, 0.3269284268010768657, 0.3333333333333333703),
 ( 1.000000000000000000, 0.9807852804032304306, 1.000000000000000000, 0.9807852804032304306, 1.000000000000000000, 0.9807852804032304306, 1.000000000000000000, 0.9807852804032304306, 1.000000000000000000, 0.9807852804032304306, 1.000000000000000000, 0.9807852804032304306, 1.000000000000000000, 0.9807852804032304306, 1.000000000000000000, 0.9807852804032304306, 1.000000000000000000, 0.9807852804032304306, 1.000000000000000000, 0.9807852804032304306, 1.000000000000000000, 0.9807852804032304306, 1.000000000000000000, 0.9807852804032304306, 1.000000000000000000, 0.9807852804032304306, 1.000000000000000000, 0.9807852804032304306, 1.000000000000000000, 0.9807852804032304306, 1.000000000000000000, 0.9807852804032304306, 1.000000000000000000, 0.9807852804032304306, 1.000000000000000000, 0.9807852804032304306, 1.000000000000000000, 0.9807852804032304306, 1.000000000000000000, 0.9807852804032304306, 1.000000000000000000, 0.9807852804032304306, 1.000000000000000000, 0.9807852804032304306, 1.000000000000000000, 0.9807852804032304306, 1.000000000000000000, 0.9807852804032304306, 1.000000000000000000, 0.9807852804032304306, 1.000000000000000000, 0.9807852804032304306, 1.000000000000000000, 0.9807852804032304306, 1.000000000000000000, 0.9807852804032304306, 1.000000000000000000, 0.9807852804032304306, 1.000000000000000000, 0.9807852804032304306, 1.000000000000000000, 0.9807852804032304306, 1.000000000000000000, 0.9807852804032304306, 1.000000000000000000, 0.9807852804032304306, 1.000000000000000000, 0.9807852804032304306, 1.000000000000000000, 0.9807852804032304306, 1.000000000000000000, 0.9807852804032304306, 1.000000000000000000, 0.9807852804032304306, 1.000000000000000000, 0.9807852804032304306, 1.000000000000000000, 0.9807852804032304306, 1.000000000000000000, 0.9807852804032304306, 1.000000000000000000, 0.9807852804032304306, 1.000000000000000000, 0.9807852804032304306, 1.000000000000000000, 0.9807852804032304306, 1.000000000000000000, 0.9807852804032304306, 1.000000000000000000, 0.9807852804032304306, 1.000000000000000000, 0.9807852804032304306, 1.000000000000000000, 0.9807852804032304306, 1.000000000000000000, 0.9807852804032304306, 1.000000000000000000, 0.9807852804032304306, 1.000000000000000000, 0.9807852804032304306, 1.000000000000000000, 0.9807852804032304306, 1.000000000000000000, 0.9807852804032304306, 1.000000000000000000, 0.9807852804032304306, 1.000000000000000000, 0.9807852804032304306, 1.000000000000000000, 0.9807852804032304306, 1.000000000000000000, 0.9807852804032304306, 1.000000000000000000, 0.9807852804032304306, 1.000000000000000000, 0.9807852804032304306, 1.000000000000000000, 0.9807852804032304306, 1.000000000000000000, 0.9807852804032304306, 1.000000000000000000, 0.9807852804032304306, 1.000000000000000000, 0.9807852804032304306, 1.000000000000000000, 0.9807852804032304306, 1.000000000000000000, 0.9807852804032304306, 1.000000000000000000, 0.9807852804032304306, 1.000000000000000000, 0.9807852804032304306, 1.000000000000000000, 0.9807852804032304306, 1.000000000000000000, 0.9807852804032304306, 1.000000000000000000, 0.9807852804032304306, 1.000000000000000000, 0.9807852804032304306, 1.000000000000000000, 0.9807852804032304306, 1.000000000000000000, 0.9807852804032304306, 1.000000000000000000, 0.9807852804032304306, 1.000000000000000000, 0.9807852804032304306, 1.000000000000000000, 0.9807852804032304306, 1.000000000000000000, 0.9807852804032304306, 1.000000000000000000, 0.9807852804032304306, 1.000000000000000000, 0.9807852804032304306, 1.000000000000000000, 0.9807852804032304306, 1.000000000000000000, 0.9807852804032304306, 1.000000000000000000, 0.9807852804032304306, 1.000000000000000000, 0.9807852804032304306, 1.000000000000000000, 0.9807852804032304306, 1.000000000000000000, 0.9807852804032304306, 1.000000000000000000, 0.9807852804032304306, 1.000000000000000000, 0.9807852804032304306, 1.000000000000000000, 0.9807852804032304306, 1.000000000000000000, 0.9807852804032304306, 1.000000000000000000, 0.9807852804032304306, 1.000000000000000000, 0.9807852804032304306, 1.000000000000000000, 0.9807852804032304306, 1.000000000000000000, 0.9807852804032304306, 1.000000000000000000, 0.9807852804032304306, 1.000000000000000000, 0.9807852804032304306, 1.000000000000000000, 0.9807852804032304306, 1.000000000000000000, 0.9807852804032304306, 1.000000000000000000, 0.9807852804032304306, 1.000000000000000000, 0.9807852804032304306, 1.000000000000000000, 0.9807852804032304306, 1.000000000000000000, 0.9807852804032304306, 1.000000000000000000, 0.9807852804032304306, 1.000000000000000000, 0.9807852804032304306, 1.000000000000000000, 0.9807852804032304306, 1.000000000000000000, 0.9807852804032304306, 1.000000000000000000, 0.9807852804032304306, 1.000000000000000000, 0.9807852804032304306, 1.000000000000000000, 0.9807852804032304306, 1.000000000000000000, 0.9807852804032304306, 1.000000000000000000, 0.9807852804032304306, 1.000000000000000000, 0.9807852804032304306, 1.000000000000000000, 0.9807852804032304306, 1.000000000000000000, 0.9807852804032304306, 1.000000000000000000, 0.9807852804032304306, 1.000000000000000000, 0.9807852804032304306, 1.000000000000000000, 0.9807852804032304306, 1.000000000000000000, 0.9807852804032304306, 1.000000000000000000, 0.9807852804032304306, 1.000000000000000000, 0.9807852804032304306, 1.000000000000000000, 0.9807852804032304306, 1.000000000000000000, 0.9807852804032304306, 1.000000000000000000, 0.9807852804032304306, 1.000000000000000000, 0.9807852804032304306, 1.000000000000000000, 0.9807852804032304306, 1.000000000000000000, 0.9807852804032304306, 1.000000000000000000, 0.9807852804032304306, 1.000000000000000000, 0.9807852804032304306, 1.000000000000000000, 0.9807852804032304306, 1.000000000000000000, 0.9807852804032304306, 1.000000000000000000, 0.9807852804032304306, 1.000000000000000000, 0.9807852804032304306, 1.000000000000000000, 0.9807852804032304306, 1.000000000000000000, 0.9807852804032304306, 1.000000000000000000, 0.9807852804032304306, 1.000000000000000000, 0.9807852804032304306, 1.000000000000000000, 0.9807852804032304306, 1.000000000000000000, 0.9807852804032304306, 1.000000000000000000, 0.9807852804032304306, 1.000000000000000000, 0.9807852804032304306, 1.000000000000000000, 0.9807852804032304306, 1.000000000000000000, 0.9807852804032304306, 1.000000000000000000, 0.9807852804032304306, 1.000000000000000000, 0.9807852804032304306, 1.000000000000000000, 0.9807852804032304306, 1.000000000000000000, 0.9807852804032304306, 1.000000000000000000, 0.9807852804032304306, 1.000000000000000000, 0.9807852804032304306, 1.000000000000000000, 0.9807852804032304306, 1.000000000000000000, 0.9807852804032304306, 1.000000000000000000, 0.9807852804032304306, 1.000000000000000000, 0.9807852804032304306, 1.000000000000000000, 0.9807852804032304306, 1.000000000000000000, 0.9807852804032304306, 1.000000000000000000, 0.9807852804032304306, 1.000000000000000000, 0.9807852804032304306, 1.000000000000000000, 0.9807852804032304306, 1.000000000000000000, 0.9807852804032304306, 1.000000000000000000, 0.9807852804032304306, 1.000000000000000000, 0.9807852804032304306, 1.000000000000000000, 0.9807852804032304306, 1.000000000000000000, 0.9807852804032304306, 1.000000000000000000, 0.9807852804032304306, 1.000000000000000000, 0.9807852804032304306, 1.000000000000000000, 0.9807852804032304306, 1.000000000000000000, 0.9807852804032304306, 1.000000000000000000, 0.9807852804032304306, 1.000000000000000000, 0.9807852804032304306, 1.000000000000000000, 0.9807852804032304306, 1.000000000000000000, 0.9807852804032304306, 1.000000000000000000, 0.9807852804032304306, 1.000000000000000000, 0.9807852804032304306, 1.000000000000000000, 0.9807852804032304306, 1.000000000000000000, 0.9807852804032304306, 1.000000000000000000, 0.9807852804032304306, 1.000000000000000000, 0.9807852804032304306, 1.000000000000000000, 0.9807852804032304306, 1.000000000000000000, 0.9807852804032304306, 1.000000000000000000, 0.9807852804032304306, 1.000000000000000000, 0.9807852804032304306, 1.000000000000000000, 0.9807852804032304306, 1.000000000000000000, 0.9807852804032304306, 1.000000000000000000, 0.9807852804032304306, 1.000000000000000000, 0.9807852804032304306, 1.000000000000000000, 0.9807852804032304306, 1.000000000000000000, 0.9807852804032304306, 1.000000000000000000, 0.9807852804032304306, 1.000000000000000000, 0.9807852804032304306, 1.000000000000000000, 0.9807852804032304306, 1.000000000000000000, 0.9807852804032304306, 1.000000000000000000, 0.9807852804032304306, 1.000000000000000000, 0.9807852804032304306, 1.000000000000000000, 0.9807852804032304306, 1.000000000000000000, 0.9807852804032304306, 1.000000000000000000, 0.9807852804032304306, 1.000000000000000000, 0.9807852804032304306, 1.000000000000000000, 0.9807852804032304306, 1.000000000000000000, 0.9807852804032304306, 1.000000000000000000, 0.9807852804032304306, 1.000000000000000000, 0.9807852804032304306, 1.000000000000000000, 0.9807852804032304306, 1.000000000000000000, 0.9807852804032304306, 1.000000000000000000, 0.9807852804032304306, 1.000000000000000000, 0.9807852804032304306, 1.000000000000000000, 0.9807852804032304306, 1.000000000000000000, 0.9807852804032304306, 1.000000000000000000, 0.9807852804032304306, 1.000000000000000000, 0.9807852804032304306, 1.000000000000000000, 0.9807852804032304306, 1.000000000000000000, 0.9807852804032304306, 1.000000000000000000, 0.9807852804032304306, 1.000000000000000000, 0.9807852804032304306, 1.000000000000000000, 0.9807852804032304306, 1.000000000000000000, 0.9807852804032304306, 1.000000000000000000, 0.9807852804032304306, 1.000000000000000000, 0.9807852804032304306, 1.000000000000000000, 0.9807852804032304306, 1.000000000000000000, 0.9807852804032304306, 1.000000000000000000, 0.9807852804032304306, 1.000000000000000000, 0.9807852804032304306, 1.000000000000000000, 0.9807852804032304306, 1.000000000000000000, 0.9807852804032304306, 1.000000000000000000, 0.9807852804032304306, 1.000000000000000000, 0.9807852804032304306, 1.000000000000000000, 0.9807852804032304306, 1.000000000000000000, 0.9807852804032304306, 1.000000000000000000, 0.9807852804032304306, 1.000000000000000000, 0.9807852804032304306, 1.000000000000000000, 0.9807852804032304306, 1.000000000000000000, 0.9807852804032304306, 1.000000000000000000, 0.9807852804032304306, 1.000000000000000000, 0.9807852804032304306, 1.000000000000000000, 0.9807852804032304306, 1.000000000000000000, 0.9807852804032304306, 1.000000000000000000, 0.9807852804032304306, 1.000000000000000000, 0.9807852804032304306, 1.000000000000000000, 0.9807852804032304306, 1.000000000000000000, 0.9807852804032304306, 1.000000000000000000, 0.9807852804032304306, 1.000000000000000000, 0.9807852804032304306, 1.000000000000000000, 0.9807852804032304306, 1.000000000000000000, 0.9807852804032304306, 1.000000000000000000),
 ( 0.3333333333333333703, 0.3269284268010768657, 0.3333333333333333703, 0.3269284268010768657, 0.3333333333333333703, 0.3269284268010768657, 0.3333333333333333703, 0.3269284268010768657, 0.3333333333333333703, 0.3269284268010768657, 0.3333333333333333703, 0.3269284268010768657, 0.3333333333333333703, 0.3269284268010768657, 0.3333333333333333703, 0.3269284268010768657, 0.3333333333333333703, 0.3269284268010768657, 0.3333333333333333703, 0.3269284268010768657, 0.3333333333333333703, 0.3269284268010768657, 0.3333333333333333703, 0.3269284268010768657, 0.3333333333333333703, 0.3269284268010768657, 0.3333333333333333703, 0.3269284268010768657, 0.3333333333333333703, 0.3269284268010768657, 0.3333333333333333703, 0.3269284268010768657, 0.3333333333333333703, 0.3269284268010768657, 0.3333333333333333703, 0.3269284268010768657, 0.3333333333333333703, 0.3269284268010768657, 0.3333333333333333703, 0.3269284268010768657, 0.3333333333333333703, 0.3269284268010768657, 0.3333333333333333703, 0.3269284268010768657, 0.3333333333333333703, 0.3269284268010768657, 0.3333333333333333703, 0.3269284268010768657, 0.3333333333333333703, 0.3269284268010768657, 0.3333333333333333703, 0.3269284268010768657, 0.3333333333333333703, 0.3269284268010768657, 0.3333333333333333703, 0.3269284268010768657, 0.3333333333333333703, 0.3269284268010768657, 0.3333333333333333703, 0.3269284268010768657, 0.3333333333333333703, 0.3269284268010768657, 0.3333333333333333703, 0.3269284268010768657, 0.3333333333333333703, 0.3269284268010768657, 0.3333333333333333703, 0.3269284268010768657, 0.3333333333333333703, 0.3269284268010768657, 0.3333333333333333703, 0.3269284268010768657, 0.3333333333333333703, 0.3269284268010768657, 0.3333333333333333703, 0.3269284268010768657, 0.3333333333333333703, 0.3269284268010768657, 0.3333333333333333703, 0.3269284268010768657, 0.3333333333333333703, 0.3269284268010768657, 0.3333333333333333703, 0.3269284268010768657, 0.3333333333333333703, 0.3269284268010768657, 0.3333333333333333703, 0.3269284268010768657, 0.3333333333333333703, 0.3269284268010768657, 0.3333333333333333703, 0.3269284268010768657, 0.3333333333333333703, 0.3269284268010768657, 0.3333333333333333703, 0.3269284268010768657, 0.3333333333333333703, 0.3269284268010768657, 0.3333333333333333703, 0.3269284268010768657, 0.3333333333333333703, 0.3269284268010768657, 0.3333333333333333703, 0.3269284268010768657, 0.3333333333333333703, 0.3269284268010768657, 0.3333333333333333703, 0.3269284268010768657, 0.3333333333333333703, 0.3269284268010768657, 0.3333333333333333703, 0.3269284268010768657, 0.3333333333333333703, 0.3269284268010768657, 0.3333333333333333703, 0.3269284268010768657, 0.3333333333333333703, 0.3269284268010768657, 0.3333333333333333703, 0.3269284268010768657, 0.3333333333333333703, 0.3269284268010768657, 0.3333333333333333703, 0.3269284268010768657, 0.3333333333333333703, 0.3269284268010768657, 0.3333333333333333703, 0.3269284268010768657, 0.3333333333333333703, 0.3269284268010768657, 0.3333333333333333703, 0.3269284268010768657, 0.3333333333333333703, 0.3269284268010768657, 0.3333333333333333703, 0.3269284268010768657, 0.3333333333333333703, 0.3269284268010768657, 0.3333333333333333703, 0.3269284268010768657, 0.3333333333333333703, 0.3269284268010768657, 0.3333333333333333703, 0.3269284268010768657, 0.3333333333333333703, 0.3269284268010768657, 0.3333333333333333703, 0.3269284268010768657, 0.3333333333333333703, 0.3269284268010768657, 0.3333333333333333703, 0.3269284268010768657, 0.3333333333333333703, 0.3269284268010768657, 0.3333333333333333703, 0.3269284268010768657, 0.3333333333333333703, 0.3269284268010768657, 0.3333333333333333703, 0.3269284268010768657, 0.3333333333333333703, 0.3269284268010768657, 0.3333333333333333703, 0.3269284268010768657, 0.3333333333333333703, 0.3269284268010768657, 0.3333333333333333703, 0.3269284268010768657, 0.3333333333333333703, 0.3269284268010768657, 0.3333333333333333703, 0.3269284268010768657, 0.3333333333333333703, 0.3269284268010768657, 0.3333333333333333703, 0.3269284268010768657, 0.3333333333333333703, 0.3269284268010768657, 0.3333333333333333703, 0.3269284268010768657, 0.3333333333333333703, 0.3269284268010768657, 0.3333333333333333703, 0.3269284268010768657, 0.3333333333333333703, 0.3269284268010768657, 0.3333333333333333703, 0.3269284268010768657, 0.3333333333333333703, 0.3269284268010768657, 0.3333333333333333703, 0.3269284268010768657, 0.3333333333333333703, 0.3269284268010768657, 0.3333333333333333703, 0.3269284268010768657, 0.3333333333333333703, 0.3269284268010768657, 0.3333333333333333703, 0.3269284268010768657, 0.3333333333333333703, 0.3269284268010768657, 0.3333333333333333703, 0.3269284268010768657, 0.3333333333333333703, 0.3269284268010768657, 0.3333333333333333703, 0.3269284268010768657, 0.3333333333333333703, 0.3269284268010768657, 0.3333333333333333703, 0.3269284268010768657, 0.3333333333333333703, 0.3269284268010768657, 0.3333333333333333703, 0.3269284268010768657, 0.3333333333333333703, 0.3269284268010768657, 0.3333333333333333703, 0.3269284268010768657, 0.3333333333333333703, 0.3269284268010768657, 0.3333333333333333703, 0.3269284268010768657, 0.3333333333333333703, 0.3269284268010768657, 0.3333333333333333703, 0.3269284268010768657, 0.3333333333333333703, 0.3269284268010768657, 0.3333333333333333703, 0.3269284268010768657, 0.3333333333333333703, 0.3269284268010768657, 0.3333333333333333703, 0.3269284268010768657, 0.3333333333333333703, 0.3269284268010768657, 0.3333333333333333703, 0.3269284268010768657, 0.3333333333333333703, 0.3269284268010768657, 0.3333333333333333703, 0.3269284268010768657, 0.3333333333333333703, 0.3269284268010768657, 0.3333333333333333703, 0.3269284268010768657, 0.3333333333333333703, 0.3269284268010768657, 0.3333333333333333703, 0.3269284268010768657, 0.3333333333333333703, 0.3269284268010768657, 0.3333333333333333703, 0.3269284268010768657, 0.3333333333333333703, 0.3269284268010768657, 0.3333333333333333703, 0.3269284268010768657, 0.3333333333333333703, 0.3269284268010768657, 0.3333333333333333703, 0.3269284268010768657, 0.3333333333333333703, 0.3269284268010768657, 0.3333333333333333703, 0.3269284268010768657, 0.3333333333333333703, 0.3269284268010768657, 0.3333333333333333703, 0.3269284268010768657, 0.3333333333333333703, 0.3269284268010768657, 0.3333333333333333703, 0.3269284268010768657, 0.3333333333333333703, 0.3269284268010768657, 0.3333333333333333703, 0.3269284268010768657, 0.3333333333333333703, 0.3269284268010768657, 0.3333333333333333703, 0.3269284268010768657, 0.3333333333333333703, 0.3269284268010768657, 0.3333333333333333703, 0.3269284268010768657, 0.3333333333333333703, 0.3269284268010768657, 0.3333333333333333703, 0.3269284268010768657, 0.3333333333333333703, 0.3269284268010768657, 0.3333333333333333703, 0.3269284268010768657, 0.3333333333333333703, 0.3269284268010768657, 0.3333333333333333703, 0.3269284268010768657, 0.3333333333333333703, 0.3269284268010768657, 0.3333333333333333703, 0.3269284268010768657, 0.3333333333333333703, 0.3269284268010768657, 0.3333333333333333703, 0.3269284268010768657, 0.3333333333333333703, 0.3269284268010768657, 0.3333333333333333703, 0.3269284268010768657, 0.3333333333333333703, 0.3269284268010768657, 0.3333333333333333703, 0.3269284268010768657, 0.3333333333333333703, 0.3269284268010768657, 0.3333333333333333703, 0.3269284268010768657, 0.3333333333333333703, 0.3269284268010768657, 0.3333333333333333703, 0.3269284268010768657, 0.3333333333333333703, 0.3269284268010768657, 0.3333333333333333703, 0.3269284268010768657, 0.3333333333333333703, 0.3269284268010768657, 0.3333333333333333703, 0.3269284268010768657, 0.3333333333333333703, 0.3269284268010768657, 0.3333333333333333703, 0.3269284268010768657, 0.3333333333333333703, 0.3269284268010768657, 0.3333333333333333703, 0.3269284268010768657, 0.3333333333333333703, 0.3269284268010768657, 0.3333333333333333703, 0.3269284268010768657, 0.3333333333333333703, 0.3269284268010768657, 0.3333333333333333703, 0.3269284268010768657, 0.3333333333333333703, 0.3269284268010768657, 0.3333333333333333703, 0.3269284268010768657, 0.3333333333333333703, 0.3269284268010768657, 0.3333333333333333703, 0.3269284268010768657, 0.3333333333333333703, 0.3269284268010768657, 0.3333333333333333703, 0.3269284268010768657, 0.3333333333333333703, 0.3269284268010768657, 0.3333333333333333703, 0.3269284268010768657, 0.3333333333333333703, 0.3269284268010768657, 0.3333333333333333703, 0.3269284268010768657, 0.3333333333333333703, 0.3269284268010768657, 0.3333333333333333703, 0.3269284268010768657, 0.3333333333333333703, 0.3269284268010768657, 0.3333333333333333703, 0.3269284268010768657, 0.3333333333333333703, 0.3269284268010768657, 0.3333333333333333703, 0.3269284268010768657, 0.3333333333333333703, 0.3269284268010768657, 0.3333333333333333703, 0.3269284268010768657, 0.3333333333333333703, 0.3269284268010768657, 0.3333333333333333703, 0.3269284268010768657, 0.3333333333333333703, 0.3269284268010768657, 0.3333333333333333703, 0.3269284268010768657, 0.3333333333333333703, 0.3269284268010768657, 0.3333333333333333703, 0.3269284268010768657, 0.3333333333333333703, 0.3269284268010768657, 0.3333333333333333703, 0.3269284268010768657, 0.3333333333333333703, 0.3269284268010768657, 0.3333333333333333703, 0.3269284268010768657, 0.3333333333333333703, 0.3269284268010768657, 0.3333333333333333703, 0.3269284268010768657, 0.3333333333333333703, 0.3269284268010768657, 0.3333333333333333703, 0.3269284268010768657, 0.3333333333333333703, 0.3269284268010768657, 0.3333333333333333703, 0.3269284268010768657, 0.3333333333333333703, 0.3269284268010768657, 0.3333333333333333703, 0.3269284268010768657, 0.3333333333333333703, 0.3269284268010768657, 0.3333333333333333703, 0.3269284268010768657, 0.3333333333333333703, 0.3269284268010768657, 0.3333333333333333703, 0.3269284268010768657, 0.3333333333333333703, 0.3269284268010768657, 0.3333333333333333703, 0.3269284268010768657, 0.3333333333333333703, 0.3269284268010768657, 0.3333333333333333703, 0.3269284268010768657, 0.3333333333333333703, 0.3269284268010768657, 0.3333333333333333703, 0.3269284268010768657, 0.3333333333333333703, 0.3269284268010768657, 0.3333333333333333703, 0.3269284268010768657, 0.3333333333333333703, 0.3269284268010768657, 0.3333333333333333703, 0.3269284268010768657, 0.3333333333333333703, 0.3269284268010768657, 0.3333333333333333703, 0.3269284268010768657, 0.3333333333333333703, 0.3269284268010768657, 0.3333333333333333703, 0.3269284268010768657, 0.3333333333333333703, 0.3269284268010768657, 0.3333333333333333703, 0.3269284268010768657, 0.3333333333333333703, 0.3269284268010768657, 0.3333333333333333703, 0.3269284268010768657, 0.3333333333333333703, 0.3269284268010768657, 0.3333333333333333703, 0.3269284268010768657, 0.3333333333333333703, 0.3269284268010768657, 0.3333333333333333703, 0.3269284268010768657, 0.3333333333333333703, 0.3269284268010768657, 0.3333333333333333703, 0.3269284268010768657, 0.3333333333333333703, 0.3269284268010768657, 0.3333333333333333703, 0.3269284268010768657, 0.3333333333333333703),
 ( 0.3333333333333333703, 0.3269284268010768657, 0.3333333333333333703, 0.3269284268010768657, 0.3333333333333333703, 0.3269284268010768657, 0.3333333333333333703, 0.3269284268010768657, 0.3333333333333333703, 0.3269284268010768657, 0.3333333333333333703, 0.3269284268010768657, 0.3333333333333333703, 0.3269284268010768657, 0.3333333333333333703, 0.3269284268010768657, 0.3333333333333333703, 0.3269284268010768657, 0.3333333333333333703, 0.3269284268010768657, 0.3333333333333333703, 0.3269284268010768657, 0.3333333333333333703, 0.3269284268010768657, 0.3333333333333333703, 0.3269284268010768657, 0.3333333333333333703, 0.3269284268010768657, 0.3333333333333333703, 0.3269284268010768657, 0.3333333333333333703, 0.3269284268010768657, 0.3333333333333333703, 0.3269284268010768657, 0.3333333333333333703, 0.3269284268010768657, 0.3333333333333333703, 0.3269284268010768657, 0.3333333333333333703, 0.3269284268010768657, 0.3333333333333333703, 0.3269284268010768657, 0.3333333333333333703, 0.3269284268010768657, 0.3333333333333333703, 0.3269284268010768657, 0.3333333333333333703, 0.3269284268010768657, 0.3333333333333333703, 0.3269284268010768657, 0.3333333333333333703, 0.3269284268010768657, 0.3333333333333333703, 0.3269284268010768657, 0.3333333333333333703, 0.3269284268010768657, 0.3333333333333333703, 0.3269284268010768657, 0.3333333333333333703, 0.3269284268010768657, 0.3333333333333333703, 0.3269284268010768657, 0.3333333333333333703, 0.3269284268010768657, 0.3333333333333333703, 0.3269284268010768657, 0.3333333333333333703, 0.3269284268010768657, 0.3333333333333333703, 0.3269284268010768657, 0.3333333333333333703, 0.3269284268010768657, 0.3333333333333333703, 0.3269284268010768657, 0.3333333333333333703, 0.3269284268010768657, 0.3333333333333333703, 0.3269284268010768657, 0.3333333333333333703, 0.3269284268010768657, 0.3333333333333333703, 0.3269284268010768657, 0.3333333333333333703, 0.3269284268010768657, 0.3333333333333333703, 0.3269284268010768657, 0.3333333333333333703, 0.3269284268010768657, 0.3333333333333333703, 0.3269284268010768657, 0.3333333333333333703, 0.3269284268010768657, 0.3333333333333333703, 0.3269284268010768657, 0.3333333333333333703, 0.3269284268010768657, 0.3333333333333333703, 0.3269284268010768657, 0.3333333333333333703, 0.3269284268010768657, 0.3333333333333333703, 0.3269284268010768657, 0.3333333333333333703, 0.3269284268010768657, 0.3333333333333333703, 0.3269284268010768657, 0.3333333333333333703, 0.3269284268010768657, 0.3333333333333333703, 0.3269284268010768657, 0.3333333333333333703, 0.3269284268010768657, 0.3333333333333333703, 0.3269284268010768657, 0.3333333333333333703, 0.3269284268010768657, 0.3333333333333333703, 0.3269284268010768657, 0.3333333333333333703, 0.3269284268010768657, 0.3333333333333333703, 0.3269284268010768657, 0.3333333333333333703, 0.3269284268010768657, 0.3333333333333333703, 0.3269284268010768657, 0.3333333333333333703, 0.3269284268010768657, 0.3333333333333333703, 0.3269284268010768657, 0.3333333333333333703, 0.3269284268010768657, 0.3333333333333333703, 0.3269284268010768657, 0.3333333333333333703, 0.3269284268010768657, 0.3333333333333333703, 0.3269284268010768657, 0.3333333333333333703, 0.3269284268010768657, 0.3333333333333333703, 0.3269284268010768657, 0.3333333333333333703, 0.3269284268010768657, 0.3333333333333333703, 0.3269284268010768657, 0.3333333333333333703, 0.3269284268010768657, 0.3333333333333333703, 0.3269284268010768657, 0.3333333333333333703, 0.3269284268010768657, 0.3333333333333333703, 0.3269284268010768657, 0.3333333333333333703, 0.3269284268010768657, 0.3333333333333333703, 0.3269284268010768657, 0.3333333333333333703, 0.3269284268010768657, 0.3333333333333333703, 0.3269284268010768657, 0.3333333333333333703, 0.3269284268010768657, 0.3333333333333333703, 0.3269284268010768657, 0.3333333333333333703, 0.3269284268010768657, 0.3333333333333333703, 0.3269284268010768657, 0.3333333333333333703, 0.3269284268010768657, 0.3333333333333333703, 0.3269284268010768657, 0.3333333333333333703, 0.3269284268010768657, 0.3333333333333333703, 0.3269284268010768657, 0.3333333333333333703, 0.3269284268010768657, 0.3333333333333333703, 0.3269284268010768657, 0.3333333333333333703, 0.3269284268010768657, 0.3333333333333333703, 0.3269284268010768657, 0.3333333333333333703, 0.3269284268010768657, 0.3333333333333333703, 0.3269284268010768657, 0.3333333333333333703, 0.3269284268010768657, 0.3333333333333333703, 0.3269284268010768657, 0.3333333333333333703, 0.3269284268010768657, 0.3333333333333333703, 0.3269284268010768657, 0.3333333333333333703, 0.3269284268010768657, 0.3333333333333333703, 0.3269284268010768657, 0.3333333333333333703, 0.3269284268010768657, 0.3333333333333333703, 0.3269284268010768657, 0.3333333333333333703, 0.3269284268010768657, 0.3333333333333333703, 0.3269284268010768657, 0.3333333333333333703, 0.3269284268010768657, 0.3333333333333333703, 0.3269284268010768657, 0.3333333333333333703, 0.3269284268010768657, 0.3333333333333333703, 0.3269284268010768657, 0.3333333333333333703, 0.3269284268010768657, 0.3333333333333333703, 0.3269284268010768657, 0.3333333333333333703, 0.3269284268010768657, 0.3333333333333333703, 0.3269284268010768657, 0.3333333333333333703, 0.3269284268010768657, 0.3333333333333333703, 0.3269284268010768657, 0.3333333333333333703, 0.3269284268010768657, 0.3333333333333333703, 0.3269284268010768657, 0.3333333333333333703, 0.3269284268010768657, 0.3333333333333333703, 0.3269284268010768657, 0.3333333333333333703, 0.3269284268010768657, 0.3333333333333333703, 0.3269284268010768657, 0.3333333333333333703, 0.3269284268010768657, 0.3333333333333333703, 0.3269284268010768657, 0.3333333333333333703, 0.3269284268010768657, 0.3333333333333333703, 0.3269284268010768657, 0.3333333333333333703, 0.3269284268010768657, 0.3333333333333333703, 0.3269284268010768657, 0.3333333333333333703, 0.3269284268010768657, 0.3333333333333333703, 0.3269284268010768657, 0.3333333333333333703, 0.3269284268010768657, 0.3333333333333333703, 0.3269284268010768657, 0.3333333333333333703, 0.3269284268010768657, 0.3333333333333333703, 0.3269284268010768657, 0.3333333333333333703, 0.3269284268010768657, 0.3333333333333333703, 0.3269284268010768657, 0.3333333333333333703, 0.3269284268010768657, 0.3333333333333333703, 0.3269284268010768657, 0.3333333333333333703, 0.3269284268010768657, 0.3333333333333333703, 0.3269284268010768657, 0.3333333333333333703, 0.3269284268010768657, 0.3333333333333333703, 0.3269284268010768657, 0.3333333333333333703, 0.3269284268010768657, 0.3333333333333333703, 0.3269284268010768657, 0.3333333333333333703, 0.3269284268010768657, 0.3333333333333333703, 0.3269284268010768657, 0.3333333333333333703, 0.3269284268010768657, 0.3333333333333333703, 0.3269284268010768657, 0.3333333333333333703, 0.3269284268010768657, 0.3333333333333333703, 0.3269284268010768657, 0.3333333333333333703, 0.3269284268010768657, 0.3333333333333333703, 0.3269284268010768657, 0.3333333333333333703, 0.3269284268010768657, 0.3333333333333333703, 0.3269284268010768657, 0.3333333333333333703, 0.3269284268010768657, 0.3333333333333333703, 0.3269284268010768657, 0.3333333333333333703, 0.3269284268010768657, 0.3333333333333333703, 0.3269284268010768657, 0.3333333333333333703, 0.3269284268010768657, 0.3333333333333333703, 0.3269284268010768657, 0.3333333333333333703, 0.3269284268010768657, 0.3333333333333333703, 0.3269284268010768657, 0.3333333333333333703, 0.3269284268010768657, 0.3333333333333333703, 0.3269284268010768657, 0.3333333333333333703, 0.3269284268010768657, 0.3333333333333333703, 0.3269284268010768657, 0.3333333333333333703, 0.3269284268010768657, 0.3333333333333333703, 0.3269284268010768657, 0.3333333333333333703, 0.3269284268010768657, 0.3333333333333333703, 0.3269284268010768657, 0.3333333333333333703, 0.3269284268010768657, 0.3333333333333333703, 0.3269284268010768657, 0.3333333333333333703, 0.3269284268010768657, 0.3333333333333333703, 0.3269284268010768657, 0.3333333333333333703, 0.3269284268010768657, 0.3333333333333333703, 0.3269284268010768657, 0.3333333333333333703, 0.3269284268010768657, 0.3333333333333333703, 0.3269284268010768657, 0.3333333333333333703, 0.3269284268010768657, 0.3333333333333333703, 0.3269284268010768657, 0.3333333333333333703, 0.3269284268010768657, 0.3333333333333333703, 0.3269284268010768657, 0.3333333333333333703, 0.3269284268010768657, 0.3333333333333333703, 0.3269284268010768657, 0.3333333333333333703, 0.3269284268010768657, 0.3333333333333333703, 0.3269284268010768657, 0.3333333333333333703, 0.3269284268010768657, 0.3333333333333333703, 0.3269284268010768657, 0.3333333333333333703, 0.3269284268010768657, 0.3333333333333333703, 0.3269284268010768657, 0.3333333333333333703, 0.3269284268010768657, 0.3333333333333333703, 0.3269284268010768657, 0.3333333333333333703, 0.3269284268010768657, 0.3333333333333333703, 0.3269284268010768657, 0.3333333333333333703, 0.3269284268010768657, 0.3333333333333333703, 0.3269284268010768657, 0.3333333333333333703, 0.3269284268010768657, 0.3333333333333333703, 0.3269284268010768657, 0.3333333333333333703, 0.3269284268010768657, 0.3333333333333333703, 0.3269284268010768657, 0.3333333333333333703, 0.3269284268010768657, 0.3333333333333333703, 0.3269284268010768657, 0.3333333333333333703, 0.3269284268010768657, 0.3333333333333333703, 0.3269284268010768657, 0.3333333333333333703, 0.3269284268010768657, 0.3333333333333333703, 0.3269284268010768657, 0.3333333333333333703, 0.3269284268010768657, 0.3333333333333333703, 0.3269284268010768657, 0.3333333333333333703, 0.3269284268010768657, 0.3333333333333333703, 0.3269284268010768657, 0.3333333333333333703, 0.3269284268010768657, 0.3333333333333333703, 0.3269284268010768657, 0.3333333333333333703, 0.3269284268010768657, 0.3333333333333333703, 0.3269284268010768657, 0.3333333333333333703, 0.3269284268010768657, 0.3333333333333333703, 0.3269284268010768657, 0.3333333333333333703, 0.3269284268010768657, 0.3333333333333333703, 0.3269284268010768657, 0.3333333333333333703, 0.3269284268010768657, 0.3333333333333333703, 0.3269284268010768657, 0.3333333333333333703, 0.3269284268010768657, 0.3333333333333333703, 0.3269284268010768657, 0.3333333333333333703, 0.3269284268010768657, 0.3333333333333333703, 0.3269284268010768657, 0.3333333333333333703, 0.3269284268010768657, 0.3333333333333333703, 0.3269284268010768657, 0.3333333333333333703, 0.3269284268010768657, 0.3333333333333333703, 0.3269284268010768657, 0.3333333333333333703, 0.3269284268010768657, 0.3333333333333333703, 0.3269284268010768657, 0.3333333333333333703, 0.3269284268010768657, 0.3333333333333333703, 0.3269284268010768657, 0.3333333333333333703, 0.3269284268010768657, 0.3333333333333333703, 0.3269284268010768657, 0.3333333333333333703, 0.3269284268010768657, 0.3333333333333333703, 0.3269284268010768657, 0.3333333333333333703, 0.3269284268010768657, 0.3333333333333333703, 0.3269284268010768657, 0.3333333333333333703, 0.3269284268010768657, 0.3333333333333333703, 0.3269284268010768657, 0.3333333333333333703, 0.3269284268010768657, 0.3333333333333333703),
 ( 1.000000000000000000, 0.9807852804032304306, 1.000000000000000000, 0.9807852804032304306, 1.000000000000000000, 0.9807852804032304306, 1.000000000000000000, 0.9807852804032304306, 1.000000000000000000, 0.9807852804032304306, 1.000000000000000000, 0.9807852804032304306, 1.000000000000000000, 0.9807852804032304306, 1.000000000000000000, 0.9807852804032304306, 1.000000000000000000, 0.9807852804032304306, 1.000000000000000000, 0.9807852804032304306, 1.000000000000000000, 0.9807852804032304306, 1.000000000000000000, 0.9807852804032304306, 1.000000000000000000, 0.9807852804032304306, 1.000000000000000000, 0.9807852804032304306, 1.000000000000000000, 0.9807852804032304306, 1.000000000000000000, 0.9807852804032304306, 1.000000000000000000, 0.9807852804032304306, 1.000000000000000000, 0.9807852804032304306, 1.000000000000000000, 0.9807852804032304306, 1.000000000000000000, 0.9807852804032304306, 1.000000000000000000, 0.9807852804032304306, 1.000000000000000000, 0.9807852804032304306, 1.000000000000000000, 0.9807852804032304306, 1.000000000000000000, 0.9807852804032304306, 1.000000000000000000, 0.9807852804032304306, 1.000000000000000000, 0.9807852804032304306, 1.000000000000000000, 0.9807852804032304306, 1.000000000000000000, 0.9807852804032304306, 1.000000000000000000, 0.9807852804032304306, 1.000000000000000000, 0.9807852804032304306, 1.000000000000000000, 0.9807852804032304306, 1.000000000000000000, 0.9807852804032304306, 1.000000000000000000, 0.9807852804032304306, 1.000000000000000000, 0.9807852804032304306, 1.000000000000000000, 0.9807852804032304306, 1.000000000000000000, 0.9807852804032304306, 1.000000000000000000, 0.9807852804032304306, 1.000000000000000000, 0.9807852804032304306, 1.000000000000000000, 0.9807852804032304306, 1.000000000000000000, 0.9807852804032304306, 1.000000000000000000, 0.9807852804032304306, 1.000000000000000000, 0.9807852804032304306, 1.000000000000000000, 0.9807852804032304306, 1.000000000000000000, 0.9807852804032304306, 1.000000000000000000, 0.9807852804032304306, 1.000000000000000000, 0.9807852804032304306, 1.000000000000000000, 0.9807852804032304306, 1.000000000000000000, 0.9807852804032304306, 1.000000000000000000, 0.9807852804032304306, 1.000000000000000000, 0.9807852804032304306, 1.000000000000000000, 0.9807852804032304306, 1.000000000000000000, 0.9807852804032304306, 1.000000000000000000, 0.9807852804032304306, 1.000000000000000000, 0.9807852804032304306, 1.000000000000000000, 0.9807852804032304306, 1.000000000000000000, 0.9807852804032304306, 1.000000000000000000, 0.9807852804032304306, 1.000000000000000000, 0.9807852804032304306, 1.000000000000000000, 0.9807852804032304306, 1.000000000000000000, 0.9807852804032304306, 1.000000000000000000, 0.9807852804032304306, 1.000000000000000000, 0.9807852804032304306, 1.000000000000000000, 0.9807852804032304306, 1.000000000000000000, 0.9807852804032304306, 1.000000000000000000, 0.9807852804032304306, 1.000000000000000000, 0.9807852804032304306, 1.000000000000000000, 0.9807852804032304306, 1.000000000000000000, 0.9807852804032304306, 1.000000000000000000, 0.9807852804032304306, 1.000000000000000000, 0.9807852804032304306, 1.000000000000000000, 0.9807852804032304306, 1.000000000000000000, 0.9807852804032304306, 1.000000000000000000, 0.9807852804032304306, 1.000000000000000000, 0.9807852804032304306, 1.000000000000000000, 0.9807852804032304306, 1.000000000000000000, 0.9807852804032304306, 1.000000000000000000, 0.9807852804032304306, 1.000000000000000000, 0.9807852804032304306, 1.000000000000000000, 0.9807852804032304306, 1.000000000000000000, 0.9807852804032304306, 1.000000000000000000, 0.9807852804032304306, 1.000000000000000000, 0.9807852804032304306, 1.000000000000000000, 0.9807852804032304306, 1.000000000000000000, 0.9807852804032304306, 1.000000000000000000, 0.9807852804032304306, 1.000000000000000000, 0.9807852804032304306, 1.000000000000000000, 0.9807852804032304306, 1.000000000000000000, 0.9807852804032304306, 1.000000000000000000, 0.9807852804032304306, 1.000000000000000000, 0.9807852804032304306, 1.000000000000000000, 0.9807852804032304306, 1.000000000000000000, 0.9807852804032304306, 1.000000000000000000, 0.9807852804032304306, 1.000000000000000000, 0.9807852804032304306, 1.000000000000000000, 0.9807852804032304306, 1.000000000000000000, 0.9807852804032304306, 1.000000000000000000, 0.9807852804032304306, 1.000000000000000000, 0.9807852804032304306, 1.000000000000000000, 0.9807852804032304306, 1.000000000000000000, 0.9807852804032304306, 1.000000000000000000, 0.9807852804032304306, 1.000000000000000000, 0.9807852804032304306, 1.000000000000000000, 0.9807852804032304306, 1.000000000000000000, 0.9807852804032304306, 1.000000000000000000, 0.9807852804032304306, 1.000000000000000000, 0.9807852804032304306, 1.000000000000000000, 0.9807852804032304306, 1.000000000000000000, 0.9807852804032304306, 1.000000000000000000, 0.9807852804032304306, 1.000000000000000000, 0.9807852804032304306, 1.000000000000000000, 0.9807852804032304306, 1.000000000000000000, 0.9807852804032304306, 1.000000000000000000, 0.9807852804032304306, 1.000000000000000000, 0.9807852804032304306, 1.000000000000000000, 0.9807852804032304306, 1.000000000000000000, 0.9807852804032304306, 1.000000000000000000, 0.9807852804032304306, 1.000000000000000000, 0.9807852804032304306, 1.000000000000000000, 0.9807852804032304306, 1.000000000000000000, 0.9807852804032304306, 1.000000000000000000, 0.9807852804032304306, 1.000000000000000000, 0.9807852804032304306, 1.000000000000000000, 0.9807852804032304306, 1.000000000000000000, 0.9807852804032304306, 1.000000000000000000, 0.9807852804032304306, 1.000000000000000000, 0.9807852804032304306, 1.000000000000000000, 0.9807852804032304306, 1.000000000000000000, 0.9807852804032304306, 1.000000000000000000, 0.9807852804032304306, 1.000000000000000000, 0.9807852804032304306, 1.000000000000000000, 0.9807852804032304306, 1.000000000000000000, 0.9807852804032304306, 1.000000000000000000, 0.9807852804032304306, 1.000000000000000000, 0.9807852804032304306, 1.000000000000000000, 0.9807852804032304306, 1.000000000000000000, 0.9807852804032304306, 1.000000000000000000, 0.9807852804032304306, 1.000000000000000000, 0.9807852804032304306, 1.000000000000000000, 0.9807852804032304306, 1.000000000000000000, 0.9807852804032304306, 1.000000000000000000, 0.9807852804032304306, 1.000000000000000000, 0.9807852804032304306, 1.000000000000000000, 0.9807852804032304306, 1.000000000000000000, 0.9807852804032304306, 1.000000000000000000, 0.9807852804032304306, 1.000000000000000000, 0.9807852804032304306, 1.000000000000000000, 0.9807852804032304306, 1.000000000000000000, 0.9807852804032304306, 1.000000000000000000, 0.9807852804032304306, 1.000000000000000000, 0.9807852804032304306, 1.000000000000000000, 0.9807852804032304306, 1.000000000000000000, 0.9807852804032304306, 1.000000000000000000, 0.9807852804032304306, 1.000000000000000000, 0.9807852804032304306, 1.000000000000000000, 0.9807852804032304306, 1.000000000000000000, 0.9807852804032304306, 1.000000000000000000, 0.9807852804032304306, 1.000000000000000000, 0.9807852804032304306, 1.000000000000000000, 0.9807852804032304306, 1.000000000000000000, 0.9807852804032304306, 1.000000000000000000, 0.9807852804032304306, 1.000000000000000000, 0.9807852804032304306, 1.000000000000000000, 0.9807852804032304306, 1.000000000000000000, 0.9807852804032304306, 1.000000000000000000, 0.9807852804032304306, 1.000000000000000000, 0.9807852804032304306, 1.000000000000000000, 0.9807852804032304306, 1.000000000000000000, 0.9807852804032304306, 1.000000000000000000, 0.9807852804032304306, 1.000000000000000000, 0.9807852804032304306, 1.000000000000000000, 0.9807852804032304306, 1.000000000000000000, 0.9807852804032304306, 1.000000000000000000, 0.9807852804032304306, 1.000000000000000000, 0.9807852804032304306, 1.000000000000000000, 0.9807852804032304306, 1.000000000000000000, 0.9807852804032304306, 1.000000000000000000, 0.9807852804032304306, 1.000000000000000000, 0.9807852804032304306, 1.000000000000000000, 0.9807852804032304306, 1.000000000000000000, 0.9807852804032304306, 1.000000000000000000, 0.9807852804032304306, 1.000000000000000000, 0.9807852804032304306, 1.000000000000000000, 0.9807852804032304306, 1.000000000000000000, 0.9807852804032304306, 1.000000000000000000, 0.9807852804032304306, 1.000000000000000000, 0.9807852804032304306, 1.000000000000000000, 0.9807852804032304306, 1.000000000000000000, 0.9807852804032304306, 1.000000000000000000, 0.9807852804032304306, 1.000000000000000000, 0.9807852804032304306, 1.000000000000000000, 0.9807852804032304306, 1.000000000000000000, 0.9807852804032304306, 1.000000000000000000, 0.9807852804032304306, 1.000000000000000000, 0.9807852804032304306, 1.000000000000000000, 0.9807852804032304306, 1.000000000000000000, 0.9807852804032304306, 1.000000000000000000, 0.9807852804032304306, 1.000000000000000000, 0.9807852804032304306, 1.000000000000000000, 0.9807852804032304306, 1.000000000000000000, 0.9807852804032304306, 1.000000000000000000, 0.9807852804032304306, 1.000000000000000000, 0.9807852804032304306, 1.000000000000000000, 0.9807852804032304306, 1.000000000000000000, 0.9807852804032304306, 1.000000000000000000, 0.9807852804032304306, 1.000000000000000000, 0.9807852804032304306, 1.000000000000000000, 0.9807852804032304306, 1.000000000000000000, 0.9807852804032304306, 1.000000000000000000, 0.9807852804032304306, 1.000000000000000000, 0.9807852804032304306, 1.000000000000000000, 0.9807852804032304306, 1.000000000000000000, 0.9807852804032304306, 1.000000000000000000, 0.9807852804032304306, 1.000000000000000000, 0.9807852804032304306, 1.000000000000000000, 0.9807852804032304306, 1.000000000000000000, 0.9807852804032304306, 1.000000000000000000, 0.9807852804032304306, 1.000000000000000000, 0.9807852804032304306, 1.000000000000000000, 0.9807852804032304306, 1.000000000000000000, 0.9807852804032304306, 1.000000000000000000, 0.9807852804032304306, 1.000000000000000000, 0.9807852804032304306, 1.000000000000000000, 0.9807852804032304306, 1.000000000000000000, 0.9807852804032304306, 1.000000000000000000, 0.9807852804032304306, 1.000000000000000000, 0.9807852804032304306, 1.000000000000000000, 0.9807852804032304306, 1.000000000000000000, 0.9807852804032304306, 1.000000000000000000, 0.9807852804032304306, 1.000000000000000000, 0.9807852804032304306, 1.000000000000000000, 0.9807852804032304306, 1.000000000000000000, 0.9807852804032304306, 1.000000000000000000, 0.9807852804032304306, 1.000000000000000000, 0.9807852804032304306, 1.000000000000000000, 0.9807852804032304306, 1.000000000000000000, 0.9807852804032304306, 1.000000000000000000, 0.9807852804032304306, 1.000000000000000000, 0.9807852804032304306, 1.000000000000000000, 0.9807852804032304306, 1.000000000000000000, 0.9807852804032304306, 1.000000000000000000) ) ) 
 REPRESENTATION_ITEM ( '' )  SURFACE ( )  );
#27457=CARTESIAN_POINT ( 'NONE',  ( 8.843639120294245259, 48.46481371789856496, 3.474262827703527901 ) ) ;
#27459=CARTESIAN_POINT ( 'NONE',  ( -9.465287035748106703, 107.4023137178985650, 2.064181346179061460 ) ) ;
#27461=CARTESIAN_POINT ( 'NONE',  ( 12.50000000000000355, 29.48981371789854933, -0.1745138560722771515 ) ) ;
#27462=( GEOMETRIC_REPRESENTATION_CONTEXT ( 3 ) GLOBAL_UNCERTAINTY_ASSIGNED_CONTEXT ( ( #27144 ) ) GLOBAL_UNIT_ASSIGNED_CONTEXT ( ( #6853, #21275, #3811 ) ) REPRESENTATION_CONTEXT ( 'NONE', 'WORKASPACE' ) );
#27463=CARTESIAN_POINT ( 'NONE',  ( -10.69584247140444866, 85.44768628210144357, 6.932735513423972762 ) ) ;
#27473=CARTESIAN_POINT ( 'NONE',  ( 0.1745138560725194299, 88.61018628210146630, -9.500000000000005329 ) ) ;
#27474=CARTESIAN_POINT ( 'NONE',  ( 10.49813415415989581, 137.7726862821014606, 7.228626920339068285 ) ) ;
#27486=CARTESIAN_POINT ( 'NONE',  ( -9.500000000000005329, 6.489813717898557321, 0.1745138560723101806 ) ) ;
#27495=CARTESIAN_POINT ( 'NONE',  ( 12.50000000000000355, 29.48981371789854933, -0.1745138560722771515 ) ) ;
#27498=CARTESIAN_POINT ( 'NONE',  ( 8.927990412390371944, 122.9273137178985422, 13.04141134922778811 ) ) ;
#27505=CARTESIAN_POINT ( 'NONE',  ( 12.53471296425194836, 127.4226862821014663, -2.311890736173178418 ) ) ;
#27516=CARTESIAN_POINT ( 'NONE',  ( 8.927990412390657937, 126.2726862821014464, -13.04141134922759804 ) ) ;
#27518=CARTESIAN_POINT ( 'NONE',  ( -3.796722387233375073, 112.1851862821014691, 8.710071997420127943 ) ) ;
#27520=CARTESIAN_POINT ( 'NONE',  ( -8.715434833791929847, 13.86018628210145032, -8.962234695871762469 ) ) ;
#27524=CARTESIAN_POINT ( 'NONE',  ( 6.594114490232313663, 82.86018628210146630, 6.840914352312096547 ) ) ;
#27526=CARTESIAN_POINT ( 'NONE',  ( 1.715153634034445762, 128.6773137178985280, -9.534712964251895073 ) ) ;
#27532=CARTESIAN_POINT ( 'NONE',  ( -9.534712964251895073, 80.37731371789853085, -1.715153634034446428 ) ) ;
#27535=CARTESIAN_POINT ( 'NONE',  ( -0.1745138560722763466, 82.38981371789854791, -12.50000000000000355 ) ) ;
#27539=CARTESIAN_POINT ( 'NONE',  ( -10.69584247140429412, 44.15231371789854364, -6.932735513424201024 ) ) ;
#27543=CARTESIAN_POINT ( 'NONE',  ( -11.61527771782819940, 30.53518628210144570, 4.622313124798574258 ) ) ;
#27548=CARTESIAN_POINT ( 'NONE',  ( -12.50000000000000355, 70.88981371789856212, 0.1745138560722786503 ) ) ;
#27554=CARTESIAN_POINT ( 'NONE',  ( -2.908627838312453306, 32.07731371789855501, 15.53471296425188797 ) ) ;
#27558=CARTESIAN_POINT ( 'NONE',  ( -4.944772684328673229, 75.38518628210144357, 11.48171059495397728 ) ) ;
#27560=CARTESIAN_POINT ( 'NONE',  ( -10.83675517735155047, 32.26018628210145067, -11.08355503943142750 ) ) ;
#27563=CARTESIAN_POINT ( 'NONE',  ( -0.1745138560725817967, 38.01018628210144357, 15.50000000000000533 ) ) ;
#27571=CARTESIAN_POINT ( 'NONE',  ( -5.529263428287297444, 127.5273137178985792, -7.954856959092311719 ) ) ;
#27576=CARTESIAN_POINT ( 'NONE',  ( 4.622313124798831829, 138.1648137178985678, -11.61527771782809282 ) ) ;
#27582=CARTESIAN_POINT ( 'NONE',  ( 12.50000000000000355, 35.71018628210144641, 0.1745138560725507937 ) ) ;
#27590=CARTESIAN_POINT ( 'NONE',  ( 6.932735513423970097, 83.14768628210144641, 10.69584247140445044 ) ) ;
#27591=CARTESIAN_POINT ( 'NONE',  ( -0.1745138560722442889, 8.789813717898553591, -15.50000000000000533 ) ) ;
#27596=CARTESIAN_POINT ( 'NONE',  ( -10.49813415416004858, 125.2273137178985820, 7.228626920338839135 ) ) ;
#27603=CARTESIAN_POINT ( 'NONE',  ( -15.50000000000000533, 107.6898137178985735, 0.1745138560722471477 ) ) ;
#27607=CARTESIAN_POINT ( 'NONE',  ( -2.311890736173176641, 125.1226862821014549, -12.53471296425194836 ) ) ;
#27608=CARTESIAN_POINT ( 'NONE',  ( -2.908627838312119351, 79.12268628210145494, -15.53471296425195369 ) ) ;
#27611=CARTESIAN_POINT ( 'NONE',  ( -15.53471296425195369, 76.82268628210144357, 2.908627838312118019 ) ) ;
#27615=CARTESIAN_POINT ( 'NONE',  ( -8.843639120294326972, 48.93518628210144072, 3.474262827703335166 ) ) ;
#27620=CARTESIAN_POINT ( 'NONE',  ( -12.46528703574805697, 68.19768628210144357, -2.660918448318280838 ) ) ;
#27623=CARTESIAN_POINT ( 'NONE',  ( 3.474262827703335166, 37.43518628210144072, 8.843639120294326972 ) ) ;
#27633=CARTESIAN_POINT ( 'NONE',  ( 0.1745138560722779009, 86.98981371789855643, 12.50000000000000355 ) ) ;
#27634=CARTESIAN_POINT ( 'NONE',  ( -10.49813415415989404, 77.97268628210144925, -7.228626920339069173 ) ) ;
#27639=CARTESIAN_POINT ( 'NONE',  ( -13.23911966647199812, 53.35231371789856780, -8.632099005475788900 ) ) ;
#27647=CARTESIAN_POINT ( 'NONE',  ( -0.1745138560723084320, 63.98981371789855643, -9.500000000000005329 ) ) ;
#27649=CARTESIAN_POINT ( 'NONE',  ( 9.500000000000005329, 93.88981371789856212, -0.1745138560723090149 ) ) ;
#27651=CARTESIAN_POINT ( 'NONE',  ( 6.932735513424201024, 37.25231371789855217, -10.69584247140429412 ) ) ;
#27653=CARTESIAN_POINT ( 'NONE',  ( -10.69584247140444866, 76.24768628210144072, 6.932735513423972762 ) ) ;
#27660=CARTESIAN_POINT ( 'NONE',  ( -3.474262827703337830, 88.03518628210144925, -8.843639120294326972 ) ) ;
#27663=CARTESIAN_POINT ( 'NONE',  ( 8.715434833791931624, 138.0601862821014549, 8.962234695871760692 ) ) ;
#27664=CARTESIAN_POINT ( 'NONE',  ( -10.88186518451280627, 142.9999999999999716, 1.989529451084718126 ) ) ;
#27674=CARTESIAN_POINT ( 'NONE',  ( 2.660918448318002838, 132.7023137178985621, 12.46528703574811558 ) ) ;
#27679=CARTESIAN_POINT ( 'NONE',  ( 2.311890736173452421, 9.077313717898549683, -12.53471296425189152 ) ) ;
#27681=CARTESIAN_POINT ( 'NONE',  ( -15.53471296425188442, 117.1773137178985706, -2.908627838312459080 ) ) ;
#27688=CARTESIAN_POINT ( 'NONE',  ( -6.932735513423968321, 124.5476862821014663, -10.69584247140445221 ) ) ;
#27696=CARTESIAN_POINT ( 'NONE',  ( -8.715434833791929847, 133.4601862821014606, -8.962234695871762469 ) ) ;
#27700=CARTESIAN_POINT ( 'NONE',  ( 3.257655550457285720, 125.6976862821014578, -15.46528703574804986 ) ) ;
#27702=CARTESIAN_POINT ( 'NONE',  ( -1.715153634034234598, 115.9226862821014521, -9.534712964251941258 ) ) ;
#27704=CARTESIAN_POINT ( 'NONE',  ( 6.932735513423970097, 9.547686282101453870, 10.69584247140445044 ) ) ;
#27708=CARTESIAN_POINT ( 'NONE',  ( 1.715153634034233487, 83.72268628210143504, 9.534712964251941258 ) ) ;
#27710=CARTESIAN_POINT ( 'NONE',  ( 2.064181346179061460, 123.5023137178985451, 9.465287035748106703 ) ) ;
#27716=CARTESIAN_POINT ( 'NONE',  ( 5.233372021372610483, 55.65231371789855785, -8.152565276336593669 ) ) ;
#27721=CARTESIAN_POINT ( 'NONE',  ( 12.46528703574811558, 75.20231371789854791, -2.660918448318005947 ) ) ;
#27725=CARTESIAN_POINT ( 'NONE',  ( -8.962234695871565293, 26.03981371789855359, -8.715434833792128799 ) ) ;
#27729=CARTESIAN_POINT ( 'NONE',  ( 11.48171059495397728, 17.88518628210143646, 4.944772684328674117 ) ) ;
#27734=CARTESIAN_POINT ( 'NONE',  ( 10.49813415416005213, 65.42731371789855643, -7.228626920338837358 ) ) ;
#27741=CARTESIAN_POINT ( 'NONE',  ( -14.25334919248795096, 33.51481371789854791, 6.092822981423662299 ) ) ;
#27744=CARTESIAN_POINT ( 'NONE',  ( 10.49813415415989581, 64.17268628210143788, 7.228626920339068285 ) ) ;
#27745=CARTESIAN_POINT ( 'NONE',  ( 11.08355503943142750, 16.16018628210144570, -10.83675517735155225 ) ) ;
#27749=CARTESIAN_POINT ( 'NONE',  ( -13.23911966647218463, 21.04768628210144499, 8.632099005475506459 ) ) ;
#27754=CARTESIAN_POINT ( 'NONE',  ( 4.944772684328679446, 6.385186282101440014, -11.48171059495397373 ) ) ;
#27756=CARTESIAN_POINT ( 'NONE',  ( -8.843639120294245259, 117.4648137178985650, -3.474262827703533230 ) ) ;
#27761=CARTESIAN_POINT ( 'NONE',  ( 11.61527771782809637, 140.4648137178985792, 4.622313124798827388 ) ) ;
#27768=CARTESIAN_POINT ( 'NONE',  ( 2.660918448318279950, 33.69768628210144357, -12.46528703574805874 ) ) ;
#27776=CARTESIAN_POINT ( 'NONE',  ( 10.69584247140445221, 80.84768628210144925, -6.932735513423970097 ) ) ;
#27778=CARTESIAN_POINT ( 'NONE',  ( -3.257655550457281723, 139.4976862821014549, 15.46528703574804986 ) ) ;
#27786=CARTESIAN_POINT ( 'NONE',  ( 12.53471296425189330, 130.9773137178985678, 2.311890736173451977 ) ) ;
#27791=CARTESIAN_POINT ( 'NONE',  ( 14.38691631536194393, 94.46481371789855075, 5.770363421894124656 ) ) ;
#27795=CARTESIAN_POINT ( 'NONE',  ( -10.69584247140444866, 122.2476862821014549, 6.932735513423972762 ) ) ;
#27796=CARTESIAN_POINT ( 'NONE',  ( -11.08355503943142573, 66.76018628210144357, 10.83675517735155402 ) ) ;
#27799=CARTESIAN_POINT ( 'NONE',  ( 11.08355503943142750, 89.76018628210145778, -10.83675517735155225 ) ) ;
#27803=CARTESIAN_POINT ( 'NONE',  ( -6.594114490232312775, 41.46018628210145351, -6.840914352312096547 ) ) ;
#27807=CARTESIAN_POINT ( 'NONE',  ( -8.962234695871760692, 57.56018628210145494, 8.715434833791933400 ) ) ;
#27810=CARTESIAN_POINT ( 'NONE',  ( 5.529263428287477744, 25.07268628210145067, -7.954856959092191815 ) ) ;
#27819=CARTESIAN_POINT ( 'NONE',  ( -4.622313124798826500, 87.56481371789855928, 11.61527771782809637 ) ) ;
#27820=CARTESIAN_POINT ( 'NONE',  ( 4.622313124798573369, 92.63518628210145778, 11.61527771782819940 ) ) ;
#27824=CARTESIAN_POINT ( 'NONE',  ( 6.092822981423662299, 58.81481371789855217, 14.25334919248795096 ) ) ;
#27829=CARTESIAN_POINT ( 'NONE',  ( -3.474262827703527901, 41.56481371789855217, 8.843639120294245259 ) ) ;
#27831=CARTESIAN_POINT ( 'NONE',  ( -0.1745138560723084320, 100.7898137178985536, -9.500000000000005329 ) ) ;
#27833=CARTESIAN_POINT ( 'NONE',  ( 12.46528703574811558, 10.80231371789855466, -2.660918448318005503 ) ) ;
#27834=CARTESIAN_POINT ( 'NONE',  ( -12.50000000000000355, 58.71018628210145351, -0.1745138560725492671 ) ) ;
#27842=CARTESIAN_POINT ( 'NONE',  ( -8.843639120294326972, 94.93518628210146915, 3.474262827703335166 ) ) ;
#27844=CARTESIAN_POINT ( 'NONE',  ( -11.61527771782819940, 104.1351862821014578, 4.622313124798574258 ) ) ;
#27845=CARTESIAN_POINT ( 'NONE',  ( -6.415111792407825142, 142.9999999999984936, 10.48095429381284838 ) ) ;
#27855=CARTESIAN_POINT ( 'NONE',  ( -10.49813415416004858, 143.6273137178986019, 7.228626920338839135 ) ) ;
#27856=CARTESIAN_POINT ( 'NONE',  ( 6.932735513423970097, 138.3476862821014493, 10.69584247140445044 ) ) ;
#27863=CARTESIAN_POINT ( 'NONE',  ( 14.38691631536194393, 103.6648137178985678, 5.770363421894124656 ) ) ;
#27870=CARTESIAN_POINT ( 'NONE',  ( -11.61527771782819940, 122.5351862821014635, 4.622313124798574258 ) ) ;
#27877=CARTESIAN_POINT ( 'NONE',  ( 6.932735513423970097, 138.3476862821014493, 10.69584247140445044 ) ) ;
#27883=CARTESIAN_POINT ( 'NONE',  ( -15.46528703574804986, 123.3976862821014606, -3.257655550457287497 ) ) ;
#27885=CARTESIAN_POINT ( 'NONE',  ( -6.932735513423968321, 4.947686282101432909, -10.69584247140445221 ) ) ;
#27890=CARTESIAN_POINT ( 'NONE',  ( 0.1745138560725194299, 79.41018628210144925, -9.500000000000005329 ) ) ;
#27892=CARTESIAN_POINT ( 'NONE',  ( 3.474262827703532341, 128.9648137178985792, -8.843639120294245259 ) ) ;
#27898=CARTESIAN_POINT ( 'NONE',  ( 6.840914352311949109, 58.23981371789854222, 6.594114490232462877 ) ) ;
#27902=CARTESIAN_POINT ( 'NONE',  ( -4.944772684328424539, 54.21481371789854364, -11.48171059495408031 ) ) ;
#27906=CARTESIAN_POINT ( 'NONE',  ( 11.61527771782809637, 30.06481371789855572, 4.622313124798827388 ) ) ;
#27911=CARTESIAN_POINT ( 'NONE',  ( 12.50000000000000355, 8.110186282101444988, 0.1745138560725507937 ) ) ;
#27915=CARTESIAN_POINT ( 'NONE',  ( 4.622313124798831829, 64.56481371789855928, -11.61527771782809282 ) ) ;
#27920=CARTESIAN_POINT ( 'NONE',  ( 11.08355503943118769, 30.63981371789855146, 10.83675517735179028 ) ) ;
#27923=CARTESIAN_POINT ( 'NONE',  ( 7.228626920339068285, 25.07268628210144712, -10.49813415415989581 ) ) ;
#27925=CARTESIAN_POINT ( 'NONE',  ( -4.622313124798576922, 60.43518628210145494, -11.61527771782819762 ) ) ;
#27926=CARTESIAN_POINT ( 'NONE',  ( 13.23911966647218996, 16.44768628210144001, -8.632099005475504683 ) ) ;
#27930=CARTESIAN_POINT ( 'NONE',  ( 8.632099005475504683, 37.14768628210143220, 13.23911966647218996 ) ) ;
#27939=CARTESIAN_POINT ( 'NONE',  ( 3.796722387233182339, 104.8148137178985593, 8.710071997420207879 ) ) ;
#27944=CARTESIAN_POINT ( 'NONE',  ( -8.715434833792127023, 115.7398137178985706, 8.962234695871568846 ) ) ;
#27951=CARTESIAN_POINT ( 'NONE',  ( 11.48171059495397728, 27.08518628210144996, 4.944772684328674117 ) ) ;
#27959=CARTESIAN_POINT ( 'NONE',  ( 7.228626920339068285, 61.87268628210145494, -10.49813415415989581 ) ) ;
#27960=CARTESIAN_POINT ( 'NONE',  ( 15.50000000000000533, 136.9101862821014777, 0.1745138560725827404 ) ) ;
#27967=CARTESIAN_POINT ( 'NONE',  ( 6.932735513424201024, 120.0523137178985564, -10.69584247140429412 ) ) ;
#27972=CARTESIAN_POINT ( 'NONE',  ( -15.50000000000000533, 89.28981371789856780, 0.1745138560722471477 ) ) ;
#27977=CARTESIAN_POINT ( 'NONE',  ( 4.944772684328679446, 116.7851862821014635, -11.48171059495397373 ) ) ;
#27978=CARTESIAN_POINT ( 'NONE',  ( -10.83675517735155047, 69.06018628210144072, -11.08355503943142750 ) ) ;
#27981=CARTESIAN_POINT ( 'NONE',  ( -2.908627838312119351, 88.32268628210142936, -15.53471296425195369 ) ) ;
#27985=CARTESIAN_POINT ( 'NONE',  ( 1.715153634034233487, 28.52268628210144286, 9.534712964251941258 ) ) ;
#27988=CARTESIAN_POINT ( 'NONE',  ( 4.944772684328679446, 52.38518628210145067, -11.48171059495397373 ) ) ;
#27991=CARTESIAN_POINT ( 'NONE',  ( 5.529263428287477744, 34.27268628210144641, -7.954856959092191815 ) ) ;
#28001=CARTESIAN_POINT ( 'NONE',  ( -0.1745138560722763466, 82.38981371789854791, -12.50000000000000355 ) ) ;
#28002=CARTESIAN_POINT ( 'NONE',  ( 8.962234695871762469, 80.56018628210145494, -8.715434833791931624 ) ) ;
#28007=CARTESIAN_POINT ( 'NONE',  ( 8.632099005475788900, 55.65231371789855785, -13.23911966647199812 ) ) ;
#28012=CARTESIAN_POINT ( 'NONE',  ( 1.715153634034445762, 45.87731371789854506, -9.534712964251895073 ) ) ;
#28015=CARTESIAN_POINT ( 'NONE',  ( 3.796722387233182339, 95.61481371789857064, 8.710071997420207879 ) ) ;
#28017=CARTESIAN_POINT ( 'NONE',  ( 12.46528703574811558, 20.00231371789855217, -2.660918448318005503 ) ) ;
#28018=ADVANCED_FACE ( 'NONE', ( #1447 ), #27453, .T. ) ;
#28019=CARTESIAN_POINT ( 'NONE',  ( -8.715434833791929847, 59.86018628210145209, -8.962234695871762469 ) ) ;
#28028=CARTESIAN_POINT ( 'NONE',  ( 9.500000000000005329, 90.91018628210146346, 0.1745138560725188748 ) ) ;
#28032=CARTESIAN_POINT ( 'NONE',  ( 8.962234695871762469, 108.1601862821014635, -8.715434833791931624 ) ) ;
#28044=CARTESIAN_POINT ( 'NONE',  ( 6.594114490232462877, 9.939813717898537959, -6.840914352311949109 ) ) ;
#28051=CARTESIAN_POINT ( 'NONE',  ( 0.1745138560722461762, 114.5898137178985650, 15.50000000000000533 ) ) ;
#28057=CARTESIAN_POINT ( 'NONE',  ( 11.61527771782819940, 108.7351862821014663, -4.622313124798573369 ) ) ;
#28063=CARTESIAN_POINT ( 'NONE',  ( 10.69584247140445221, 126.8476862821014635, -6.932735513423970097 ) ) ;
#28069=CARTESIAN_POINT ( 'NONE',  ( 0.1745138560725837118, 116.2101862821014748, -15.50000000000000533 ) ) ;
#28071=CARTESIAN_POINT ( 'NONE',  ( -7.228626920339069173, 11.27268628210143042, 10.49813415415989581 ) ) ;
#28075=CARTESIAN_POINT ( 'NONE',  ( 3.796722387233379514, 79.98518628210145209, -8.710071997420127943 ) ) ;
#28077=CARTESIAN_POINT ( 'NONE',  ( -8.843639120294245259, 126.6648137178985820, -3.474262827703533230 ) ) ;
#28084=CARTESIAN_POINT ( 'NONE',  ( 9.465287035748106703, 56.80231371789854933, -2.064181346179063237 ) ) ;
#28088=CARTESIAN_POINT ( 'NONE',  ( 12.53471296425189330, 57.37731371789855928, 2.311890736173451533 ) ) ;
#28092=CARTESIAN_POINT ( 'NONE',  ( -0.1745138560722763466, 27.18981371789855217, -12.50000000000000355 ) ) ;
#28095=CARTESIAN_POINT ( 'NONE',  ( 12.46528703574805874, 8.397686282101442856, 2.660918448318279950 ) ) ;
#28102=CARTESIAN_POINT ( 'NONE',  ( 7.228626920338837358, 58.52731371789855785, 10.49813415416005036 ) ) ;
#28108=CARTESIAN_POINT ( 'NONE',  ( -3.257655550456946880, 36.10231371789854649, -15.46528703574811736 ) ) ;
#28110=CARTESIAN_POINT ( 'NONE',  ( -8.715434833791929847, 23.06018628210145138, -8.962234695871762469 ) ) ;
#28111=CARTESIAN_POINT ( 'NONE',  ( -7.228626920339069173, 75.67268628210146630, 10.49813415415989581 ) ) ;
#28112=CARTESIAN_POINT ( 'NONE',  ( 13.23911966647218996, 7.247686282101430066, -8.632099005475504683 ) ) ;
#28116=CARTESIAN_POINT ( 'NONE',  ( -11.08355503943142573, 29.96018628210143575, 10.83675517735155402 ) ) ;
#28125=CARTESIAN_POINT ( 'NONE',  ( -5.529263428287297444, 118.3273137178985763, -7.954856959092311719 ) ) ;
#28131=CARTESIAN_POINT ( 'NONE',  ( -10.49813415416004858, 116.0273137178985650, 7.228626920338840023 ) ) ;
#28144=CARTESIAN_POINT ( 'NONE',  ( 12.53471296425194836, 63.02268628210145351, -2.311890736173178418 ) ) ;
#28149=CARTESIAN_POINT ( 'NONE',  ( -4.622313124798826500, 124.3648137178985706, 11.61527771782809637 ) ) ;
#28155=CARTESIAN_POINT ( 'NONE',  ( -5.770363421894122880, 87.56481371789857349, 14.38691631536194393 ) ) ;
#28160=CARTESIAN_POINT ( 'NONE',  ( -12.53471296425194836, 113.6226862821014407, 2.311890736173176641 ) ) ;
#28161=CARTESIAN_POINT ( 'NONE',  ( 15.53471296425195369, 63.02268628210144641, -2.908627838312120684 ) ) ;
#28165=CARTESIAN_POINT ( 'NONE',  ( -5.770363421893818234, 88.03518628210144925, -14.38691631536207005 ) ) ;
#28169=CARTESIAN_POINT ( 'NONE',  ( 6.594114490232313663, 27.66018628210143859, 6.840914352312096547 ) ) ;
#28173=CARTESIAN_POINT ( 'NONE',  ( 4.944772684328679446, 61.58518628210145351, -11.48171059495397373 ) ) ;
#28176=CARTESIAN_POINT ( 'NONE',  ( 5.233372021372432847, 27.94768628210144001, 8.152565276336710909 ) ) ;
#28187=CARTESIAN_POINT ( 'NONE',  ( 10.69584247140445221, 80.84768628210144925, -6.932735513423970097 ) ) ;
#28193=CARTESIAN_POINT ( 'NONE',  ( 11.08355503943118769, 49.03981371789855359, 10.83675517735179028 ) ) ;
#28201=CARTESIAN_POINT ( 'NONE',  ( -9.500000000000005329, 43.28981371789856070, 0.1745138560723101806 ) ) ;
#28204=CARTESIAN_POINT ( 'NONE',  ( -8.843639120294245259, 89.86481371789855643, -3.474262827703533230 ) ) ;
#28206=CARTESIAN_POINT ( 'NONE',  ( -12.53471296425189152, 6.777313717898553413, -2.311890736173453753 ) ) ;
#28207=CARTESIAN_POINT ( 'NONE',  ( -11.48171059495397373, 68.48518628210145209, -4.944772684328680334 ) ) ;
#28215=CARTESIAN_POINT ( 'NONE',  ( 3.474262827703335166, 74.23518628210142367, 8.843639120294326972 ) ) ;
#28219=CARTESIAN_POINT ( 'NONE',  ( 7.228626920339068285, 117.0726862821014720, -10.49813415415989581 ) ) ;
#28231=CARTESIAN_POINT ( 'NONE',  ( -12.46528703574811558, 135.0023137178985735, 2.660918448318003726 ) ) ;
#28232=CARTESIAN_POINT ( 'NONE',  ( 2.660918448318279950, 134.8976862821014606, -12.46528703574805874 ) ) ;
#28237=CARTESIAN_POINT ( 'NONE',  ( 11.61527771782809637, 11.66481371789854293, 4.622313124798827388 ) ) ;
#28240=CARTESIAN_POINT ( 'NONE',  ( -6.092822981423666739, 118.6148137178985706, -14.25334919248795096 ) ) ;
#28245=CARTESIAN_POINT ( 'NONE',  ( -4.622313124798576922, 106.4351862821014549, -11.61527771782819762 ) ) ;
#28252=CARTESIAN_POINT ( 'NONE',  ( -12.50000000000000355, 123.1101862821014663, -0.1745138560725492671 ) ) ;
#28257=CARTESIAN_POINT ( 'NONE',  ( -6.092822981423970496, 112.1851862821014691, 14.25334919248782661 ) ) ;
#28259=CARTESIAN_POINT ( 'NONE',  ( -5.233372021372430183, 124.5476862821014663, -8.152565276336710909 ) ) ;
#28264=CARTESIAN_POINT ( 'NONE',  ( 8.710071997420127943, 73.08518628210143220, 3.796722387233375073 ) ) ;
#28270=CARTESIAN_POINT ( 'NONE',  ( 2.064181346179061460, 49.90231371789854364, 9.465287035748106703 ) ) ;
#28274=CARTESIAN_POINT ( 'NONE',  ( 6.932735513424201024, 64.85231371789855359, -10.69584247140429412 ) ) ;
#28277=CARTESIAN_POINT ( 'NONE',  ( -12.53471296425189152, 25.17731371789855288, -2.311890736173453753 ) ) ;
#28281=CARTESIAN_POINT ( 'NONE',  ( -2.660918448318275509, 10.69768628210143646, 12.46528703574805874 ) ) ;
#28292=CARTESIAN_POINT ( 'NONE',  ( 14.38691631536194393, 39.26481371789855501, 5.770363421894124656 ) ) ;
#28295=CARTESIAN_POINT ( 'NONE',  ( -12.53471296425194836, 12.42268628210144321, 2.311890736173176641 ) ) ;
#28296=CARTESIAN_POINT ( 'NONE',  ( -12.53471296425194836, 58.42268628210145209, 2.311890736173176641 ) ) ;
#28297=CARTESIAN_POINT ( 'NONE',  ( -15.50000000000000533, 12.71018628210143753, -0.1745138560725808530 ) ) ;
#28301=CARTESIAN_POINT ( 'NONE',  ( -15.53471296425195369, 21.62268628210143717, 2.908627838312118019 ) ) ;
#28308=CARTESIAN_POINT ( 'NONE',  ( -9.465287035748106703, 107.4023137178985650, 2.064181346179061460 ) ) ;
#28314=CARTESIAN_POINT ( 'NONE',  ( 11.48171059495408208, 111.7148137178985650, -4.944772684328420986 ) ) ;
#28327=CARTESIAN_POINT ( 'NONE',  ( -12.53471296425194836, 58.42268628210145209, 2.311890736173176641 ) ) ;
#28334=CARTESIAN_POINT ( 'NONE',  ( -2.660918448318004614, 118.9023137178985507, -12.46528703574811558 ) ) ;
#28341=CARTESIAN_POINT ( 'NONE',  ( -14.25334919248795096, 88.71481371789855075, 6.092822981423662299 ) ) ;
#28344=CARTESIAN_POINT ( 'NONE',  ( -10.49813415415989581, 114.7726862821014606, -7.228626920339068285 ) ) ;
#28345=CARTESIAN_POINT ( 'NONE',  ( -6.092822981423970496, 56.98518628210145209, 14.25334919248782661 ) ) ;
#28348=CARTESIAN_POINT ( 'NONE',  ( 8.632099005475504683, 92.34768628210142083, 13.23911966647218996 ) ) ;
#28350=CARTESIAN_POINT ( 'NONE',  ( 9.534712964251941258, 26.22268628210144925, -1.715153634034235708 ) ) ;
#28355=CARTESIAN_POINT ( 'NONE',  ( 10.69584247140445221, 62.44768628210145778, -6.932735513423970097 ) ) ;
#28358=CARTESIAN_POINT ( 'NONE',  ( -8.843639120294326972, 30.53518628210144570, 3.474262827703335166 ) ) ;
#28369=CARTESIAN_POINT ( 'NONE',  ( -12.50000000000000355, 95.51018628210144357, -0.1745138560725492671 ) ) ;
#28374=CARTESIAN_POINT ( 'NONE',  ( 13.23911966647199812, 30.35231371789855359, 8.632099005475788900 ) ) ;
#28381=CARTESIAN_POINT ( 'NONE',  ( 3.796722387233182339, 31.21481371789855430, 8.710071997420207879 ) ) ;
#28383=CARTESIAN_POINT ( 'NONE',  ( -2.064181346179062349, 91.30231371789854222, -9.465287035748106703 ) ) ;
#28385=CARTESIAN_POINT ( 'NONE',  ( -2.908627838312453306, 142.4773137178985678, 15.53471296425188797 ) ) ;
#28386=CARTESIAN_POINT ( 'NONE',  ( 0.1745138560725515708, 70.21018628210144641, -12.50000000000000355 ) ) ;
#28393=CARTESIAN_POINT ( 'NONE',  ( -3.796722387233375073, 75.38518628210142936, 8.710071997420127943 ) ) ;
#28395=CARTESIAN_POINT ( 'NONE',  ( 2.660918448318279950, 116.4976862821014549, -12.46528703574805697 ) ) ;
#28407=CARTESIAN_POINT ( 'NONE',  ( -12.50000000000000355, 126.0898137178985650, 0.1745138560722786503 ) ) ;
#28408=CARTESIAN_POINT ( 'NONE',  ( -2.311890736173176641, 134.3226862821014436, -12.53471296425194659 ) ) ;
#28409=ORIENTED_EDGE ( 'NONE', *, *, #11135, .F. ) ;
#28412=CARTESIAN_POINT ( 'NONE',  ( -8.715434833792127023, 14.53981371789855892, 8.962234695871568846 ) ) ;
#28413=CARTESIAN_POINT ( 'NONE',  ( -13.04141134922778456, 106.8273137178985479, 8.927990412390377273 ) ) ;
#28419=CARTESIAN_POINT ( 'NONE',  ( 6.932735513423970097, 119.9476862821014578, 10.69584247140445044 ) ) ;
#28425=CARTESIAN_POINT ( 'NONE',  ( 0.1745138560725515708, 116.2101862821014606, -12.50000000000000355 ) ) ;
#28432=CARTESIAN_POINT ( 'NONE',  ( 5.770363421893814682, 101.8351862821014606, 14.38691631536207183 ) ) ;
#28433=CARTESIAN_POINT ( 'NONE',  ( 12.50000000000000355, 17.31018628210144428, 0.1745138560725507937 ) ) ;
#28435=CARTESIAN_POINT ( 'NONE',  ( 3.796722387233379514, 125.9851862821014521, -8.710071997420127943 ) ) ;
#28441=CARTESIAN_POINT ( 'NONE',  ( -3.796722387233375073, 56.98518628210145209, 8.710071997420127943 ) ) ;
#28450=CARTESIAN_POINT ( 'NONE',  ( -9.465287035748106703, 33.80231371789854222, 2.064181346179061460 ) ) ;
#28455=CARTESIAN_POINT ( 'NONE',  ( 10.69584247140429589, 67.15231371789855075, 6.932735513424201024 ) ) ;
#28458=CARTESIAN_POINT ( 'NONE',  ( 4.622313124798831829, 36.96481371789854364, -11.61527771782809282 ) ) ;
#28474=CARTESIAN_POINT ( 'NONE',  ( 15.50000000000000533, 20.28981371789855004, -0.1745138560722452326 ) ) ;
#28476=CARTESIAN_POINT ( 'NONE',  ( -0.1745138560725182642, 139.2101862821014890, 9.500000000000005329 ) ) ;
#28477=CARTESIAN_POINT ( 'NONE',  ( 0.1745138560725515708, 42.61018628210144499, -12.50000000000000355 ) ) ;
#28482=CARTESIAN_POINT ( 'NONE',  ( 2.908627838312118019, 10.12268628210144428, 15.53471296425195369 ) ) ;
#28489=CARTESIAN_POINT ( 'NONE',  ( -3.796722387233185003, 118.6148137178985706, -8.710071997420207879 ) ) ;
#28496=CARTESIAN_POINT ( 'NONE',  ( 10.69584247140429589, 122.3523137178985678, 6.932735513424201024 ) ) ;
#28509=CARTESIAN_POINT ( 'NONE',  ( -12.46528703574805697, 49.79768628210145209, -2.660918448318280838 ) ) ;
#28514=CARTESIAN_POINT ( 'NONE',  ( -10.69584247140429412, 99.35231371789855359, -6.932735513424201024 ) ) ;
#28520=CARTESIAN_POINT ( 'NONE',  ( 10.83675517735179206, 92.73981371789854222, -11.08355503943118769 ) ) ;
#28524=CARTESIAN_POINT ( 'NONE',  ( 11.48171059495397728, 100.6851862821014691, 4.944772684328674117 ) ) ;
#28525=CARTESIAN_POINT ( 'NONE',  ( 14.25334919248782661, 73.08518628210143220, 6.092822981423971385 ) ) ;
#28528=CARTESIAN_POINT ( 'NONE',  ( -2.908627838312119351, 60.72268628210144925, -15.53471296425195369 ) ) ;
#28530=CARTESIAN_POINT ( 'NONE',  ( -0.1745138560725182642, 19.61018628210144144, 9.500000000000005329 ) ) ;
#28533=CARTESIAN_POINT ( 'NONE',  ( -2.311890736173176641, 51.52268628210145351, -12.53471296425194836 ) ) ;
#28536=CARTESIAN_POINT ( 'NONE',  ( -6.840914352312096547, 20.76018628210144001, 6.594114490232313663 ) ) ;
#28548=CARTESIAN_POINT ( 'NONE',  ( 12.50000000000000355, 63.31018628210144072, 0.1745138560725507937 ) ) ;
#28554=CARTESIAN_POINT ( 'NONE',  ( -8.927990412390371944, 35.52731371789855075, -13.04141134922778988 ) ) ;
#28560=CARTESIAN_POINT ( 'NONE',  ( 8.843639120294245259, 30.06481371789855572, 3.474262827703527901 ) ) ;
#28566=CARTESIAN_POINT ( 'NONE',  ( 11.48171059495408208, 19.71481371789854364, -4.944772684328420986 ) ) ;
#28569=CARTESIAN_POINT ( 'NONE',  ( 4.944772684328679446, 70.78518628210144925, -11.48171059495397373 ) ) ;
#28575=CARTESIAN_POINT ( 'NONE',  ( -8.843639120294326972, 85.73518628210145209, 3.474262827703335166 ) ) ;
#28578=CARTESIAN_POINT ( 'NONE',  ( -8.715434833791929847, 105.8601862821014521, -8.962234695871762469 ) ) ;
#28591=CARTESIAN_POINT ( 'NONE',  ( -4.622313124798826500, 115.1648137178985678, 11.61527771782809637 ) ) ;
#28592=CARTESIAN_POINT ( 'NONE',  ( -4.944772684328673229, 130.5851862821014606, 11.48171059495397728 ) ) ;
#28597=CARTESIAN_POINT ( 'NONE',  ( 15.50000000000000533, 93.88981371789856212, -0.1745138560722452326 ) ) ;
#28599=CARTESIAN_POINT ( 'NONE',  ( 8.715434833791931624, 92.06018628210145494, 8.962234695871760692 ) ) ;
#28603=CARTESIAN_POINT ( 'NONE',  ( -11.48171059495397373, 114.4851862821014521, -4.944772684328680334 ) ) ;
#28609=CARTESIAN_POINT ( 'NONE',  ( 8.715434833791931624, 119.6601862821014493, 8.962234695871760692 ) ) ;
#28614=CARTESIAN_POINT ( 'NONE',  ( -8.632099005475501130, 96.94768628210147199, -13.23911966647218996 ) ) ;
#28615=CARTESIAN_POINT ( 'NONE',  ( -12.53471296425194659, 21.62268628210144072, 2.311890736173176641 ) ) ;
#28619=CARTESIAN_POINT ( 'NONE',  ( -9.534712964251941258, 122.8226862821014294, 1.715153634034234154 ) ) ;
#28624=CARTESIAN_POINT ( 'NONE',  ( -2.064181346179269738, 65.89768628210143220, 9.465287035748067623 ) ) ;
#28633=CARTESIAN_POINT ( 'NONE',  ( -8.152565276336593669, 44.15231371789854364, -5.233372021372610483 ) ) ;
#28638=CARTESIAN_POINT ( 'NONE',  ( 7.228626920338837358, 58.52731371789855785, 10.49813415416005036 ) ) ;
#28641=CARTESIAN_POINT ( 'NONE',  ( -10.83675517735179028, 143.3398137178985507, 11.08355503943118947 ) ) ;
#28645=CARTESIAN_POINT ( 'NONE',  ( -8.715434833791929847, 4.660186282101435928, -8.962234695871762469 ) ) ;
#28657=CARTESIAN_POINT ( 'NONE',  ( 5.770363421894130873, 18.56481371789855928, -14.38691631536193860 ) ) ;
#28659=CARTESIAN_POINT ( 'NONE',  ( -11.48171059495397373, 13.28518628210142971, -4.944772684328680334 ) ) ;
#28660=CARTESIAN_POINT ( 'NONE',  ( -4.622313124798576922, 42.03518628210144215, -11.61527771782819762 ) ) ;
#28671=CARTESIAN_POINT ( 'NONE',  ( -5.529263428287297444, 99.92731371789854222, -7.954856959092311719 ) ) ;
#28677=EDGE_LOOP ( 'NONE', ( #34153, #26688 ) ) ;
#28678=CARTESIAN_POINT ( 'NONE',  ( 2.311890736173452421, 110.2773137178985650, -12.53471296425189152 ) ) ;
#28682=CARTESIAN_POINT ( 'NONE',  ( -11.48171059495408208, 79.51481371789856212, 4.944772684328421875 ) ) ;
#28694=CARTESIAN_POINT ( 'NONE',  ( -8.962234695871760692, 57.56018628210145494, 8.715434833791933400 ) ) ;
#28702=CARTESIAN_POINT ( 'NONE',  ( 12.46528703574811558, 102.8023137178985422, -2.660918448318005503 ) ) ;
#28708=CARTESIAN_POINT ( 'NONE',  ( 8.927990412390371944, 67.72731371789853938, 13.04141134922778811 ) ) ;
#28713=CARTESIAN_POINT ( 'NONE',  ( 7.228626920339068285, 98.67268628210145209, -10.49813415415989581 ) ) ;
#28714=CARTESIAN_POINT ( 'NONE',  ( -11.08355503943142573, 39.16018628210144215, 10.83675517735155402 ) ) ;
#28717=CARTESIAN_POINT ( 'NONE',  ( -3.257655550457281723, 75.09768628210143504, 15.46528703574804986 ) ) ;
#28721=CARTESIAN_POINT ( 'NONE',  ( -11.61527771782819940, 30.53518628210144570, 4.622313124798574258 ) ) ;
#28724=CARTESIAN_POINT ( 'NONE',  ( -3.474262827703337830, 14.43518628210144072, -8.843639120294326972 ) ) ;
#28734=CARTESIAN_POINT ( 'NONE',  ( 10.69584247140445221, 71.64768628210146062, -6.932735513423970097 ) ) ;
#28740=CARTESIAN_POINT ( 'NONE',  ( -13.04141134922778456, 33.22731371789855359, 8.927990412390377273 ) ) ;
#28746=CARTESIAN_POINT ( 'NONE',  ( -3.474262827703527901, 13.96481371789853831, 8.843639120294245259 ) ) ;
#28753=CARTESIAN_POINT ( 'NONE',  ( 10.83675517735179206, 129.5398137178985678, -11.08355503943118769 ) ) ;
#28755=CARTESIAN_POINT ( 'NONE',  ( 10.49813415415989581, 45.77268628210144641, 7.228626920339068285 ) ) ;
#28763=CARTESIAN_POINT ( 'NONE',  ( 1.715153634034233487, 74.52268628210144641, 9.534712964251941258 ) ) ;
#28765=CARTESIAN_POINT ( 'NONE',  ( -12.46528703574805697, 95.79768628210143788, -2.660918448318280838 ) ) ;
#28779=CARTESIAN_POINT ( 'NONE',  ( -10.69584247140429412, 126.9523137178985621, -6.932735513424201024 ) ) ;
#28780=CARTESIAN_POINT ( 'NONE',  ( 11.61527771782819940, 117.9351862821014549, -4.622313124798573369 ) ) ;
#28787=CARTESIAN_POINT ( 'NONE',  ( 11.08355503943118769, 95.03981371789855359, 10.83675517735179028 ) ) ;
#28790=CARTESIAN_POINT ( 'NONE',  ( -3.796722387233185003, 81.81481371789855928, -8.710071997420207879 ) ) ;
#28793=CARTESIAN_POINT ( 'NONE',  ( 11.48171059495408208, 74.91481371789855359, -4.944772684328420986 ) ) ;
#28795=CARTESIAN_POINT ( 'NONE',  ( -2.660918448318275509, 111.8976862821014606, 12.46528703574805874 ) ) ;
#28802=CARTESIAN_POINT ( 'NONE',  ( -15.46528703574804986, 95.79768628210145209, -3.257655550457287497 ) ) ;
#28803=CARTESIAN_POINT ( 'NONE',  ( -11.61527771782819940, 12.13518628210144534, 4.622313124798574258 ) ) ;
#28806=CARTESIAN_POINT ( 'NONE',  ( 9.465287035748067623, 127.9976862821014265, 2.064181346179272847 ) ) ;
#28810=CARTESIAN_POINT ( 'NONE',  ( 6.594114490232313663, 55.26018628210144357, 6.840914352312096547 ) ) ;
#28819=CARTESIAN_POINT ( 'NONE',  ( 6.594114490232462877, 37.53981371789855359, -6.840914352311949109 ) ) ;
#28824=CARTESIAN_POINT ( 'NONE',  ( 8.962234695871567070, 39.83981371789855075, 8.715434833792127023 ) ) ;
#28827=CARTESIAN_POINT ( 'NONE',  ( 8.962234695871567070, 12.23981371789853512, 8.715434833792127023 ) ) ;
#28844=CARTESIAN_POINT ( 'NONE',  ( -3.257655550456946880, 26.90231371789854364, -15.46528703574811736 ) ) ;
#28846=CARTESIAN_POINT ( 'NONE',  ( 2.660918448318279950, 6.097686282101443922, -12.46528703574805697 ) ) ;
#28848=CARTESIAN_POINT ( 'NONE',  ( -2.660918448318275509, 47.49768628210144783, 12.46528703574805874 ) ) ;
#28860=CARTESIAN_POINT ( 'NONE',  ( -5.529263428287297444, 90.72731371789855359, -7.954856959092311719 ) ) ;
#28868=CARTESIAN_POINT ( 'NONE',  ( -7.228626920338836470, 99.92731371789857064, -10.49813415416005213 ) ) ;
#28872=CARTESIAN_POINT ( 'NONE',  ( -10.69584247140429412, 62.55231371789856354, -6.932735513424201024 ) ) ;
#28882=CARTESIAN_POINT ( 'NONE',  ( 11.48171059495397728, 45.48518628210145209, 4.944772684328674117 ) ) ;
#28889=CARTESIAN_POINT ( 'NONE',  ( -8.962234695871565293, 99.63981371789856212, -8.715434833792128799 ) ) ;
#28894=CARTESIAN_POINT ( 'NONE',  ( -2.908627838312453306, 78.07731371789854791, 15.53471296425188797 ) ) ;
#28898=CARTESIAN_POINT ( 'NONE',  ( 0.1745138560725515708, 107.0101862821014578, -12.50000000000000355 ) ) ;
#28899=CARTESIAN_POINT ( 'NONE',  ( -15.53471296425195369, 40.02268628210144641, 2.908627838312118019 ) ) ;
#28902=CARTESIAN_POINT ( 'NONE',  ( 10.83675517735155225, 73.66018628210144925, 11.08355503943142573 ) ) ;
#28908=CARTESIAN_POINT ( 'NONE',  ( -8.962234695871760692, 39.16018628210144215, 8.715434833791933400 ) ) ;
#28911=CARTESIAN_POINT ( 'NONE',  ( 8.152565276336714462, 7.247686282101430066, -5.233372021372432847 ) ) ;
#28923=CARTESIAN_POINT ( 'NONE',  ( -12.46528703574805874, 58.99768628210144783, -2.660918448318280838 ) ) ;
#28930=CARTESIAN_POINT ( 'NONE',  ( -11.08355503943118592, 35.23981371789855643, -10.83675517735179383 ) ) ;
#28937=CARTESIAN_POINT ( 'NONE',  ( 5.529263428287300108, 21.72731371789853938, 7.954856959092309943 ) ) ;
#28942=CARTESIAN_POINT ( 'NONE',  ( 14.25334919248795451, 139.3148137178985451, -6.092822981423661410 ) ) ;
#28944=CARTESIAN_POINT ( 'NONE',  ( 12.53471296425194836, 53.82268628210144357, -2.311890736173178418 ) ) ;
#28952=CARTESIAN_POINT ( 'NONE',  ( 0.1745138560725194299, 70.21018628210144641, -9.500000000000005329 ) ) ;
#28954=CARTESIAN_POINT ( 'NONE',  ( -11.48171059495397373, 86.88518628210145778, -4.944772684328680334 ) ) ;
#28965=CARTESIAN_POINT ( 'NONE',  ( 4.944772684328420986, 123.2148137178985650, 11.48171059495408208 ) ) ;
#28966=CARTESIAN_POINT ( 'NONE',  ( -0.1745138560725500443, 130.0101862821014436, 12.50000000000000355 ) ) ;
#28971=CARTESIAN_POINT ( 'NONE',  ( -15.53471296425188442, 89.57731371789856212, -2.908627838312459080 ) ) ;
#28975=CARTESIAN_POINT ( 'NONE',  ( 3.796722387233182339, 68.01481371789854791, 8.710071997420207879 ) ) ;
#28979=CARTESIAN_POINT ( 'NONE',  ( 8.715434833792128799, 55.93981371789855217, -8.962234695871567070 ) ) ;
#28981=CARTESIAN_POINT ( 'NONE',  ( 0.1745138560725515708, 97.81018628210144072, -12.50000000000000355 ) ) ;
#28986=CARTESIAN_POINT ( 'NONE',  ( -6.092822981423970496, 93.78518628210144925, 14.25334919248782661 ) ) ;
#28987=CARTESIAN_POINT ( 'NONE',  ( 8.962234695871762469, 6.960186282101432198, -8.715434833791931624 ) ) ;
#28990=CARTESIAN_POINT ( 'NONE',  ( -6.840914352312096547, 131.1601862821014777, 6.594114490232313663 ) ) ;
#28995=CARTESIAN_POINT ( 'NONE',  ( -1.715153634034234598, 69.92268628210143788, -9.534712964251941258 ) ) ;
#29001=CARTESIAN_POINT ( 'NONE',  ( 9.465287035748106703, 47.60231371789853938, -2.064181346179063237 ) ) ;
#29006=CARTESIAN_POINT ( 'NONE',  ( 11.48171059495408208, 38.11481371789854222, -4.944772684328420986 ) ) ;
#29009=CARTESIAN_POINT ( 'NONE',  ( -12.53471296425189152, 6.777313717898553413, -2.311890736173453753 ) ) ;
#29025=CARTESIAN_POINT ( 'NONE',  ( 2.908627838312458636, 18.27731371789853299, -15.53471296425188442 ) ) ;
#29027=CARTESIAN_POINT ( 'NONE',  ( -10.49813415415989581, 13.57268628210145600, -7.228626920339068285 ) ) ;
#29028=CARTESIAN_POINT ( 'NONE',  ( -4.944772684328673229, 56.98518628210144499, 11.48171059495397728 ) ) ;
#29040=CARTESIAN_POINT ( 'NONE',  ( -3.796722387233185003, 91.01481371789856212, -8.710071997420207879 ) ) ;
#29047=CARTESIAN_POINT ( 'NONE',  ( -11.61527771782809282, 99.06481371789855928, -4.622313124798832717 ) ) ;
#29051=CARTESIAN_POINT ( 'NONE',  ( -8.962234695871565293, 72.03981371789855359, -8.715434833792128799 ) ) ;
#29060=CARTESIAN_POINT ( 'NONE',  ( 10.69584247140445221, 44.04768628210144499, -6.932735513423970097 ) ) ;
#29066=CARTESIAN_POINT ( 'NONE',  ( 8.962234695871567070, 95.03981371789856780, 8.715434833792127023 ) ) ;
#29072=CARTESIAN_POINT ( 'NONE',  ( -14.38691631536193860, 80.66481371789856780, -5.770363421894132649 ) ) ;
#29077=CARTESIAN_POINT ( 'NONE',  ( -10.69584247140444866, 103.8476862821014493, 6.932735513423972762 ) ) ;
#29078=CARTESIAN_POINT ( 'NONE',  ( 8.632099005475504683, 37.14768628210143220, 13.23911966647218996 ) ) ;
#29082=CARTESIAN_POINT ( 'NONE',  ( -15.53471296425195369, 67.62268628210145494, 2.908627838312118019 ) ) ;
#29088=CARTESIAN_POINT ( 'NONE',  ( -2.660918448318275509, 47.49768628210144783, 12.46528703574805874 ) ) ;
#29091=CARTESIAN_POINT ( 'NONE',  ( 6.840914352312096547, 16.16018628210144570, -6.594114490232313663 ) ) ;
#29102=CARTESIAN_POINT ( 'NONE',  ( -11.61527771782819940, 76.53518628210146346, 4.622313124798574258 ) ) ;
#29108=CARTESIAN_POINT ( 'NONE',  ( -14.25334919248795096, 42.71481371789855075, 6.092822981423662299 ) ) ;
#29115=CARTESIAN_POINT ( 'NONE',  ( 6.594114490232462877, 28.33981371789855430, -6.840914352311949109 ) ) ;
#29121=CARTESIAN_POINT ( 'NONE',  ( -11.08355503943118592, 127.2398137178985422, -10.83675517735179383 ) ) ;
#29124=CARTESIAN_POINT ( 'NONE',  ( -12.53471296425194836, 49.22268628210144215, 2.311890736173176641 ) ) ;
#29133=CARTESIAN_POINT ( 'NONE',  ( -5.529263428287477744, 57.27268628210143220, 7.954856959092191815 ) ) ;
#29136=CARTESIAN_POINT ( 'NONE',  ( -10.49813415415989581, 96.37268628210145494, -7.228626920339068285 ) ) ;
#29147=CARTESIAN_POINT ( 'NONE',  ( -11.61527771782809282, 126.6648137178985678, -4.622313124798832717 ) ) ;
#29148=CARTESIAN_POINT ( 'NONE',  ( -8.715434833791929847, 124.2601862821014578, -8.962234695871762469 ) ) ;
#29153=CARTESIAN_POINT ( 'NONE',  ( -2.908627838312453306, 87.27731371789855075, 15.53471296425188797 ) ) ;
#29158=CARTESIAN_POINT ( 'NONE',  ( -6.594114490232462877, 78.93981371789855928, 6.840914352311949109 ) ) ;
#29162=CARTESIAN_POINT ( 'NONE',  ( 6.932735513424201024, 55.65231371789855785, -10.69584247140429412 ) ) ;
#29165=CARTESIAN_POINT ( 'NONE',  ( 4.622313124798573369, 92.63518628210145778, 11.61527771782819940 ) ) ;
#29171=CARTESIAN_POINT ( 'NONE',  ( 15.50000000000000533, 100.1101862821014521, 0.1745138560725827404 ) ) ;
#29176=CARTESIAN_POINT ( 'NONE',  ( 9.534712964251941258, 118.2226862821014493, -1.715153634034235708 ) ) ;
#29178=CARTESIAN_POINT ( 'NONE',  ( 3.257655550457285720, 15.29768628210142722, -15.46528703574804986 ) ) ;
#29183=CARTESIAN_POINT ( 'NONE',  ( 2.064181346179272847, 70.49768628210145494, -9.465287035748065847 ) ) ;
#29190=CARTESIAN_POINT ( 'NONE',  ( 6.594114490232462877, 46.73981371789855643, -6.840914352311949109 ) ) ;
#29195=CARTESIAN_POINT ( 'NONE',  ( -10.69584247140429412, 34.95231371789854791, -6.932735513424201024 ) ) ;
#29198=CARTESIAN_POINT ( 'NONE',  ( 0.1745138560722779009, 13.38981371789854613, 12.50000000000000355 ) ) ;
#29208=FILL_AREA_STYLE ('',( #14823 ) ) ;
#29215=CARTESIAN_POINT ( 'NONE',  ( 13.04141134922778988, 19.42731371789854933, -8.927990412390371944 ) ) ;
#29218=CARTESIAN_POINT ( 'NONE',  ( 9.534712964251941258, 136.6226862821014549, -1.715153634034235708 ) ) ;
#29219=CARTESIAN_POINT ( 'NONE',  ( 10.49813415415989581, 45.77268628210144641, 7.228626920339068285 ) ) ;
#29225=CARTESIAN_POINT ( 'NONE',  ( 3.474262827703335166, 28.23518628210144854, 8.843639120294326972 ) ) ;
#29233=CARTESIAN_POINT ( 'NONE',  ( -6.594114490232462877, 88.13981371789856212, 6.840914352311949109 ) ) ;
#29238=CARTESIAN_POINT ( 'NONE',  ( 12.46528703574811558, 93.60231371789856780, -2.660918448318005947 ) ) ;
#29242=CARTESIAN_POINT ( 'NONE',  ( 12.53471296425189330, 66.57731371789856212, 2.311890736173451977 ) ) ;
#29250=CARTESIAN_POINT ( 'NONE',  ( -2.660918448318275509, 47.49768628210144783, 12.46528703574805874 ) ) ;
#29255=CARTESIAN_POINT ( 'NONE',  ( 10.49813415416005213, 102.2273137178985536, -7.228626920338837358 ) ) ;
#29262=CARTESIAN_POINT ( 'NONE',  ( -6.092822981423666739, 72.61481371789855643, -14.25334919248795096 ) ) ;
#29266=CARTESIAN_POINT ( 'NONE',  ( 11.61527771782819940, 99.53518628210144925, -4.622313124798573369 ) ) ;
#29267=CARTESIAN_POINT ( 'NONE',  ( 8.927990412390657937, 43.47268628210144215, -13.04141134922759804 ) ) ;
#29269=FACE_OUTER_BOUND ( 'NONE', #14816, .T. ) ;
#29271=CARTESIAN_POINT ( 'NONE',  ( -8.927990412390661490, 66.47268628210146346, 13.04141134922759804 ) ) ;
#29277=CARTESIAN_POINT ( 'NONE',  ( 12.53471296425194836, 35.42268628210144499, -2.311890736173178418 ) ) ;
#29280=CARTESIAN_POINT ( 'NONE',  ( 9.465287035748067623, 8.397686282101439303, 2.064181346179272847 ) ) ;
#29283=ORIENTED_EDGE ( 'NONE', *, *, #25320, .T. ) ;
#29292=CARTESIAN_POINT ( 'NONE',  ( 8.715434833791931624, 73.66018628210144925, 8.962234695871760692 ) ) ;
#29299=CARTESIAN_POINT ( 'NONE',  ( 12.53471296425194836, 99.82268628210144357, -2.311890736173178418 ) ) ;
#29300=CARTESIAN_POINT ( 'NONE',  ( 15.50000000000000533, 29.48981371789855288, -0.1745138560722452326 ) ) ;
#29306=CARTESIAN_POINT ( 'NONE',  ( -8.710071997420207879, 15.11481371789854933, 3.796722387233182339 ) ) ;
#29313=CARTESIAN_POINT ( 'NONE',  ( 10.83675517735179206, 138.7398137178985564, -11.08355503943118769 ) ) ;
#29317=CARTESIAN_POINT ( 'NONE',  ( 2.311890736173175753, 46.92268628210145209, 12.53471296425194836 ) ) ;
#29325=CARTESIAN_POINT ( 'NONE',  ( 8.152565276336714462, 53.24768628210144783, -5.233372021372432847 ) ) ;
#29329=CARTESIAN_POINT ( 'NONE',  ( -12.50000000000000355, 95.51018628210144357, -0.1745138560725492671 ) ) ;
#29341=CARTESIAN_POINT ( 'NONE',  ( 10.49813415416005213, 111.4273137178985564, -7.228626920338837358 ) ) ;
#29342=CARTESIAN_POINT ( 'NONE',  ( -8.715434833791929847, 115.0601862821014549, -8.962234695871762469 ) ) ;
#29348=CARTESIAN_POINT ( 'NONE',  ( -15.53471296425188442, 98.77731371789855075, -2.908627838312459080 ) ) ;
#29351=CARTESIAN_POINT ( 'NONE',  ( -1.715153634034234598, 106.7226862821014635, -9.534712964251941258 ) ) ;
#29353=CARTESIAN_POINT ( 'NONE',  ( 9.534712964251900402, 84.97731371789856780, 1.715153634034445540 ) ) ;
#29356=CARTESIAN_POINT ( 'NONE',  ( -0.1745138560722763466, 54.78981371789855359, -12.50000000000000355 ) ) ;
#29359=CARTESIAN_POINT ( 'NONE',  ( -10.69584247140444866, 103.8476862821014493, 6.932735513423972762 ) ) ;
#29364=CARTESIAN_POINT ( 'NONE',  ( -13.04141134922759804, 77.97268628210142083, -8.927990412390657937 ) ) ;
#29368=CARTESIAN_POINT ( 'NONE',  ( 2.064181346179272847, 116.4976862821014549, -9.465287035748065847 ) ) ;
#29371=CARTESIAN_POINT ( 'NONE',  ( -6.092822981423970496, 20.18518628210144783, 14.25334919248782661 ) ) ;
#29384=CARTESIAN_POINT ( 'NONE',  ( 9.465287035748106703, 29.20231371789855501, -2.064181346179063237 ) ) ;
#29388=CARTESIAN_POINT ( 'NONE',  ( -2.311890736173447980, 50.47731371789855359, 12.53471296425189330 ) ) ;
#29391=CARTESIAN_POINT ( 'NONE',  ( -2.660918448318004614, 8.502313717898557499, -12.46528703574811558 ) ) ;
#29412=CARTESIAN_POINT ( 'NONE',  ( -15.50000000000000533, 6.489813717898557321, 0.1745138560722471477 ) ) ;
#29414=CARTESIAN_POINT ( 'NONE',  ( 9.465287035748067623, 127.9976862821014265, 2.064181346179272847 ) ) ;
#29415=CARTESIAN_POINT ( 'NONE',  ( -4.944772684328673229, 38.58518628210144641, 11.48171059495397728 ) ) ;
#29419=CARTESIAN_POINT ( 'NONE',  ( -11.08355503943142573, 131.1601862821014777, 10.83675517735155402 ) ) ;
#29421=CARTESIAN_POINT ( 'NONE',  ( 3.796722387233379514, 6.385186282101440902, -8.710071997420127943 ) ) ;
#29428=CARTESIAN_POINT ( 'NONE',  ( 7.954856959092311719, 93.02731371789853654, -5.529263428287300108 ) ) ;
#29433=CARTESIAN_POINT ( 'NONE',  ( 4.622313124798831829, 92.16481371789855359, -11.61527771782809282 ) ) ;
#29437=CARTESIAN_POINT ( 'NONE',  ( -4.622313124798826500, 59.96481371789855075, 11.61527771782809637 ) ) ;
#29445=CARTESIAN_POINT ( 'NONE',  ( 12.50000000000000355, 35.71018628210144641, 0.1745138560725507937 ) ) ;
#29450=CARTESIAN_POINT ( 'NONE',  ( 6.932735513424201024, 83.25231371789857349, -10.69584247140429412 ) ) ;
#29455=CARTESIAN_POINT ( 'NONE',  ( 0.1745138560722461762, 68.58981371789855075, 15.50000000000000533 ) ) ;
#29459=CARTESIAN_POINT ( 'NONE',  ( 4.944772684328679446, 79.98518628210145209, -11.48171059495397373 ) ) ;
#29460=CARTESIAN_POINT ( 'NONE',  ( 15.46528703574804986, 45.19768628210142225, 3.257655550457285720 ) ) ;
#29463=CARTESIAN_POINT ( 'NONE',  ( -8.632099005475501130, 50.94768628210145067, -13.23911966647218996 ) ) ;
#29470=CARTESIAN_POINT ( 'NONE',  ( -8.715434833791929847, 32.26018628210145067, -8.962234695871762469 ) ) ;
#29472=CARTESIAN_POINT ( 'NONE',  ( -5.233372021372612259, 143.0523137178985280, 8.152565276336593669 ) ) ;
#29482=CARTESIAN_POINT ( 'NONE',  ( -4.622313124798576922, 42.03518628210144215, -11.61527771782819762 ) ) ;
#29491=CARTESIAN_POINT ( 'NONE',  ( -4.944772684328673229, 102.9851862821014663, 11.48171059495397728 ) ) ;
#29492=CARTESIAN_POINT ( 'NONE',  ( 5.770363421894130873, 18.56481371789855928, -14.38691631536193860 ) ) ;
#29498=CARTESIAN_POINT ( 'NONE',  ( -5.529263428287297444, 26.32731371789854791, -7.954856959092311719 ) ) ;
#29504=CARTESIAN_POINT ( 'NONE',  ( 15.53471296425188797, 140.1773137178985564, 2.908627838312457747 ) ) ;
#29507=CARTESIAN_POINT ( 'NONE',  ( -12.46528703574805697, 49.79768628210145209, -2.660918448318280838 ) ) ;
#29515=CARTESIAN_POINT ( 'NONE',  ( -1.715153634034234598, 51.52268628210144641, -9.534712964251941258 ) ) ;
#29519=CARTESIAN_POINT ( 'NONE',  ( -8.715434833791929847, 87.46018628210144641, -8.962234695871762469 ) ) ;
#29532=CARTESIAN_POINT ( 'NONE',  ( 12.46528703574811558, 102.8023137178985422, -2.660918448318005503 ) ) ;
#29533=CARTESIAN_POINT ( 'NONE',  ( -12.50000000000000355, 113.9101862821014493, -0.1745138560725492671 ) ) ;
#29539=CARTESIAN_POINT ( 'NONE',  ( 0.1745138560722461762, 77.78981371789853938, 15.50000000000000533 ) ) ;
#29542=CARTESIAN_POINT ( 'NONE',  ( 6.594114490232313663, 92.06018628210145494, 6.840914352312096547 ) ) ;
#29545=CARTESIAN_POINT ( 'NONE',  ( 3.474262827703532341, 73.76481371789856212, -8.843639120294245259 ) ) ;
#29549=CARTESIAN_POINT ( 'NONE',  ( 12.53471296425189330, 57.37731371789855928, 2.311890736173451977 ) ) ;
#29551=CARTESIAN_POINT ( 'NONE',  ( 11.48171059495397728, 100.6851862821014691, 4.944772684328674117 ) ) ;
#29556=CARTESIAN_POINT ( 'NONE',  ( 10.83675517735155225, 92.06018628210145494, 11.08355503943142573 ) ) ;
#29558=CARTESIAN_POINT ( 'NONE',  ( 0.1745138560725515708, 5.810186282101447830, -12.50000000000000355 ) ) ;
#29562=CARTESIAN_POINT ( 'NONE',  ( 6.594114490232313663, 110.4601862821014606, 6.840914352312096547 ) ) ;
#29564=CARTESIAN_POINT ( 'NONE',  ( 6.092822981423978490, 6.385186282101440902, -14.25334919248782306 ) ) ;
#29575=CARTESIAN_POINT ( 'NONE',  ( -1.715153634034442431, 22.87731371789854151, 9.534712964251900402 ) ) ;
#29580=CARTESIAN_POINT ( 'NONE',  ( -6.932735513424201912, 32.65231371789855075, 10.69584247140429412 ) ) ;
#29582=CARTESIAN_POINT ( 'NONE',  ( 2.908627838312458636, 137.8773137178985735, -15.53471296425188442 ) ) ;
#29599=CARTESIAN_POINT ( 'NONE',  ( -0.1745138560722442889, 8.789813717898553591, -15.50000000000000533 ) ) ;
#29601=CARTESIAN_POINT ( 'NONE',  ( 8.710071997420127943, 128.2851862821014493, 3.796722387233375073 ) ) ;
#29604=CARTESIAN_POINT ( 'NONE',  ( -2.660918448318275509, 29.09768628210144925, 12.46528703574805874 ) ) ;
#29609=CARTESIAN_POINT ( 'NONE',  ( 8.927990412390657937, 126.2726862821014464, -13.04141134922759804 ) ) ;
#29611=CARTESIAN_POINT ( 'NONE',  ( -6.594114490232462877, 143.3398137178985507, 6.840914352311949109 ) ) ;
#29617=CARTESIAN_POINT ( 'NONE',  ( 2.064181346179061460, 77.50231371789855928, 9.465287035748106703 ) ) ;
#29621=CARTESIAN_POINT ( 'NONE',  ( 10.69584247140429589, 103.9523137178985621, 6.932735513424201024 ) ) ;
#29625=CARTESIAN_POINT ( 'NONE',  ( -10.69584247140429412, 53.35231371789855359, -6.932735513424201024 ) ) ;
#29632=CARTESIAN_POINT ( 'NONE',  ( -4.622313124798576922, 32.83518628210143930, -11.61527771782819762 ) ) ;
#29638=CARTESIAN_POINT ( 'NONE',  ( -4.622313124798826500, 87.56481371789855928, 11.61527771782809637 ) ) ;
#29643=CARTESIAN_POINT ( 'NONE',  ( 2.908627838312458636, 55.07731371789854080, -15.53471296425188442 ) ) ;
#29647=CARTESIAN_POINT ( 'NONE',  ( -2.660918448318275509, 93.49768628210145494, 12.46528703574805874 ) ) ;
#29649=CARTESIAN_POINT ( 'NONE',  ( 5.770363421893814682, 28.23518628210144854, 14.38691631536207183 ) ) ;
#29653=CARTESIAN_POINT ( 'NONE',  ( 15.46528703574804986, 45.19768628210142225, 3.257655550457285720 ) ) ;
#29658=CARTESIAN_POINT ( 'NONE',  ( 8.715434833791931624, 18.46018628210144286, 8.962234695871760692 ) ) ;
#29660=CARTESIAN_POINT ( 'NONE',  ( 3.796722387233182339, 123.2148137178985792, 8.710071997420207879 ) ) ;
#29671=CARTESIAN_POINT ( 'NONE',  ( 11.48171059495397728, 54.68518628210144783, 4.944772684328674117 ) ) ;
#29679=CARTESIAN_POINT ( 'NONE',  ( 2.660918448318279950, 88.89768628210146062, -12.46528703574805697 ) ) ;
#29680=CARTESIAN_POINT ( 'NONE',  ( 6.092822981423662299, 12.81481371789855217, 14.25334919248795096 ) ) ;
#29686=CARTESIAN_POINT ( 'NONE',  ( 4.944772684328420986, 132.4148137178985678, 11.48171059495408208 ) ) ;
#29692=CARTESIAN_POINT ( 'NONE',  ( 11.08355503943118769, 113.4398137178985593, 10.83675517735179028 ) ) ;
#29695=CARTESIAN_POINT ( 'NONE',  ( -12.50000000000000355, 31.11018628210143788, -0.1745138560725492671 ) ) ;
#29699=CARTESIAN_POINT ( 'NONE',  ( 10.83675517735155225, 101.2601862821014436, 11.08355503943142573 ) ) ;
#29702=CARTESIAN_POINT ( 'NONE',  ( 5.529263428287477744, 52.67268628210144499, -7.954856959092191815 ) ) ;
#29705=CARTESIAN_POINT ( 'NONE',  ( -12.50000000000000355, 77.11018628210145209, -0.1745138560725492671 ) ) ;
#29718=CARTESIAN_POINT ( 'NONE',  ( 10.49813415416005213, 102.2273137178985536, -7.228626920338837358 ) ) ;
#29719=CARTESIAN_POINT ( 'NONE',  ( -2.660918448318275509, 111.8976862821014606, 12.46528703574805874 ) ) ;
#29724=CARTESIAN_POINT ( 'NONE',  ( 15.53471296425188797, 75.77731371789855075, 2.908627838312457747 ) ) ;
#29728=CARTESIAN_POINT ( 'NONE',  ( 9.500000000000005329, 90.91018628210146346, 0.1745138560725188748 ) ) ;
#29730=CARTESIAN_POINT ( 'NONE',  ( 9.465287035748106703, 56.80231371789854933, -2.064181346179063237 ) ) ;
#29732=CARTESIAN_POINT ( 'NONE',  ( 7.954856959092311719, 120.6273137178985451, -5.529263428287300108 ) ) ;
#29734=CARTESIAN_POINT ( 'NONE',  ( -10.69584247140429412, 44.15231371789854364, -6.932735513424201024 ) ) ;
#29736=CARTESIAN_POINT ( 'NONE',  ( -6.932735513423968321, 106.1476862821014606, -10.69584247140445221 ) ) ;
#29742=CARTESIAN_POINT ( 'NONE',  ( -14.38691631536207183, 85.73518628210145209, 5.770363421893814682 ) ) ;
#29747=CARTESIAN_POINT ( 'NONE',  ( -0.1745138560725182642, 111.6101862821014521, 9.500000000000005329 ) ) ;
#29750=CARTESIAN_POINT ( 'NONE',  ( -15.46528703574804986, 3.797686282101448096, -3.257655550457287497 ) ) ;
#29761=CARTESIAN_POINT ( 'NONE',  ( 8.710071997420211432, 19.71481371789854720, -3.796722387233181895 ) ) ;
#29766=CARTESIAN_POINT ( 'NONE',  ( 10.69584247140429589, 21.15231371789855075, 6.932735513424201024 ) ) ;
#29768=CARTESIAN_POINT ( 'NONE',  ( -14.25334919248795096, 134.7148137178985507, 6.092822981423662299 ) ) ;
#29777=CARTESIAN_POINT ( 'NONE',  ( -12.50000000000000355, 123.1101862821014663, -0.1745138560725492671 ) ) ;
#29788=CARTESIAN_POINT ( 'NONE',  ( -6.092822981423666739, 8.214813717898532985, -14.25334919248795096 ) ) ;
#29791=CARTESIAN_POINT ( 'NONE',  ( -6.594114490232312775, 124.2601862821014578, -6.840914352312096547 ) ) ;
#29793=CARTESIAN_POINT ( 'NONE',  ( -12.46528703574805697, 22.19768628210145067, -2.660918448318280838 ) ) ;
#29797=CARTESIAN_POINT ( 'NONE',  ( -5.770363421893818234, 124.8351862821014748, -14.38691631536207005 ) ) ;
#29799=CARTESIAN_POINT ( 'NONE',  ( -3.474262827703337830, 5.235186282101429001, -8.843639120294326972 ) ) ;
#29805=CARTESIAN_POINT ( 'NONE',  ( -9.534712964251895073, 71.17731371789855643, -1.715153634034446428 ) ) ;
#29809=CARTESIAN_POINT ( 'NONE',  ( 12.53471296425189330, 84.97731371789855359, 2.311890736173451533 ) ) ;
#29813=CARTESIAN_POINT ( 'NONE',  ( 11.48171059495408208, 56.51481371789855501, -4.944772684328420986 ) ) ;
#29818=CARTESIAN_POINT ( 'NONE',  ( -11.48171059495397373, 13.28518628210142971, -4.944772684328680334 ) ) ;
#29825=CARTESIAN_POINT ( 'NONE',  ( 11.61527771782809637, 94.46481371789855075, 4.622313124798827388 ) ) ;
#29830=CARTESIAN_POINT ( 'NONE',  ( 15.53471296425188797, 66.57731371789853370, 2.908627838312457747 ) ) ;
#29834=CARTESIAN_POINT ( 'NONE',  ( -2.311890736173176641, 88.32268628210144357, -12.53471296425194836 ) ) ;
#29835=CARTESIAN_POINT ( 'NONE',  ( -13.04141134922759804, 22.77268628210143220, -8.927990412390657937 ) ) ;
#29838=CARTESIAN_POINT ( 'NONE',  ( -13.04141134922759804, 50.37268628210144783, -8.927990412390657937 ) ) ;
#29844=CARTESIAN_POINT ( 'NONE',  ( -11.61527771782819940, 12.13518628210144534, 4.622313124798574258 ) ) ;
#29846=CARTESIAN_POINT ( 'NONE',  ( -1.715153634034442431, 124.0773137178985621, 9.534712964251900402 ) ) ;
#29848=ORIENTED_EDGE ( 'NONE', *, *, #20597, .T. ) ;
#29852=CARTESIAN_POINT ( 'NONE',  ( -6.932735513424201912, 133.8523137178985678, 10.69584247140429412 ) ) ;
#29859=CARTESIAN_POINT ( 'NONE',  ( -8.962234695871760692, 57.56018628210145494, 8.715434833791933400 ) ) ;
#29868=CARTESIAN_POINT ( 'NONE',  ( -7.228626920339069173, 94.07268628210145778, 10.49813415415989581 ) ) ;
#29869=CARTESIAN_POINT ( 'NONE',  ( 11.08355503943118769, 21.43981371789854506, 10.83675517735179028 ) ) ;
#29876=CARTESIAN_POINT ( 'NONE',  ( -0.1745138560723084320, 8.789813717898553591, -9.500000000000005329 ) ) ;
#29884=CARTESIAN_POINT ( 'NONE',  ( 15.53471296425188797, 112.5773137178985479, 2.908627838312457747 ) ) ;
#29887=CARTESIAN_POINT ( 'NONE',  ( 12.50000000000000355, 35.71018628210144641, 0.1745138560725507937 ) ) ;
#29892=CARTESIAN_POINT ( 'NONE',  ( 2.908627838312118019, 111.3226862821014578, 15.53471296425195369 ) ) ;
#29895=CARTESIAN_POINT ( 'NONE',  ( -2.064181346179269738, 56.69768628210144357, 9.465287035748067623 ) ) ;
#29900=CARTESIAN_POINT ( 'NONE',  ( 2.311890736173175753, 74.52268628210146062, 12.53471296425194836 ) ) ;
#29903=CARTESIAN_POINT ( 'NONE',  ( -2.064181346179269738, 47.49768628210145494, 9.465287035748067623 ) ) ;
#29912=CARTESIAN_POINT ( 'NONE',  ( -12.50000000000000355, 98.48981371789855643, 0.1745138560722786503 ) ) ;
#29913=CARTESIAN_POINT ( 'NONE',  ( 8.715434833791931624, 110.4601862821014606, 8.962234695871760692 ) ) ;
#29917=CARTESIAN_POINT ( 'NONE',  ( -10.83675517735179028, 78.93981371789855928, 11.08355503943118947 ) ) ;
#29921=CARTESIAN_POINT ( 'NONE',  ( 5.529263428287477744, 98.67268628210146630, -7.954856959092191815 ) ) ;
#29925=CARTESIAN_POINT ( 'NONE',  ( -9.465287035748106703, 52.20231371789854080, 2.064181346179061460 ) ) ;
#29929=CARTESIAN_POINT ( 'NONE',  ( 5.529263428287300108, 113.7273137178985678, 7.954856959092309943 ) ) ;
#29931=CARTESIAN_POINT ( 'NONE',  ( -12.53471296425189152, 25.17731371789855288, -2.311890736173453753 ) ) ;
#29933=CARTESIAN_POINT ( 'NONE',  ( -8.715434833791929847, 78.26018628210144357, -8.962234695871762469 ) ) ;
#29937=CARTESIAN_POINT ( 'NONE',  ( 0.1745138560725837118, 79.41018628210144925, -15.50000000000000533 ) ) ;
#29942=CARTESIAN_POINT ( 'NONE',  ( 9.534712964251941258, 109.0226862821014606, -1.715153634034235708 ) ) ;
#29944=CARTESIAN_POINT ( 'NONE',  ( 7.228626920339068285, 126.2726862821014606, -10.49813415415989581 ) ) ;
#29955=CARTESIAN_POINT ( 'NONE',  ( -3.796722387233185003, 17.41481371789854649, -8.710071997420207879 ) ) ;
#29960=CARTESIAN_POINT ( 'NONE',  ( -8.962234695871565293, 16.83981371789855430, -8.715434833792128799 ) ) ;
#29962=CARTESIAN_POINT ( 'NONE',  ( -15.50000000000000533, 126.0898137178985650, 0.1745138560722471477 ) ) ;
#29968=CARTESIAN_POINT ( 'NONE',  ( 10.49813415415989581, 137.7726862821014606, 7.228626920339068285 ) ) ;
#29974=CARTESIAN_POINT ( 'NONE',  ( 2.311890736173175753, 129.7226862821014777, 12.53471296425194836 ) ) ;
#29979=CARTESIAN_POINT ( 'NONE',  ( -13.04141134922759804, 133.1726862821014663, -8.927990412390657937 ) ) ;
#29981=CARTESIAN_POINT ( 'NONE',  ( -2.064181346179269738, 130.2976862821014379, 9.465287035748067623 ) ) ;
#29983=CARTESIAN_POINT ( 'NONE',  ( -12.46528703574805697, 31.39768628210144641, -2.660918448318280838 ) ) ;
#29989=CARTESIAN_POINT ( 'NONE',  ( 0.1745138560725837118, 116.2101862821014748, -15.50000000000000533 ) ) ;
#29991=CARTESIAN_POINT ( 'NONE',  ( -5.529263428287297444, 136.7273137178985110, -7.954856959092311719 ) ) ;
#29998=CARTESIAN_POINT ( 'NONE',  ( 0.1745138560723095977, 77.78981371789853938, 9.500000000000005329 ) ) ;
#30003=CARTESIAN_POINT ( 'NONE',  ( 12.50000000000000355, 84.68981371789854506, -0.1745138560722771515 ) ) ;
#30006=CARTESIAN_POINT ( 'NONE',  ( 6.932735513424201024, 46.45231371789855501, -10.69584247140429412 ) ) ;
#30012=CARTESIAN_POINT ( 'NONE',  ( -12.53471296425194836, 30.82268628210144001, 2.311890736173176641 ) ) ;
#30017=CARTESIAN_POINT ( 'NONE',  ( -12.53471296425189152, 89.57731371789856212, -2.311890736173453753 ) ) ;
#30022=CARTESIAN_POINT ( 'NONE',  ( -14.25334919248795096, 51.91481371789856070, 6.092822981423662299 ) ) ;
#30025=CARTESIAN_POINT ( 'NONE',  ( 2.311890736173175753, 83.72268628210143504, 12.53471296425194836 ) ) ;
#30026=CARTESIAN_POINT ( 'NONE',  ( -2.908627838312119351, 23.92268628210143788, -15.53471296425195369 ) ) ;
#30030=CARTESIAN_POINT ( 'NONE',  ( 8.927990412390657937, 52.67268628210144499, -13.04141134922759804 ) ) ;
#30036=CARTESIAN_POINT ( 'NONE',  ( 4.622313124798573369, 19.03518628210144925, 11.61527771782819940 ) ) ;
#30038=CARTESIAN_POINT ( 'NONE',  ( -2.064181346179062349, 137.3023137178985564, -9.465287035748106703 ) ) ;
#30044=CARTESIAN_POINT ( 'NONE',  ( 7.228626920338837358, 132.1273137178985451, 10.49813415416005036 ) ) ;
#30050=CARTESIAN_POINT ( 'NONE',  ( -4.622313124798576922, 51.23518628210143788, -11.61527771782819762 ) ) ;
#30058=CARTESIAN_POINT ( 'NONE',  ( 4.622313124798573369, 74.23518628210145209, 11.61527771782819940 ) ) ;
#30059=CARTESIAN_POINT ( 'NONE',  ( -15.46528703574811736, 15.40231371789854720, 3.257655550456946436 ) ) ;
#30065=CARTESIAN_POINT ( 'NONE',  ( -12.53471296425189152, 135.5773137178985621, -2.311890736173453753 ) ) ;
#30071=CARTESIAN_POINT ( 'NONE',  ( 10.83675517735179206, 120.3398137178985507, -11.08355503943118769 ) ) ;
#30075=CARTESIAN_POINT ( 'NONE',  ( 6.932735513423970097, 27.94768628210143646, 10.69584247140445044 ) ) ;
#30079=CARTESIAN_POINT ( 'NONE',  ( 0.1745138560725837118, 107.0101862821014578, -15.50000000000000533 ) ) ;
#30084=CARTESIAN_POINT ( 'NONE',  ( -9.534712964251941258, 40.02268628210144641, 1.715153634034234154 ) ) ;
#30089=CARTESIAN_POINT ( 'NONE',  ( 6.932735513423970097, 73.94768628210145778, 10.69584247140445044 ) ) ;
#30092=CARTESIAN_POINT ( 'NONE',  ( 5.529263428287477744, 52.67268628210144499, -7.954856959092191815 ) ) ;
#30104=CARTESIAN_POINT ( 'NONE',  ( 2.660918448318002838, 105.1023137178985536, 12.46528703574811558 ) ) ;
#30105=CARTESIAN_POINT ( 'NONE',  ( 2.660918448318279950, 107.2976862821014521, -12.46528703574805874 ) ) ;
#30111=CARTESIAN_POINT ( 'NONE',  ( 13.04141134922778988, 83.82731371789856212, -8.927990412390371944 ) ) ;
#30115=CARTESIAN_POINT ( 'NONE',  ( -6.594114490232312775, 96.66018628210144925, -6.840914352312096547 ) ) ;
#30117=CARTESIAN_POINT ( 'NONE',  ( -9.534712964251895073, 52.77731371789855785, -1.715153634034446428 ) ) ;
#30119=CARTESIAN_POINT ( 'NONE',  ( 9.500000000000005329, 112.2898137178985678, -0.1745138560723090149 ) ) ;
#30121=CARTESIAN_POINT ( 'NONE',  ( 10.49813415416005213, 37.82731371789854791, -7.228626920338837358 ) ) ;
#30122=CARTESIAN_POINT ( 'NONE',  ( 10.49813415415989581, 82.57268628210145778, 7.228626920339068285 ) ) ;
#30130=CARTESIAN_POINT ( 'NONE',  ( 5.233372021372432847, 92.34768628210142083, 8.152565276336710909 ) ) ;
#30132=CARTESIAN_POINT ( 'NONE',  ( -4.944772684328673229, 139.7851862821014493, 11.48171059495397728 ) ) ;
#30146=CARTESIAN_POINT ( 'NONE',  ( -1.715153634034442431, 13.67731371789853867, 9.534712964251900402 ) ) ;
#30152=CARTESIAN_POINT ( 'NONE',  ( 12.53471296425189330, 20.57731371789854435, 2.311890736173451533 ) ) ;
#30154=CARTESIAN_POINT ( 'NONE',  ( -6.092822981423666739, 127.8148137178985735, -14.25334919248795096 ) ) ;
#30160=CARTESIAN_POINT ( 'NONE',  ( 4.622313124798573369, 138.6351862821014720, 11.61527771782819940 ) ) ;
#30167=CARTESIAN_POINT ( 'NONE',  ( 8.962234695871762469, 135.7601862821014720, -8.715434833791931624 ) ) ;
#30171=CARTESIAN_POINT ( 'NONE',  ( 0.1745138560725837118, 134.6101862821014947, -15.50000000000000533 ) ) ;
#30173=CARTESIAN_POINT ( 'NONE',  ( 8.710071997420127943, 119.0851862821014606, 3.796722387233375073 ) ) ;
#30175=CARTESIAN_POINT ( 'NONE',  ( -7.228626920339069173, 29.67268628210144499, 10.49813415415989581 ) ) ;
#30181=CARTESIAN_POINT ( 'NONE',  ( -15.46528703574804986, 114.1976862821014578, -3.257655550457287497 ) ) ;
#30183=CARTESIAN_POINT ( 'NONE',  ( -7.954856959092191815, 4.372686282101438948, -5.529263428287477744 ) ) ;
#30189=CARTESIAN_POINT ( 'NONE',  ( 9.465287035748106703, 75.20231371789854791, -2.064181346179063237 ) ) ;
#30192=CARTESIAN_POINT ( 'NONE',  ( -11.61527771782809282, 89.86481371789855643, -4.622313124798832717 ) ) ;
#30194=CARTESIAN_POINT ( 'NONE',  ( -10.52346919520418922, 142.9999999999999432, 8.647714196784560770 ) ) ;
#30196=CARTESIAN_POINT ( 'NONE',  ( -6.932735513424201912, 51.05231371789854933, 10.69584247140429412 ) ) ;
#30200=CARTESIAN_POINT ( 'NONE',  ( -6.932735513423968321, 23.34768628210144570, -10.69584247140445221 ) ) ;
#30206=CARTESIAN_POINT ( 'NONE',  ( -4.622313124798826500, 78.36481371789855643, 11.61527771782809637 ) ) ;
#30213=CARTESIAN_POINT ( 'NONE',  ( -11.08355503943118592, 62.83981371789855785, -10.83675517735179383 ) ) ;
#30216=CARTESIAN_POINT ( 'NONE',  ( -4.622313124798576922, 78.83518628210146062, -11.61527771782819762 ) ) ;
#30217=CARTESIAN_POINT ( 'NONE',  ( 2.908627838312118019, 19.32268628210144001, 15.53471296425195369 ) ) ;
#30222=CARTESIAN_POINT ( 'NONE',  ( 10.83675517735155225, 55.26018628210144357, 11.08355503943142573 ) ) ;
#30229=CARTESIAN_POINT ( 'NONE',  ( 8.962234695871762469, 25.36018628210144499, -8.715434833791931624 ) ) ;
#30231=CARTESIAN_POINT ( 'NONE',  ( -8.152565276336593669, 136.1523137178985507, -5.233372021372610483 ) ) ;
#30235=CARTESIAN_POINT ( 'NONE',  ( -2.660918448318005058, 128.1023137178985678, -12.46528703574811558 ) ) ;
#30241=CARTESIAN_POINT ( 'NONE',  ( -4.622313124798576922, 32.83518628210143930, -11.61527771782819762 ) ) ;
#30242=ORIENTED_EDGE ( 'NONE', *, *, #11135, .T. ) ;
#30243=ORIENTED_EDGE ( 'NONE', *, *, #24913, .T. ) ;
#30249=CARTESIAN_POINT ( 'NONE',  ( -7.228626920339069173, 84.87268628210146915, 10.49813415415989581 ) ) ;
#30250=CARTESIAN_POINT ( 'NONE',  ( 8.927990412390657937, 135.4726862821014777, -13.04141134922759804 ) ) ;
#30256=CARTESIAN_POINT ( 'NONE',  ( -2.311890736173448424, 133.2773137178985507, 12.53471296425189330 ) ) ;
#30264=CARTESIAN_POINT ( 'NONE',  ( 15.53471296425188797, 121.7773137178985650, 2.908627838312457747 ) ) ;
#30271=CARTESIAN_POINT ( 'NONE',  ( 8.927990412390657937, 98.67268628210146630, -13.04141134922759804 ) ) ;
#30275=CARTESIAN_POINT ( 'NONE',  ( 0.1745138560725194299, 33.41018628210144925, -9.500000000000005329 ) ) ;
#30278=CARTESIAN_POINT ( 'NONE',  ( -10.49813415415989581, 77.97268628210144925, -7.228626920339068285 ) ) ;
#30281=CARTESIAN_POINT ( 'NONE',  ( -9.465287035748065847, 40.59768628210144215, -2.064181346179273735 ) ) ;
#30292=CARTESIAN_POINT ( 'NONE',  ( -12.46528703574811558, 89.00231371789855928, 2.660918448318003726 ) ) ;
#30293=CARTESIAN_POINT ( 'NONE',  ( 6.932735513423970097, 110.7476862821014691, 10.69584247140445044 ) ) ;
#30298=CARTESIAN_POINT ( 'NONE',  ( 13.04141134922778988, 65.42731371789857064, -8.927990412390371944 ) ) ;
#30305=CARTESIAN_POINT ( 'NONE',  ( -2.064181346179062349, 63.70231371789854791, -9.465287035748106703 ) ) ;
#30307=CARTESIAN_POINT ( 'NONE',  ( -0.1745138560723084320, 109.9898137178985706, -9.500000000000005329 ) ) ;
#30309=CARTESIAN_POINT ( 'NONE',  ( 7.228626920338837358, 30.92731371789854222, 10.49813415416005036 ) ) ;
#30311=CARTESIAN_POINT ( 'NONE',  ( 7.228626920339068285, 89.47268628210144925, -10.49813415415989581 ) ) ;
#30319=CARTESIAN_POINT ( 'NONE',  ( 7.954856959092191815, 100.9726862821014635, 5.529263428287477744 ) ) ;
#30321=CARTESIAN_POINT ( 'NONE',  ( -8.962234695871760692, 140.3601862821014379, 8.715434833791933400 ) ) ;
#30334=CARTESIAN_POINT ( 'NONE',  ( -12.50000000000000355, 135.2898137178985678, 0.1745138560722786503 ) ) ;
#30339=CARTESIAN_POINT ( 'NONE',  ( -12.50000000000000355, 34.08981371789854364, 0.1745138560722786503 ) ) ;
#30341=CARTESIAN_POINT ( 'NONE',  ( -5.770363421894122880, 124.3648137178985849, 14.38691631536194393 ) ) ;
#30349=CARTESIAN_POINT ( 'NONE',  ( -12.53471296425194836, 141.2226862821014493, 2.311890736173176641 ) ) ;
#30357=CARTESIAN_POINT ( 'NONE',  ( -8.962234695871760692, 140.3601862821014379, 8.715434833791933400 ) ) ;
#30361=CARTESIAN_POINT ( 'NONE',  ( -15.46528703574804986, 114.1976862821014578, -3.257655550457287497 ) ) ;
#30363=CARTESIAN_POINT ( 'NONE',  ( -7.954856959092191815, 114.7726862821014322, -5.529263428287477744 ) ) ;
#30365=CARTESIAN_POINT ( 'NONE',  ( 11.48171059495397728, 17.88518628210143646, 4.944772684328674117 ) ) ;
#30369=CARTESIAN_POINT ( 'NONE',  ( -8.152565276336710909, 85.44768628210142936, 5.233372021372435512 ) ) ;
#30372=CARTESIAN_POINT ( 'NONE',  ( 8.152565276336593669, 131.5523137178985564, 5.233372021372610483 ) ) ;
#30379=CARTESIAN_POINT ( 'NONE',  ( 9.534712964251900402, 75.77731371789855075, 1.715153634034445540 ) ) ;
#30383=CARTESIAN_POINT ( 'NONE',  ( -2.311890736173447980, 87.27731371789856496, 12.53471296425189330 ) ) ;
#30387=CARTESIAN_POINT ( 'NONE',  ( -10.49813415416004858, 51.62731371789855217, 7.228626920338839135 ) ) ;
#30391=CARTESIAN_POINT ( 'NONE',  ( -4.622313124798576922, 14.43518628210144250, -11.61527771782819762 ) ) ;
#30397=CARTESIAN_POINT ( 'NONE',  ( -10.69584247140429412, 71.75231371789855928, -6.932735513424201024 ) ) ;
#30403=CARTESIAN_POINT ( 'NONE',  ( -15.53471296425188442, 61.97731371789853938, -2.908627838312459080 ) ) ;
#30406=CARTESIAN_POINT ( 'NONE',  ( -6.932735513423968321, 60.14768628210144641, -10.69584247140445221 ) ) ;
#30407=CARTESIAN_POINT ( 'NONE',  ( -14.25334919248782306, 31.68518628210144428, -6.092822981423979378 ) ) ;
#30411=CARTESIAN_POINT ( 'NONE',  ( 3.257655550457285720, 33.69768628210143646, -15.46528703574804986 ) ) ;
#30419=CARTESIAN_POINT ( 'NONE',  ( 12.50000000000000355, 17.31018628210144428, 0.1745138560725507937 ) ) ;
#30421=CARTESIAN_POINT ( 'NONE',  ( -9.534712964251895073, 126.3773137178985309, -1.715153634034446428 ) ) ;
#30427=CARTESIAN_POINT ( 'NONE',  ( -10.69584247140429412, 136.1523137178985792, -6.932735513424201024 ) ) ;
#30434=CARTESIAN_POINT ( 'NONE',  ( -11.48171059495397373, 31.68518628210144428, -4.944772684328680334 ) ) ;
#30442=CARTESIAN_POINT ( 'NONE',  ( 0.1745138560725515708, 79.41018628210144925, -12.50000000000000355 ) ) ;
#30443=CARTESIAN_POINT ( 'NONE',  ( -13.23911966647218463, 131.4476862821014436, 8.632099005475506459 ) ) ;
#30452=CARTESIAN_POINT ( 'NONE',  ( -7.228626920338836470, 127.5273137178985792, -10.49813415416005213 ) ) ;
#30459=CARTESIAN_POINT ( 'NONE',  ( 3.257655550456945548, 114.3023137178985422, 15.46528703574811736 ) ) ;
#30466=CARTESIAN_POINT ( 'NONE',  ( -13.23911966647218463, 85.44768628210142936, 8.632099005475506459 ) ) ;
#30469=CARTESIAN_POINT ( 'NONE',  ( -6.594114490232312775, 32.26018628210145067, -6.840914352312096547 ) ) ;
#30473=CARTESIAN_POINT ( 'NONE',  ( -8.962234695871760692, 85.16018628210144925, 8.715434833791933400 ) ) ;
#30476=CARTESIAN_POINT ( 'NONE',  ( 1.715153634034233487, 37.72268628210143504, 9.534712964251941258 ) ) ;
#30486=CARTESIAN_POINT ( 'NONE',  ( 11.61527771782809637, 76.06481371789855928, 4.622313124798827388 ) ) ;
#30487=CARTESIAN_POINT ( 'NONE',  ( -10.69584247140444866, 85.44768628210144357, 6.932735513423972762 ) ) ;
#30492=CARTESIAN_POINT ( 'NONE',  ( 10.83675517735179206, 65.13981371789854791, -11.08355503943118769 ) ) ;
#30499=CARTESIAN_POINT ( 'NONE',  ( -2.064181346179062349, 54.50231371789855928, -9.465287035748106703 ) ) ;
#30501=CARTESIAN_POINT ( 'NONE',  ( -3.796722387233185003, 91.01481371789856212, -8.710071997420207879 ) ) ;
#30503=CARTESIAN_POINT ( 'NONE',  ( -0.1745138560722763466, 27.18981371789855217, -12.50000000000000355 ) ) ;
#30505=CARTESIAN_POINT ( 'NONE',  ( -12.46528703574805697, 77.39768628210144641, -2.660918448318280838 ) ) ;
#30513=CARTESIAN_POINT ( 'NONE',  ( 2.064181346179272847, 88.89768628210146062, -9.465287035748065847 ) ) ;
#30515=CARTESIAN_POINT ( 'NONE',  ( 2.660918448318279950, 134.8976862821014890, -12.46528703574805697 ) ) ;
#30516=CARTESIAN_POINT ( 'NONE',  ( -6.406268989994019059, 143.0000000000000853, 10.69826447808074299 ) ) ;
#30526=CARTESIAN_POINT ( 'NONE',  ( -6.932735513424201912, 133.8523137178985678, 10.69584247140429412 ) ) ;
#30527=CARTESIAN_POINT ( 'NONE',  ( 2.311890736173175753, 138.9226862821014663, 12.53471296425194659 ) ) ;
#30536=CARTESIAN_POINT ( 'NONE',  ( 8.927990412390371944, 104.5273137178985650, 13.04141134922778811 ) ) ;
#30544=CARTESIAN_POINT ( 'NONE',  ( 0.1745138560725515708, 134.6101862821014663, -12.50000000000000355 ) ) ;
#30552=CARTESIAN_POINT ( 'NONE',  ( -6.932735513423968321, 133.7476862821014549, -10.69584247140445221 ) ) ;
#30557=CARTESIAN_POINT ( 'NONE',  ( -10.83675517735155047, 124.2601862821014578, -11.08355503943142750 ) ) ;
#30558=CARTESIAN_POINT ( 'NONE',  ( -9.534712964251941258, 113.6226862821014549, 1.715153634034234154 ) ) ;
#30561=CARTESIAN_POINT ( 'NONE',  ( -10.69584247140444866, 11.84768628210144925, 6.932735513423972762 ) ) ;
#30565=CARTESIAN_POINT ( 'NONE',  ( 9.534712964251941258, 81.42268628210145209, -1.715153634034235708 ) ) ;
#30567=CARTESIAN_POINT ( 'NONE',  ( -7.954856959092309943, 125.2273137178985394, 5.529263428287300108 ) ) ;
#30575=CARTESIAN_POINT ( 'NONE',  ( 5.529263428287300108, 58.52731371789855785, 7.954856959092309943 ) ) ;
#30578=CARTESIAN_POINT ( 'NONE',  ( -2.311890736173447980, 78.07731371789856212, 12.53471296425189330 ) ) ;
#30582=CARTESIAN_POINT ( 'NONE',  ( 12.53471296425189330, 20.57731371789854435, 2.311890736173451977 ) ) ;
#30585=CARTESIAN_POINT ( 'NONE',  ( -4.622313124798576922, 23.63518628210144357, -11.61527771782819762 ) ) ;
#30590=CARTESIAN_POINT ( 'NONE',  ( -6.932735513424201912, 60.25231371789855217, 10.69584247140429412 ) ) ;
#30595=CARTESIAN_POINT ( 'NONE',  ( -13.23911966647199812, 34.95231371789854080, -8.632099005475788900 ) ) ;
#30599=CARTESIAN_POINT ( 'NONE',  ( 12.50000000000000355, 72.51018628210145778, 0.1745138560725507937 ) ) ;
#30600=CARTESIAN_POINT ( 'NONE',  ( 2.908627838312118019, 10.12268628210144428, 15.53471296425195369 ) ) ;
#30604=CARTESIAN_POINT ( 'NONE',  ( -2.908627838312119351, 23.92268628210143788, -15.53471296425195369 ) ) ;
#30612=CARTESIAN_POINT ( 'NONE',  ( -6.594114490232462877, 106.5398137178985536, 6.840914352311949109 ) ) ;
#30622=CARTESIAN_POINT ( 'NONE',  ( 12.53471296425194659, 35.42268628210144499, -2.311890736173178418 ) ) ;
#30630=CARTESIAN_POINT ( 'NONE',  ( -2.311890736173176641, 69.92268628210146630, -12.53471296425194836 ) ) ;
#30631=CARTESIAN_POINT ( 'NONE',  ( -11.08355503943142573, 140.3601862821014663, 10.83675517735155402 ) ) ;
#30636=CARTESIAN_POINT ( 'NONE',  ( -4.944772684328424539, 118.6148137178985564, -11.48171059495408031 ) ) ;
#30642=CARTESIAN_POINT ( 'NONE',  ( -6.092822981423666739, 100.2148137178985650, -14.25334919248795096 ) ) ;
#30647=CARTESIAN_POINT ( 'NONE',  ( 8.715434833791931624, 119.6601862821014493, 8.962234695871760692 ) ) ;
#30648=CARTESIAN_POINT ( 'NONE',  ( -11.08355503943142573, 75.96018628210144641, 10.83675517735155402 ) ) ;
#30651=CARTESIAN_POINT ( 'NONE',  ( -14.38691631536207183, 76.53518628210146346, 5.770363421893814682 ) ) ;
#30655=CARTESIAN_POINT ( 'NONE',  ( -5.233372021372430183, 32.54768628210143788, -8.152565276336710909 ) ) ;
#30659=CARTESIAN_POINT ( 'NONE',  ( -12.50000000000000355, 49.51018628210145067, -0.1745138560725492671 ) ) ;
#30661=CARTESIAN_POINT ( 'NONE',  ( -6.594114490232312775, 41.46018628210145351, -6.840914352312096547 ) ) ;
#30672=CARTESIAN_POINT ( 'NONE',  ( 2.311890736173452865, 91.87731371789855928, -12.53471296425189152 ) ) ;
#30673=CARTESIAN_POINT ( 'NONE',  ( 11.61527771782819940, 90.33518628210144641, -4.622313124798573369 ) ) ;
#30677=CARTESIAN_POINT ( 'NONE',  ( -13.04141134922778456, 60.82731371789854080, 8.927990412390377273 ) ) ;
#30683=CARTESIAN_POINT ( 'NONE',  ( 0.1745138560723095977, 40.98981371789854933, 9.500000000000005329 ) ) ;
#30686=CARTESIAN_POINT ( 'NONE',  ( -9.465287035748106703, 98.20231371789854791, 2.064181346179061460 ) ) ;
#30688=CARTESIAN_POINT ( 'NONE',  ( -2.311890736173448424, 22.87731371789854151, 12.53471296425189330 ) ) ;
#30689=CARTESIAN_POINT ( 'NONE',  ( 2.311890736173175753, 74.52268628210146062, 12.53471296425194836 ) ) ;
#30697=CARTESIAN_POINT ( 'NONE',  ( 9.465287035748067623, 100.3976862821014606, 2.064181346179272847 ) ) ;
#30699=CARTESIAN_POINT ( 'NONE',  ( -7.228626920339069173, 130.8726862821014834, 10.49813415415989581 ) ) ;
#30700=CARTESIAN_POINT ( 'NONE',  ( -6.962373209266437435, 142.9999999999999716, 9.648466868844547406 ) ) ;
#30713=CARTESIAN_POINT ( 'NONE',  ( -5.529263428287297444, 7.927313717898536005, -7.954856959092311719 ) ) ;
#30718=CARTESIAN_POINT ( 'NONE',  ( 4.622313124798831829, 9.364813717898545775, -11.61527771782809282 ) ) ;
#30720=CARTESIAN_POINT ( 'NONE',  ( 13.23911966647199812, 103.9523137178985763, 8.632099005475788900 ) ) ;
#30726=CARTESIAN_POINT ( 'NONE',  ( 10.49813415415989581, 110.1726862821014521, 7.228626920339068285 ) ) ;
#30739=CARTESIAN_POINT ( 'NONE',  ( 14.38691631536207538, 127.1351862821014720, -5.770363421893813793 ) ) ;
#30742=CARTESIAN_POINT ( 'NONE',  ( 0.1745138560725515708, 5.810186282101447830, -12.50000000000000355 ) ) ;
#30746=CARTESIAN_POINT ( 'NONE',  ( 8.710071997420127943, 82.28518628210146346, 3.796722387233375073 ) ) ;
#30747=CARTESIAN_POINT ( 'NONE',  ( 6.840914352311949109, 122.6398137178985479, 6.594114490232462877 ) ) ;
#30753=CARTESIAN_POINT ( 'NONE',  ( 8.152565276336593669, 57.95231371789854791, 5.233372021372610483 ) ) ;
#30758=CARTESIAN_POINT ( 'NONE',  ( 8.715434833792128799, 65.13981371789854791, -8.962234695871567070 ) ) ;
#30762=CARTESIAN_POINT ( 'NONE',  ( -12.46528703574811558, 33.80231371789854933, 2.660918448318003726 ) ) ;
#30765=CARTESIAN_POINT ( 'NONE',  ( -4.622313124798576922, 5.235186282101428112, -11.61527771782819762 ) ) ;
#30769=CARTESIAN_POINT ( 'NONE',  ( 8.962234695871567070, 67.43981371789855928, 8.715434833792127023 ) ) ;
#30774=CARTESIAN_POINT ( 'NONE',  ( -14.25334919248795096, 42.71481371789855075, 6.092822981423662299 ) ) ;
#30776=CARTESIAN_POINT ( 'NONE',  ( -10.69584247140444866, 30.24768628210144783, 6.932735513423972762 ) ) ;
#30778=CARTESIAN_POINT ( 'NONE',  ( -7.228626920339069173, 66.47268628210144925, 10.49813415415989581 ) ) ;
#30779=CARTESIAN_POINT ( 'NONE',  ( 15.46528703574804986, 8.397686282101439303, 3.257655550457285720 ) ) ;
#30783=CARTESIAN_POINT ( 'NONE',  ( 11.08355503943142750, 34.56018628210144783, -10.83675517735155225 ) ) ;
#30789=CARTESIAN_POINT ( 'NONE',  ( 12.53471296425194836, 7.822686282101448896, -2.311890736173178418 ) ) ;
#30791=CARTESIAN_POINT ( 'NONE',  ( -7.954856959092309943, 106.8273137178985479, 5.529263428287300108 ) ) ;
#30795=CARTESIAN_POINT ( 'NONE',  ( -10.69584247140429412, 108.5523137178985564, -6.932735513424201024 ) ) ;
#30801=CARTESIAN_POINT ( 'NONE',  ( 0.1745138560725515708, 33.41018628210144925, -12.50000000000000355 ) ) ;
#30810=CARTESIAN_POINT ( 'NONE',  ( -12.50000000000000355, 67.91018628210144925, -0.1745138560725492671 ) ) ;
#30811=CARTESIAN_POINT ( 'NONE',  ( 5.770363421894130873, 9.364813717898543999, -14.38691631536193860 ) ) ;
#30817=CARTESIAN_POINT ( 'NONE',  ( -12.46528703574811558, 125.8023137178985706, 2.660918448318003726 ) ) ;
#30824=CARTESIAN_POINT ( 'NONE',  ( -8.632099005475794229, 97.05231371789855643, 13.23911966647199812 ) ) ;
#30828=CARTESIAN_POINT ( 'NONE',  ( -11.48171059495397373, 123.6851862821014549, -4.944772684328680334 ) ) ;
#30829=CARTESIAN_POINT ( 'NONE',  ( -14.25334919248782306, 59.28518628210144925, -6.092822981423979378 ) ) ;
#30832=CARTESIAN_POINT ( 'NONE',  ( -3.257655550457281723, 93.49768628210142651, 15.46528703574804986 ) ) ;
#30835=CARTESIAN_POINT ( 'NONE',  ( -9.534712964251941258, 30.82268628210143291, 1.715153634034234154 ) ) ;
#30839=CARTESIAN_POINT ( 'NONE',  ( 7.228626920339068285, 52.67268628210144499, -10.49813415415989581 ) ) ;
#30842=CARTESIAN_POINT ( 'NONE',  ( 3.796722387233379514, 33.98518628210143788, -8.710071997420127943 ) ) ;
#30852=CARTESIAN_POINT ( 'NONE',  ( -10.49813415416004858, 88.42731371789858485, 7.228626920338839135 ) ) ;
#30853=CARTESIAN_POINT ( 'NONE',  ( 2.311890736173175753, 83.72268628210144925, 12.53471296425194659 ) ) ;
#30858=CARTESIAN_POINT ( 'NONE',  ( 14.25334919248795451, 56.51481371789856212, -6.092822981423661410 ) ) ;
#30863=CARTESIAN_POINT ( 'NONE',  ( 7.954856959092311719, 37.82731371789854080, -5.529263428287300108 ) ) ;
#30867=CARTESIAN_POINT ( 'NONE',  ( -8.843639120294245259, 99.06481371789857349, -3.474262827703533230 ) ) ;
#30869=CARTESIAN_POINT ( 'NONE',  ( 8.715434833792128799, 19.13981371789855146, -8.962234695871567070 ) ) ;
#30870=CARTESIAN_POINT ( 'NONE',  ( 12.46528703574805874, 72.79768628210146630, 2.660918448318279950 ) ) ;
#30872=CARTESIAN_POINT ( 'NONE',  ( -12.50000000000000355, 143.0000000000000284, -1.353084311261909534E-13 ) ) ;
#30877=CARTESIAN_POINT ( 'NONE',  ( 3.474262827703335166, 101.8351862821014606, 8.843639120294326972 ) ) ;
#30880=CARTESIAN_POINT ( 'NONE',  ( -8.962234695871760692, 112.7601862821014720, 8.715434833791933400 ) ) ;
#30893=CARTESIAN_POINT ( 'NONE',  ( 0.1745138560722779009, 142.1898137178985735, 12.50000000000000355 ) ) ;
#30899=CARTESIAN_POINT ( 'NONE',  ( -12.53471296425189152, 15.97731371789853938, -2.311890736173453309 ) ) ;
#30901=CARTESIAN_POINT ( 'NONE',  ( -14.25334919248795096, 116.3148137178985735, 6.092822981423662299 ) ) ;
#30908=CARTESIAN_POINT ( 'NONE',  ( -6.932735513423968321, 115.3476862821014635, -10.69584247140445221 ) ) ;
#30915=CARTESIAN_POINT ( 'NONE',  ( 11.61527771782819940, 117.9351862821014549, -4.622313124798573369 ) ) ;
#30923=CARTESIAN_POINT ( 'NONE',  ( -15.53471296425195369, 122.8226862821014294, 2.908627838312118019 ) ) ;
#30925=CARTESIAN_POINT ( 'NONE',  ( -12.53471296425194836, 12.42268628210144321, 2.311890736173176641 ) ) ;
#30929=CARTESIAN_POINT ( 'NONE',  ( 8.843639120294328748, 81.13518628210145778, -3.474262827703334722 ) ) ;
#30931=CARTESIAN_POINT ( 'NONE',  ( -6.840914352311947333, 127.2398137178985422, -6.594114490232462877 ) ) ;
#30937=CARTESIAN_POINT ( 'NONE',  ( 8.710071997420211432, 65.71481371789855075, -3.796722387233181895 ) ) ;
#30941=CARTESIAN_POINT ( 'NONE',  ( 12.50000000000000355, 57.08981371789855075, -0.1745138560722771515 ) ) ;
#30946=CARTESIAN_POINT ( 'NONE',  ( 8.962234695871567070, 30.63981371789854791, 8.715434833792127023 ) ) ;
#30957=CARTESIAN_POINT ( 'NONE',  ( 12.53471296425189330, 66.57731371789856212, 2.311890736173451977 ) ) ;
#30962=CARTESIAN_POINT ( 'NONE',  ( 10.83675517735179206, 37.53981371789855359, -11.08355503943118769 ) ) ;
#30964=CARTESIAN_POINT ( 'NONE',  ( -11.48171059495397373, 22.48518628210144499, -4.944772684328680334 ) ) ;
#30966=CARTESIAN_POINT ( 'NONE',  ( 12.46528703574805874, 63.59768628210145636, 2.660918448318279950 ) ) ;
#30967=CARTESIAN_POINT ( 'NONE',  ( -2.908627838312119351, 5.522686282101450850, -15.53471296425195369 ) ) ;
#30972=CARTESIAN_POINT ( 'NONE',  ( -3.257655550457281723, 29.09768628210144925, 15.46528703574804986 ) ) ;
#30978=CARTESIAN_POINT ( 'NONE',  ( -11.48171059495397373, 4.085186282101443744, -4.944772684328680334 ) ) ;
#30980=CARTESIAN_POINT ( 'NONE',  ( -5.233372021372612259, 115.4523137178985479, 8.152565276336593669 ) ) ;
#30987=CARTESIAN_POINT ( 'NONE',  ( 12.46528703574811558, 121.2023137178985621, -2.660918448318005947 ) ) ;
#30993=CARTESIAN_POINT ( 'NONE',  ( -12.50000000000000355, 40.31018628210144783, -0.1745138560725492671 ) ) ;
#31001=CARTESIAN_POINT ( 'NONE',  ( -8.962234695871760692, 66.76018628210145778, 8.715434833791933400 ) ) ;
#31007=CARTESIAN_POINT ( 'NONE',  ( 10.69584247140429589, 122.3523137178985678, 6.932735513424201024 ) ) ;
#31012=CARTESIAN_POINT ( 'NONE',  ( 11.08355503943118769, 95.03981371789855359, 10.83675517735179028 ) ) ;
#31015=CARTESIAN_POINT ( 'NONE',  ( 4.944772684328679446, 125.9851862821014521, -11.48171059495397373 ) ) ;
#31016=CARTESIAN_POINT ( 'NONE',  ( -8.632099005475501130, 69.34768628210143504, -13.23911966647218996 ) ) ;
#31019=CARTESIAN_POINT ( 'NONE',  ( 15.46528703574804986, 91.19768628210145778, 3.257655550457285720 ) ) ;
#31023=CARTESIAN_POINT ( 'NONE',  ( -9.465287035748065847, 12.99768628210143362, -2.064181346179273735 ) ) ;
#31027=CARTESIAN_POINT ( 'NONE',  ( -2.660918448318275509, 56.69768628210145067, 12.46528703574805874 ) ) ;
#31030=CARTESIAN_POINT ( 'NONE',  ( 6.840914352312096547, 34.56018628210144783, -6.594114490232313663 ) ) ;
#31042=CARTESIAN_POINT ( 'NONE',  ( -8.715434833792127023, 88.13981371789856212, 8.962234695871568846 ) ) ;
#31043=CARTESIAN_POINT ( 'NONE',  ( -2.660918448318275509, 84.29768628210146630, 12.46528703574805874 ) ) ;
#31048=CARTESIAN_POINT ( 'NONE',  ( -8.927990412390371944, 63.12731371789852375, -13.04141134922778988 ) ) ;
#31053=CARTESIAN_POINT ( 'NONE',  ( 5.529263428287300108, 40.12731371789853796, 7.954856959092309943 ) ) ;
#31056=CARTESIAN_POINT ( 'NONE',  ( 6.594114490232462877, 101.9398137178985735, -6.840914352311949109 ) ) ;
#31058=CARTESIAN_POINT ( 'NONE',  ( 7.228626920338837358, 12.52731371789855785, 10.49813415416005036 ) ) ;
#31059=CARTESIAN_POINT ( 'NONE',  ( 8.715434833791931624, 55.26018628210144357, 8.962234695871760692 ) ) ;
#31067=CARTESIAN_POINT ( 'NONE',  ( 8.843639120294328748, 71.93518628210142651, -3.474262827703334722 ) ) ;
#31070=CARTESIAN_POINT ( 'NONE',  ( 0.1745138560725515708, 116.2101862821014606, -12.50000000000000355 ) ) ;
#31082=CARTESIAN_POINT ( 'NONE',  ( -8.715434833792127023, 134.1398137178985621, 8.962234695871568846 ) ) ;
#31087=CARTESIAN_POINT ( 'NONE',  ( -11.61527771782809282, 7.064813717898549505, -4.622313124798832717 ) ) ;
#31089=CARTESIAN_POINT ( 'NONE',  ( -15.46528703574811736, 116.6023137178985394, 3.257655550456946436 ) ) ;
#31096=CARTESIAN_POINT ( 'NONE',  ( -2.311890736173176641, 106.7226862821014635, -12.53471296425194836 ) ) ;
#31103=CARTESIAN_POINT ( 'NONE',  ( -8.962234695871760692, 121.9601862821014464, 8.715434833791933400 ) ) ;
#31110=CARTESIAN_POINT ( 'NONE',  ( -14.38691631536207183, 113.3351862821014606, 5.770363421893814682 ) ) ;
#31111=CARTESIAN_POINT ( 'NONE',  ( -8.962234695871760692, 20.76018628210144001, 8.715434833791933400 ) ) ;
#31117=CARTESIAN_POINT ( 'NONE',  ( 7.954856959092191815, 73.37268628210144072, 5.529263428287477744 ) ) ;
#31126=CARTESIAN_POINT ( 'NONE',  ( -1.715153634034442431, 50.47731371789854649, 9.534712964251900402 ) ) ;
#31130=CARTESIAN_POINT ( 'NONE',  ( -2.660918448318005058, 54.50231371789855928, -12.46528703574811558 ) ) ;
#31133=CARTESIAN_POINT ( 'NONE',  ( 8.715434833792128799, 28.33981371789855075, -8.962234695871567070 ) ) ;
#31148=CARTESIAN_POINT ( 'NONE',  ( 8.927990412390371944, 40.12731371789853796, 13.04141134922778811 ) ) ;
#31150=CARTESIAN_POINT ( 'NONE',  ( 4.944772684328679446, 15.58518628210145351, -11.48171059495397373 ) ) ;
#31151=CARTESIAN_POINT ( 'NONE',  ( 4.622313124798573369, 74.23518628210145209, 11.61527771782819940 ) ) ;
#31152=CARTESIAN_POINT ( 'NONE',  ( 14.25334919248782661, 17.88518628210143646, 6.092822981423971385 ) ) ;
#31156=CARTESIAN_POINT ( 'NONE',  ( 13.23911966647218996, 34.84768628210143504, -8.632099005475504683 ) ) ;
#31164=CARTESIAN_POINT ( 'NONE',  ( -6.840914352311947333, 108.8398137178985507, -6.594114490232462877 ) ) ;
#31171=CARTESIAN_POINT ( 'NONE',  ( 12.53471296425189330, 112.5773137178985621, 2.311890736173451533 ) ) ;
#31183=CARTESIAN_POINT ( 'NONE',  ( 10.49813415415989581, 64.17268628210143788, 7.228626920339068285 ) ) ;
#31189=CARTESIAN_POINT ( 'NONE',  ( -4.944772684328424539, 127.8148137178985735, -11.48171059495408031 ) ) ;
#31194=CARTESIAN_POINT ( 'NONE',  ( -11.08355503943118592, 99.63981371789857633, -10.83675517735179383 ) ) ;
#31198=CARTESIAN_POINT ( 'NONE',  ( -11.48171059495397373, 114.4851862821014521, -4.944772684328680334 ) ) ;
#31199=CARTESIAN_POINT ( 'NONE',  ( 15.50000000000000533, 63.31018628210144783, 0.1745138560725827404 ) ) ;
#31203=CARTESIAN_POINT ( 'NONE',  ( 15.50000000000000533, 90.91018628210146346, 0.1745138560725827404 ) ) ;
#31205=CARTESIAN_POINT ( 'NONE',  ( 0.1745138560725194299, 15.01018628210143291, -9.500000000000005329 ) ) ;
#31207=CARTESIAN_POINT ( 'NONE',  ( -10.49813415415989581, 59.57268628210145778, -7.228626920339068285 ) ) ;
#31210=CARTESIAN_POINT ( 'NONE',  ( -9.534712964251941258, 30.82268628210143291, 1.715153634034234154 ) ) ;
#31221=CARTESIAN_POINT ( 'NONE',  ( -12.46528703574805874, 86.59768628210146346, -2.660918448318280838 ) ) ;
#31227=CARTESIAN_POINT ( 'NONE',  ( 14.25334919248795451, 47.31481371789856638, -6.092822981423661410 ) ) ;
#31234=CARTESIAN_POINT ( 'NONE',  ( -9.534712964251895073, 34.37731371789854506, -1.715153634034446428 ) ) ;
#31236=CARTESIAN_POINT ( 'NONE',  ( 9.500000000000005329, 103.0898137178985792, -0.1745138560723090149 ) ) ;
#31238=CARTESIAN_POINT ( 'NONE',  ( -8.632099005475794229, 143.0523137178985280, 13.23911966647199812 ) ) ;
#31240=CARTESIAN_POINT ( 'NONE',  ( 11.48171059495397728, 63.88518628210145067, 4.944772684328674117 ) ) ;
#31248=CARTESIAN_POINT ( 'NONE',  ( 7.954856959092191815, 82.57268628210144357, 5.529263428287477744 ) ) ;
#31250=( GEOMETRIC_REPRESENTATION_CONTEXT ( 3 ) GLOBAL_UNCERTAINTY_ASSIGNED_CONTEXT ( ( #33969 ) ) GLOBAL_UNIT_ASSIGNED_CONTEXT ( ( #32358, #18345, #35014 ) ) REPRESENTATION_CONTEXT ( 'NONE', 'WORKASPACE' ) );
#31252=CARTESIAN_POINT ( 'NONE',  ( -10.69584247140444866, 122.2476862821014549, 6.932735513423972762 ) ) ;
#31264=CARTESIAN_POINT ( 'NONE',  ( 10.69584247140429589, 122.3523137178985678, 6.932735513424201024 ) ) ;
#31265=CARTESIAN_POINT ( 'NONE',  ( 12.46528703574805874, 137.1976862821014720, 2.660918448318279950 ) ) ;
#31270=CARTESIAN_POINT ( 'NONE',  ( 7.228626920338837358, 12.52731371789855785, 10.49813415416005036 ) ) ;
#31272=CARTESIAN_POINT ( 'NONE',  ( -13.23911966647199812, 108.5523137178985422, -8.632099005475788900 ) ) ;
#31277=CARTESIAN_POINT ( 'NONE',  ( -8.715434833791929847, 115.0601862821014549, -8.962234695871762469 ) ) ;
#31283=CARTESIAN_POINT ( 'NONE',  ( 12.53471296425194836, 118.2226862821014635, -2.311890736173178418 ) ) ;
#31289=CARTESIAN_POINT ( 'NONE',  ( -10.83675517735155047, 105.8601862821014379, -11.08355503943142750 ) ) ;
#31290=CARTESIAN_POINT ( 'NONE',  ( 6.932735513423970097, 9.547686282101450317, 10.69584247140445044 ) ) ;
#31292=CARTESIAN_POINT ( 'NONE',  ( 8.152565276336714462, 126.8476862821014635, -5.233372021372432847 ) ) ;
#31297=CARTESIAN_POINT ( 'NONE',  ( -6.840914352312096547, 57.56018628210145494, 6.594114490232313663 ) ) ;
#31304=CARTESIAN_POINT ( 'NONE',  ( 9.500000000000005329, 47.88981371789855501, -0.1745138560723090149 ) ) ;
#31308=CARTESIAN_POINT ( 'NONE',  ( 7.228626920338837358, 67.72731371789855359, 10.49813415416005036 ) ) ;
#31311=CARTESIAN_POINT ( 'NONE',  ( 2.660918448318002838, 22.30231371789854933, 12.46528703574811558 ) ) ;
#31326=CARTESIAN_POINT ( 'NONE',  ( -10.83675517735179028, 32.93981371789854506, 11.08355503943118947 ) ) ;
#31328=CARTESIAN_POINT ( 'NONE',  ( -3.796722387233375073, 139.7851862821014493, 8.710071997420127943 ) ) ;
#31329=CARTESIAN_POINT ( 'NONE',  ( -10.69584247140444866, 57.84768628210144925, 6.932735513423972762 ) ) ;
#31333=CARTESIAN_POINT ( 'NONE',  ( 2.908627838312118019, 19.32268628210144001, 15.53471296425195369 ) ) ;
#31339=CARTESIAN_POINT ( 'NONE',  ( -2.660918448318275509, 10.69768628210143646, 12.46528703574805874 ) ) ;
#31341=CARTESIAN_POINT ( 'NONE',  ( 8.843639120294245259, 103.6648137178985678, 3.474262827703527901 ) ) ;
#31347=CARTESIAN_POINT ( 'NONE',  ( 4.622313124798831829, 119.7648137178985763, -11.61527771782809282 ) ) ;
#31362=CARTESIAN_POINT ( 'NONE',  ( -2.311890736173176641, 51.52268628210145351, -12.53471296425194836 ) ) ;
#31369=CARTESIAN_POINT ( 'NONE',  ( -4.944772684328424539, 100.2148137178985650, -11.48171059495408031 ) ) ;
#31377=CARTESIAN_POINT ( 'NONE',  ( 2.908627838312458636, 101.0773137178985479, -15.53471296425188442 ) ) ;
#31381=CARTESIAN_POINT ( 'NONE',  ( -10.69584247140444866, 131.4476862821014436, 6.932735513423972762 ) ) ;
#31382=CARTESIAN_POINT ( 'NONE',  ( -0.1745138560725817967, 65.61018628210146630, 15.50000000000000533 ) ) ;
#31386=CARTESIAN_POINT ( 'NONE',  ( 6.092822981423978490, 61.58518628210146062, -14.25334919248782306 ) ) ;
#31388=CARTESIAN_POINT ( 'NONE',  ( 9.500000000000005329, 26.51018628210144001, 0.1745138560725188748 ) ) ;
#31392=CARTESIAN_POINT ( 'NONE',  ( 11.61527771782819940, 53.53518628210144925, -4.622313124798573369 ) ) ;
#31396=CARTESIAN_POINT ( 'NONE',  ( 6.840914352312096547, 25.36018628210144854, -6.594114490232313663 ) ) ;
#31407=CARTESIAN_POINT ( 'NONE',  ( -11.61527771782819940, 67.33518628210144641, 4.622313124798574258 ) ) ;
#31413=CARTESIAN_POINT ( 'NONE',  ( 15.46528703574811736, 38.40231371789853654, -3.257655550456947768 ) ) ;
#31419=CARTESIAN_POINT ( 'NONE',  ( 6.840914352311949109, 30.63981371789855146, 6.594114490232462877 ) ) ;
#31424=CARTESIAN_POINT ( 'NONE',  ( -2.311890736173448424, 13.67731371789854400, 12.53471296425189330 ) ) ;
#31426=CARTESIAN_POINT ( 'NONE',  ( 8.715434833791931624, 64.46018628210146062, 8.962234695871760692 ) ) ;
#31433=CARTESIAN_POINT ( 'NONE',  ( 5.233372021372432847, 83.14768628210143220, 8.152565276336710909 ) ) ;
#31435=CARTESIAN_POINT ( 'NONE',  ( 10.49813415415989581, 110.1726862821014521, 7.228626920339068285 ) ) ;
#31447=CARTESIAN_POINT ( 'NONE',  ( -7.228626920338836470, 118.3273137178985621, -10.49813415416005213 ) ) ;
#31448=CARTESIAN_POINT ( 'NONE',  ( -12.53471296425194659, 132.0226862821014606, 2.311890736173176641 ) ) ;
#31454=CARTESIAN_POINT ( 'NONE',  ( -8.927990412390371944, 99.92731371789854222, -13.04141134922778988 ) ) ;
#31455=CARTESIAN_POINT ( 'NONE',  ( -2.660918448318275509, 93.49768628210145494, 12.46528703574805874 ) ) ;
#31458=CARTESIAN_POINT ( 'NONE',  ( 12.53471296425194836, 118.2226862821014635, -2.311890736173178418 ) ) ;
#31464=CARTESIAN_POINT ( 'NONE',  ( -6.932735513423968321, 115.3476862821014635, -10.69584247140445221 ) ) ;
#31469=CARTESIAN_POINT ( 'NONE',  ( -3.257655550457281723, 102.6976862821014294, 15.46528703574804986 ) ) ;
#31470=CARTESIAN_POINT ( 'NONE',  ( 4.622313124798573369, 9.835186282101449962, 11.61527771782819940 ) ) ;
#31473=CARTESIAN_POINT ( 'NONE',  ( 0.1745138560725194299, 134.6101862821014947, -9.500000000000005329 ) ) ;
#31478=CARTESIAN_POINT ( 'NONE',  ( 1.715153634034233487, 56.12268628210142651, 9.534712964251941258 ) ) ;
#31486=CARTESIAN_POINT ( 'NONE',  ( -5.529263428287297444, 44.72731371789853938, -7.954856959092311719 ) ) ;
#31491=CARTESIAN_POINT ( 'NONE',  ( -12.53471296425189152, 61.97731371789855359, -2.311890736173453309 ) ) ;
#31494=CARTESIAN_POINT ( 'NONE',  ( 7.228626920338837358, 12.52731371789855785, 10.49813415416005036 ) ) ;
#31498=CARTESIAN_POINT ( 'NONE',  ( -12.46528703574805697, 3.797686282101447652, -2.660918448318280838 ) ) ;
#31502=( NAMED_UNIT ( * ) PLANE_ANGLE_UNIT ( ) SI_UNIT ( $, .RADIAN. ) );
#31509=CARTESIAN_POINT ( 'NONE',  ( 8.927990412390371944, 12.52731371789855963, 13.04141134922778811 ) ) ;
#31511=CARTESIAN_POINT ( 'NONE',  ( 8.962234695871762469, 16.16018628210144570, -8.715434833791931624 ) ) ;
#31513=CARTESIAN_POINT ( 'NONE',  ( -12.50000000000000355, 49.51018628210145067, -0.1745138560725492671 ) ) ;
#31516=CARTESIAN_POINT ( 'NONE',  ( 6.092822981423978490, 15.58518628210145351, -14.25334919248782306 ) ) ;
#31524=CARTESIAN_POINT ( 'NONE',  ( 6.594114490232462877, 101.9398137178985735, -6.840914352311949109 ) ) ;
#31532=CARTESIAN_POINT ( 'NONE',  ( 10.49813415416005213, 111.4273137178985564, -7.228626920338837358 ) ) ;
#31545=CARTESIAN_POINT ( 'NONE',  ( -11.48171059495397373, 50.08518628210144641, -4.944772684328680334 ) ) ;
#31552=CARTESIAN_POINT ( 'NONE',  ( -4.944772684328424539, 109.4148137178985536, -11.48171059495408031 ) ) ;
#31557=CARTESIAN_POINT ( 'NONE',  ( 14.38691631536194393, 85.26481371789857633, 5.770363421894124656 ) ) ;
#31561=CARTESIAN_POINT ( 'NONE',  ( -12.50000000000000355, 95.51018628210144357, -0.1745138560725492671 ) ) ;
#31563=CARTESIAN_POINT ( 'NONE',  ( 8.632099005475504683, 64.74768628210144072, 13.23911966647218996 ) ) ;
#31567=CARTESIAN_POINT ( 'NONE',  ( -13.04141134922759804, 59.57268628210145067, -8.927990412390657937 ) ) ;
#31572=CARTESIAN_POINT ( 'NONE',  ( 12.53471296425194836, 44.62268628210144783, -2.311890736173178418 ) ) ;
#31575=CARTESIAN_POINT ( 'NONE',  ( -2.064181346179269738, 29.09768628210144925, 9.465287035748067623 ) ) ;
#31586=CARTESIAN_POINT ( 'NONE',  ( -2.311890736173176641, 60.72268628210144925, -12.53471296425194659 ) ) ;
#31593=CARTESIAN_POINT ( 'NONE',  ( 8.632099005475788900, 37.25231371789855217, -13.23911966647199812 ) ) ;
#31600=CARTESIAN_POINT ( 'NONE',  ( 1.715153634034445762, 18.27731371789853299, -9.534712964251895073 ) ) ;
#31604=CARTESIAN_POINT ( 'NONE',  ( -6.092822981423666739, 137.0148137178985621, -14.25334919248795096 ) ) ;
#31606=CARTESIAN_POINT ( 'NONE',  ( -11.48171059495397373, 59.28518628210144215, -4.944772684328680334 ) ) ;
#31614=CARTESIAN_POINT ( 'NONE',  ( 3.474262827703335166, 83.43518628210145494, 8.843639120294326972 ) ) ;
#31616=CARTESIAN_POINT ( 'NONE',  ( -10.69584247140444866, 94.64768628210146062, 6.932735513423972762 ) ) ;
#31628=CARTESIAN_POINT ( 'NONE',  ( -10.49813415416004858, 116.0273137178985650, 7.228626920338839135 ) ) ;
#31629=CARTESIAN_POINT ( 'NONE',  ( -0.1745138560725500443, 120.8101862821014691, 12.50000000000000355 ) ) ;
#31636=CARTESIAN_POINT ( 'NONE',  ( -11.08355503943118592, 90.43981371789854506, -10.83675517735179383 ) ) ;
#31638=CARTESIAN_POINT ( 'NONE',  ( -2.311890736173176641, 88.32268628210144357, -12.53471296425194836 ) ) ;
#31641=CARTESIAN_POINT ( 'NONE',  ( 2.064181346179061460, 68.30231371789852801, 9.465287035748106703 ) ) ;
#31645=CARTESIAN_POINT ( 'NONE',  ( 11.61527771782809637, 66.86481371789855643, 4.622313124798827388 ) ) ;
#31648=CARTESIAN_POINT ( 'NONE',  ( -10.49813415415989581, 123.9726862821014493, -7.228626920339068285 ) ) ;
#31653=CARTESIAN_POINT ( 'NONE',  ( 14.25334919248782661, 100.6851862821014834, 6.092822981423971385 ) ) ;
#31654=CARTESIAN_POINT ( 'NONE',  ( -6.932735513423968321, 14.14768628210144641, -10.69584247140445221 ) ) ;
#31657=CARTESIAN_POINT ( 'NONE',  ( 3.474262827703335166, 129.4351862821014549, 8.843639120294326972 ) ) ;
#31661=CARTESIAN_POINT ( 'NONE',  ( -9.534712964251941258, 67.62268628210145494, 1.715153634034234154 ) ) ;
#31669=CARTESIAN_POINT ( 'NONE',  ( 9.500000000000005329, 29.48981371789855288, -0.1745138560723090149 ) ) ;
#31674=CARTESIAN_POINT ( 'NONE',  ( -12.53471296425189152, 43.57731371789855501, -2.311890736173453309 ) ) ;
#31677=CARTESIAN_POINT ( 'NONE',  ( 8.927990412390371944, 141.3273137178985621, 13.04141134922778811 ) ) ;
#31693=CARTESIAN_POINT ( 'NONE',  ( -8.927990412390371944, 26.32731371789854791, -13.04141134922778988 ) ) ;
#31696=CARTESIAN_POINT ( 'NONE',  ( 12.46528703574805874, 8.397686282101442856, 2.660918448318279950 ) ) ;
#31698=CARTESIAN_POINT ( 'NONE',  ( 11.61527771782819940, 53.53518628210144925, -4.622313124798573369 ) ) ;
#31711=CARTESIAN_POINT ( 'NONE',  ( -0.1745138560723084320, 91.58981371789856496, -9.500000000000005329 ) ) ;
#31718=CARTESIAN_POINT ( 'NONE',  ( -2.311890736173447980, 96.47731371789855359, 12.53471296425189330 ) ) ;
#31722=CARTESIAN_POINT ( 'NONE',  ( 12.53471296425189330, 57.37731371789855928, 2.311890736173451977 ) ) ;
#31732=CARTESIAN_POINT ( 'NONE',  ( 10.69584247140445221, 53.24768628210144072, -6.932735513423970097 ) ) ;
#31738=CARTESIAN_POINT ( 'NONE',  ( -12.53471296425189152, 98.77731371789855075, -2.311890736173453753 ) ) ;
#31744=CARTESIAN_POINT ( 'NONE',  ( 13.04141134922778988, 74.62731371789853085, -8.927990412390371944 ) ) ;
#31748=CARTESIAN_POINT ( 'NONE',  ( -8.962234695871760692, 112.7601862821014720, 8.715434833791933400 ) ) ;
#31749=CARTESIAN_POINT ( 'NONE',  ( -14.25334919248782306, 40.88518628210145067, -6.092822981423979378 ) ) ;
#31750=DIRECTION ( 'NONE',  ( 1.045431693899523378E-14, 0.1163425707149433885, -0.9932091452657081376 ) ) ;
#31752=CARTESIAN_POINT ( 'NONE',  ( 15.53471296425195369, 72.22268628210143504, -2.908627838312120684 ) ) ;
#31757=CARTESIAN_POINT ( 'NONE',  ( -8.715434833791929847, 41.46018628210144641, -8.962234695871762469 ) ) ;
#31760=CARTESIAN_POINT ( 'NONE',  ( -6.594114490232462877, 143.3398137178985507, 6.840914352311949109 ) ) ;
#31768=CARTESIAN_POINT ( 'NONE',  ( -11.48171059495397373, 59.28518628210144215, -4.944772684328680334 ) ) ;
#31774=CARTESIAN_POINT ( 'NONE',  ( 11.08355503943118769, 39.83981371789855075, 10.83675517735179028 ) ) ;
#31780=CARTESIAN_POINT ( 'NONE',  ( -5.233372021372612259, 23.45231371789854435, 8.152565276336593669 ) ) ;
#31786=CARTESIAN_POINT ( 'NONE',  ( 8.927990412390371944, 122.9273137178985422, 13.04141134922778811 ) ) ;
#31788=CARTESIAN_POINT ( 'NONE',  ( 6.932735513423970097, 46.34768628210145636, 10.69584247140445044 ) ) ;
#31795=CARTESIAN_POINT ( 'NONE',  ( 3.796722387233379514, 70.78518628210143504, -8.710071997420127943 ) ) ;
#31798=CARTESIAN_POINT ( 'NONE',  ( 8.715434833791931624, 92.06018628210145494, 8.962234695871760692 ) ) ;
#31812=CARTESIAN_POINT ( 'NONE',  ( 2.311890736173452865, 119.4773137178985678, -12.53471296425189152 ) ) ;
#31813=CARTESIAN_POINT ( 'NONE',  ( -8.962234695871760692, 121.9601862821014464, 8.715434833791933400 ) ) ;
#31819=CARTESIAN_POINT ( 'NONE',  ( -8.927990412390371944, 90.72731371789855359, -13.04141134922778988 ) ) ;
#31824=CARTESIAN_POINT ( 'NONE',  ( -3.474262827703527901, 78.36481371789855643, 8.843639120294245259 ) ) ;
#31828=CARTESIAN_POINT ( 'NONE',  ( 0.1745138560722779009, 50.18981371789854506, 12.50000000000000355 ) ) ;
#31830=CARTESIAN_POINT ( 'NONE',  ( -8.962234695871760692, 94.36018628210145209, 8.715434833791933400 ) ) ;
#31836=CARTESIAN_POINT ( 'NONE',  ( -14.25334919248782306, 105.2851862821014777, -6.092822981423979378 ) ) ;
#31838=CARTESIAN_POINT ( 'NONE',  ( 12.50000000000000355, 8.110186282101444988, 0.1745138560725507937 ) ) ;
#31842=CARTESIAN_POINT ( 'NONE',  ( -9.534712964251941258, 132.0226862821014322, 1.715153634034234154 ) ) ;
#31846=CARTESIAN_POINT ( 'NONE',  ( -6.594114490232312775, 59.86018628210145209, -6.840914352312096547 ) ) ;
#31854=CARTESIAN_POINT ( 'NONE',  ( 7.954856959092311719, 37.82731371789854080, -5.529263428287300108 ) ) ;
#31859=CARTESIAN_POINT ( 'NONE',  ( -0.1745138560722763466, 36.38981371789855501, -12.50000000000000355 ) ) ;
#31862=CARTESIAN_POINT ( 'NONE',  ( 8.715434833792128799, 9.939813717898537959, -8.962234695871567070 ) ) ;
#31881=CARTESIAN_POINT ( 'NONE',  ( -15.50000000000000533, 24.88981371789854080, 0.1745138560722471477 ) ) ;
#31883=CARTESIAN_POINT ( 'NONE',  ( -5.529263428287477744, 140.0726862821014151, 7.954856959092191815 ) ) ;
#31884=CARTESIAN_POINT ( 'NONE',  ( 4.622313124798573369, 46.63518628210145067, 11.61527771782819940 ) ) ;
#31896=CARTESIAN_POINT ( 'NONE',  ( -7.954856959092309943, 97.62731371789854506, 5.529263428287300108 ) ) ;
#31904=CARTESIAN_POINT ( 'NONE',  ( -11.61527771782809282, 108.2648137178985621, -4.622313124798832717 ) ) ;
#31908=CARTESIAN_POINT ( 'NONE',  ( -12.53471296425189152, 61.97731371789854649, -2.311890736173453753 ) ) ;
#31916=CARTESIAN_POINT ( 'NONE',  ( 2.660918448318279950, 42.89768628210143930, -12.46528703574805697 ) ) ;
#31922=CARTESIAN_POINT ( 'NONE',  ( -7.228626920338836470, 109.1273137178985735, -10.49813415416005213 ) ) ;
#31927=CARTESIAN_POINT ( 'NONE',  ( 3.257655550456945548, 77.50231371789855928, 15.46528703574811736 ) ) ;
#31931=CARTESIAN_POINT ( 'NONE',  ( -12.46528703574805697, 104.9976862821014691, -2.660918448318280838 ) ) ;
#31932=CARTESIAN_POINT ( 'NONE',  ( -13.23911966647218463, 48.64768628210144641, 8.632099005475506459 ) ) ;
#31935=CARTESIAN_POINT ( 'NONE',  ( 8.632099005475504683, 73.94768628210142936, 13.23911966647218996 ) ) ;
#31941=CARTESIAN_POINT ( 'NONE',  ( -4.622313124798576922, 32.83518628210143930, -11.61527771782819762 ) ) ;
#31944=CARTESIAN_POINT ( 'NONE',  ( 8.843639120294245259, 140.4648137178985507, 3.474262827703527901 ) ) ;
#31956=CARTESIAN_POINT ( 'NONE',  ( 12.46528703574805874, 63.59768628210145636, 2.660918448318279950 ) ) ;
#31964=CARTESIAN_POINT ( 'NONE',  ( -2.908627838312453306, 32.07731371789855501, 15.53471296425188797 ) ) ;
#31972=CARTESIAN_POINT ( 'NONE',  ( 3.796722387233182339, 22.01481371789855501, 8.710071997420207879 ) ) ;
#31978=CARTESIAN_POINT ( 'NONE',  ( 8.927990412390371944, 132.1273137178985735, 13.04141134922778811 ) ) ;
#31980=CARTESIAN_POINT ( 'NONE',  ( 0.1745138560725515708, 51.81018628210144783, -12.50000000000000355 ) ) ;
#31987=CARTESIAN_POINT ( 'NONE',  ( 7.954856959092191815, 64.17268628210143788, 5.529263428287477744 ) ) ;
#31990=CARTESIAN_POINT ( 'NONE',  ( 6.932735513423970097, 92.34768628210144925, 10.69584247140445044 ) ) ;
#32001=CARTESIAN_POINT ( 'NONE',  ( 12.53471296425189330, 112.5773137178985621, 2.311890736173451977 ) ) ;
#32002=CARTESIAN_POINT ( 'NONE',  ( -11.48171059495397373, 123.6851862821014549, -4.944772684328680334 ) ) ;
#32007=CARTESIAN_POINT ( 'NONE',  ( 14.25334919248795451, 93.31481371789855928, -6.092822981423661410 ) ) ;
#32011=CARTESIAN_POINT ( 'NONE',  ( -8.152565276336593669, 80.95231371789854791, -5.233372021372610483 ) ) ;
#32014=CARTESIAN_POINT ( 'NONE',  ( 0.1745138560722779009, 40.98981371789854933, 12.50000000000000355 ) ) ;
#32016=CARTESIAN_POINT ( 'NONE',  ( -0.1745138560725500443, 93.21018628210146062, 12.50000000000000355 ) ) ;
#32021=CARTESIAN_POINT ( 'NONE',  ( -2.908627838312119351, 106.7226862821014635, -15.53471296425195369 ) ) ;
#32022=CARTESIAN_POINT ( 'NONE',  ( -4.622313124798576922, 23.63518628210144357, -11.61527771782819762 ) ) ;
#32025=CARTESIAN_POINT ( 'NONE',  ( -3.474262827703337830, 124.8351862821014748, -8.843639120294326972 ) ) ;
#32032=CARTESIAN_POINT ( 'NONE',  ( -9.534712964251941258, 58.42268628210145209, 1.715153634034234154 ) ) ;
#32039=CARTESIAN_POINT ( 'NONE',  ( 7.954856959092311719, 47.02731371789855075, -5.529263428287300108 ) ) ;
#32044=CARTESIAN_POINT ( 'NONE',  ( 12.46528703574811558, 38.40231371789855075, -2.660918448318005947 ) ) ;
#32047=CARTESIAN_POINT ( 'NONE',  ( -4.944772684328424539, 17.41481371789854649, -11.48171059495408031 ) ) ;
#32067=CARTESIAN_POINT ( 'NONE',  ( 0.1745138560722461762, 22.58981371789854364, 15.50000000000000533 ) ) ;
#32069=CARTESIAN_POINT ( 'NONE',  ( -8.152565276336710909, 131.4476862821014436, 5.233372021372435512 ) ) ;
#32070=CARTESIAN_POINT ( 'NONE',  ( -2.311890736173176641, 42.32268628210145067, -12.53471296425194836 ) ) ;
#32075=CARTESIAN_POINT ( 'NONE',  ( 9.500000000000005329, 17.31018628210144428, 0.1745138560725188748 ) ) ;
#32083=CARTESIAN_POINT ( 'NONE',  ( 9.465287035748106703, 102.8023137178985422, -2.064181346179063237 ) ) ;
#32088=CARTESIAN_POINT ( 'NONE',  ( 10.49813415416005213, 102.2273137178985536, -7.228626920338837358 ) ) ;
#32092=CARTESIAN_POINT ( 'NONE',  ( -8.715434833792127023, 69.73981371789855643, 8.962234695871568846 ) ) ;
#32101=CARTESIAN_POINT ( 'NONE',  ( -4.622313124798576922, 42.03518628210144215, -11.61527771782819762 ) ) ;
#32105=CARTESIAN_POINT ( 'NONE',  ( -10.69584247140429412, 108.5523137178985564, -6.932735513424201024 ) ) ;
#32110=CARTESIAN_POINT ( 'NONE',  ( 5.770363421894130873, 82.96481371789856496, -14.38691631536193860 ) ) ;
#32114=CARTESIAN_POINT ( 'NONE',  ( -2.660918448318275509, 102.6976862821014720, 12.46528703574805874 ) ) ;
#32115=CARTESIAN_POINT ( 'NONE',  ( -6.092822981423970496, 47.78518628210144215, 14.25334919248782661 ) ) ;
#32116=CARTESIAN_POINT ( 'NONE',  ( -12.50000000000000355, 144.4898137178985564, 0.1745138560722786503 ) ) ;
#32119=CARTESIAN_POINT ( 'NONE',  ( 0.1745138560725837118, 70.21018628210144641, -15.50000000000000533 ) ) ;
#32126=CARTESIAN_POINT ( 'NONE',  ( 10.49813415415989581, 36.57268628210145067, 7.228626920339068285 ) ) ;
#32128=CARTESIAN_POINT ( 'NONE',  ( 9.500000000000005329, 8.110186282101443211, 0.1745138560725188748 ) ) ;
#32138=CARTESIAN_POINT ( 'NONE',  ( 4.944772684328679446, 61.58518628210145351, -11.48171059495397373 ) ) ;
#32145=CARTESIAN_POINT ( 'NONE',  ( 2.908627838312458636, 27.47731371789854649, -15.53471296425188442 ) ) ;
#32153=CARTESIAN_POINT ( 'NONE',  ( -3.796722387233185003, 17.41481371789854649, -8.710071997420207879 ) ) ;
#32159=CARTESIAN_POINT ( 'NONE',  ( -15.46528703574811736, 125.8023137178985706, 3.257655550456946436 ) ) ;
#32164=CARTESIAN_POINT ( 'NONE',  ( 10.69584247140445221, 53.24768628210144072, -6.932735513423970097 ) ) ;
#32173=CARTESIAN_POINT ( 'NONE',  ( 0.1745138560725194299, 61.01018628210145067, -9.500000000000005329 ) ) ;
#32177=CARTESIAN_POINT ( 'NONE',  ( 2.660918448318279950, 98.09768628210146346, -12.46528703574805697 ) ) ;
#32191=CARTESIAN_POINT ( 'NONE',  ( 7.228626920338837358, 104.5273137178985650, 10.49813415416005036 ) ) ;
#32192=CARTESIAN_POINT ( 'NONE',  ( -2.660918448318275509, 130.2976862821014379, 12.46528703574805874 ) ) ;
#32197=CARTESIAN_POINT ( 'NONE',  ( -8.632099005475794229, 87.85231371789855359, 13.23911966647199812 ) ) ;
#32200=CARTESIAN_POINT ( 'NONE',  ( -9.500000000000005329, 104.7101862821014606, -0.1745138560725176813 ) ) ;
#32203=CARTESIAN_POINT ( 'NONE',  ( 0.1745138560723095977, 68.58981371789855075, 9.500000000000005329 ) ) ;
#32206=CARTESIAN_POINT ( 'NONE',  ( 4.622313124798831829, 55.36481371789855643, -11.61527771782809282 ) ) ;
#32208=CARTESIAN_POINT ( 'NONE',  ( 7.228626920339068285, 98.67268628210145209, -10.49813415415989581 ) ) ;
#32211=CARTESIAN_POINT ( 'NONE',  ( 8.715434833791931624, 138.0601862821014549, 8.962234695871760692 ) ) ;
#32213=CARTESIAN_POINT ( 'NONE',  ( 15.50000000000000533, 90.91018628210146346, 0.1745138560725827404 ) ) ;
#32217=CARTESIAN_POINT ( 'NONE',  ( 5.529263428287477744, 107.8726862821014549, -7.954856959092191815 ) ) ;
#32219=CARTESIAN_POINT ( 'NONE',  ( 15.50000000000000533, 8.110186282101443211, 0.1745138560725827404 ) ) ;
#32230=CARTESIAN_POINT ( 'NONE',  ( -9.500000000000005329, 34.08981371789853654, 0.1745138560723101806 ) ) ;
#32234=CARTESIAN_POINT ( 'NONE',  ( -11.48171059495408208, 51.91481371789855359, 4.944772684328421875 ) ) ;
#32236=CARTESIAN_POINT ( 'NONE',  ( -8.962234695871565293, 16.83981371789855430, -8.715434833792128799 ) ) ;
#32251=CARTESIAN_POINT ( 'NONE',  ( -8.927990412390661490, 140.0726862821014151, 13.04141134922759804 ) ) ;
#32254=CARTESIAN_POINT ( 'NONE',  ( 2.064181346179272847, 125.6976862821014578, -9.465287035748065847 ) ) ;
#32255=CARTESIAN_POINT ( 'NONE',  ( 2.311890736173175753, 28.52268628210144641, 12.53471296425194836 ) ) ;
#32259=CARTESIAN_POINT ( 'NONE',  ( 6.092822981423978490, 125.9851862821014521, -14.25334919248782306 ) ) ;
#32261=CARTESIAN_POINT ( 'NONE',  ( 8.152565276336714462, 16.44768628210144001, -5.233372021372432847 ) ) ;
#32268=CARTESIAN_POINT ( 'NONE',  ( 8.843639120294245259, 85.26481371789857633, 3.474262827703527901 ) ) ;
#32273=CARTESIAN_POINT ( 'NONE',  ( -10.49813415416004858, 97.62731371789857349, 7.228626920338840023 ) ) ;
#32277=CARTESIAN_POINT ( 'NONE',  ( 6.932735513424201024, 64.85231371789855359, -10.69584247140429412 ) ) ;
#32285=CARTESIAN_POINT ( 'NONE',  ( -7.228626920339069173, 38.87268628210144072, 10.49813415415989581 ) ) ;
#32294=CARTESIAN_POINT ( 'NONE',  ( -11.48171059495408208, 79.51481371789856212, 4.944772684328421875 ) ) ;
#32300=CARTESIAN_POINT ( 'NONE',  ( -11.08355503943118592, 81.23981371789855643, -10.83675517735179383 ) ) ;
#32303=CARTESIAN_POINT ( 'NONE',  ( 11.48171059495397728, 82.28518628210146346, 4.944772684328674117 ) ) ;
#32304=CARTESIAN_POINT ( 'NONE',  ( 10.83675517735155225, 46.06018628210144072, 11.08355503943142573 ) ) ;
#32308=CARTESIAN_POINT ( 'NONE',  ( 15.53471296425195369, 53.82268628210144357, -2.908627838312120684 ) ) ;
#32314=CARTESIAN_POINT ( 'NONE',  ( 4.944772684328679446, 33.98518628210143788, -11.48171059495397373 ) ) ;
#32316=CARTESIAN_POINT ( 'NONE',  ( -9.500000000000005329, 144.4898137178985280, 0.1745138560723101806 ) ) ;
#32328=CARTESIAN_POINT ( 'NONE',  ( -6.932735513423968321, 50.94768628210144357, -10.69584247140445221 ) ) ;
#32335=CARTESIAN_POINT ( 'NONE',  ( 10.69584247140445221, 99.24768628210146915, -6.932735513423970097 ) ) ;
#32336=CARTESIAN_POINT ( 'NONE',  ( 14.25334919248795451, 28.91481371789854649, -6.092822981423661410 ) ) ;
#32342=CARTESIAN_POINT ( 'NONE',  ( 5.529263428287300108, 12.52731371789855963, 7.954856959092309943 ) ) ;
#32349=CARTESIAN_POINT ( 'NONE',  ( -10.83675517735179028, 134.1398137178985621, 11.08355503943118947 ) ) ;
#32353=CARTESIAN_POINT ( 'NONE',  ( -6.932735513423968321, 41.74768628210144783, -10.69584247140445221 ) ) ;
#32358=( LENGTH_UNIT ( ) NAMED_UNIT ( * ) SI_UNIT ( .MILLI., .METRE. ) );
#32360=CARTESIAN_POINT ( 'NONE',  ( -9.465287035748065847, 58.99768628210144783, -2.064181346179273735 ) ) ;
#32363=CARTESIAN_POINT ( 'NONE',  ( -12.53471296425194836, 95.22268628210146346, 2.311890736173176641 ) ) ;
#32371=PRODUCT_DEFINITION_CONTEXT ( 'detailed design', #25034, 'design' ) ;
#32377=CARTESIAN_POINT ( 'NONE',  ( -2.660918448318004614, 100.5023137178985593, -12.46528703574811558 ) ) ;
#32378=CARTESIAN_POINT ( 'NONE',  ( -4.622313124798576922, 97.23518628210145209, -11.61527771782819762 ) ) ;
#32382=CARTESIAN_POINT ( 'NONE',  ( -15.46528703574811736, 79.80231371789852801, 3.257655550456946436 ) ) ;
#32385=CARTESIAN_POINT ( 'NONE',  ( -5.233372021372430183, 106.1476862821014322, -8.152565276336710909 ) ) ;
#32388=CARTESIAN_POINT ( 'NONE',  ( 6.594114490232462877, 74.33981371789855075, -6.840914352311949109 ) ) ;
#32391=CARTESIAN_POINT ( 'NONE',  ( -12.53471296425189152, 52.77731371789855075, -2.311890736173453753 ) ) ;
#32393=CARTESIAN_POINT ( 'NONE',  ( -7.228626920339069173, 103.2726862821014606, 10.49813415415989581 ) ) ;
#32399=CARTESIAN_POINT ( 'NONE',  ( 14.38691631536207538, 81.13518628210145778, -5.770363421893813793 ) ) ;
#32401=CARTESIAN_POINT ( 'NONE',  ( 2.660918448318279950, 6.097686282101443922, -12.46528703574805874 ) ) ;
#32404=CARTESIAN_POINT ( 'NONE',  ( -5.529263428287477744, 121.6726862821014521, 7.954856959092191815 ) ) ;
#32406=CARTESIAN_POINT ( 'NONE',  ( -14.38691631536207183, 12.13518628210144712, 5.770363421893814682 ) ) ;
#32417=CARTESIAN_POINT ( 'NONE',  ( 9.500000000000005329, 11.08981371789854897, -0.1745138560723090149 ) ) ;
#32421=CARTESIAN_POINT ( 'NONE',  ( -4.622313124798826500, 50.76481371789855501, 11.61527771782809637 ) ) ;
#32423=CARTESIAN_POINT ( 'NONE',  ( 15.53471296425188797, 130.9773137178985394, 2.908627838312457747 ) ) ;
#32441=CARTESIAN_POINT ( 'NONE',  ( 15.46528703574811736, 10.80231371789855466, -3.257655550456947768 ) ) ;
#32443=CARTESIAN_POINT ( 'NONE',  ( 2.064181346179272847, 134.8976862821014606, -9.465287035748065847 ) ) ;
#32445=CARTESIAN_POINT ( 'NONE',  ( 0.1745138560725515708, 24.21018628210144641, -12.50000000000000355 ) ) ;
#32449=CARTESIAN_POINT ( 'NONE',  ( -3.257655550457281723, 130.2976862821014379, 15.46528703574804986 ) ) ;
#32451=CARTESIAN_POINT ( 'NONE',  ( -6.594114490232312775, 4.660186282101435928, -6.840914352312096547 ) ) ;
#32458=CARTESIAN_POINT ( 'NONE',  ( 6.594114490232462877, 83.53981371789856780, -6.840914352311949109 ) ) ;
#32462=CARTESIAN_POINT ( 'NONE',  ( -10.69584247140429412, 90.15231371789853654, -6.932735513424201024 ) ) ;
#32466=CARTESIAN_POINT ( 'NONE',  ( 0.1745138560722779009, 59.38981371789856212, 12.50000000000000355 ) ) ;
#32472=CARTESIAN_POINT ( 'NONE',  ( 0.1745138560725515708, 42.61018628210144499, -12.50000000000000355 ) ) ;
#32477=CARTESIAN_POINT ( 'NONE',  ( -2.311890736173448424, 87.27731371789856496, 12.53471296425189330 ) ) ;
#32482=CARTESIAN_POINT ( 'NONE',  ( 10.83675517735179206, 65.13981371789854791, -11.08355503943118769 ) ) ;
#32485=CARTESIAN_POINT ( 'NONE',  ( 12.50000000000000355, 90.91018628210146346, 0.1745138560725507937 ) ) ;
#32486=CARTESIAN_POINT ( 'NONE',  ( -13.23911966647218463, 39.44768628210144357, 8.632099005475506459 ) ) ;
#32489=CARTESIAN_POINT ( 'NONE',  ( 14.25334919248782661, 54.68518628210145494, 6.092822981423971385 ) ) ;
#32497=CARTESIAN_POINT ( 'NONE',  ( 2.660918448318279950, 24.49768628210144783, -12.46528703574805697 ) ) ;
#32499=CARTESIAN_POINT ( 'NONE',  ( 3.796722387233379514, 15.58518628210145351, -8.710071997420127943 ) ) ;
#32510=CARTESIAN_POINT ( 'NONE',  ( 11.61527771782819940, 53.53518628210144925, -4.622313124798573369 ) ) ;
#32518=CARTESIAN_POINT ( 'NONE',  ( 4.944772684328679446, 89.18518628210145494, -11.48171059495397373 ) ) ;
#32519=CARTESIAN_POINT ( 'NONE',  ( -14.25334919248795096, 24.31481371789855217, 6.092822981423662299 ) ) ;
#32527=CARTESIAN_POINT ( 'NONE',  ( -9.534712964251895073, 6.777313717898553413, -1.715153634034446428 ) ) ;
#32535=CARTESIAN_POINT ( 'NONE',  ( -6.092822981423666739, 118.6148137178985706, -14.25334919248795096 ) ) ;
#32538=CARTESIAN_POINT ( 'NONE',  ( 8.962234695871762469, 43.76018628210144357, -8.715434833791931624 ) ) ;
#32541=CARTESIAN_POINT ( 'NONE',  ( -13.23911966647218463, 94.64768628210147483, 8.632099005475506459 ) ) ;
#32544=CARTESIAN_POINT ( 'NONE',  ( 9.465287035748067623, 63.59768628210142793, 2.064181346179272847 ) ) ;
#32547=CARTESIAN_POINT ( 'NONE',  ( -8.715434833791929847, 78.26018628210144357, -8.962234695871762469 ) ) ;
#32561=CARTESIAN_POINT ( 'NONE',  ( -4.944772684328424539, 109.4148137178985536, -11.48171059495408031 ) ) ;
#32562=CARTESIAN_POINT ( 'NONE',  ( -4.944772684328673229, 102.9851862821014663, 11.48171059495397728 ) ) ;
#32568=CARTESIAN_POINT ( 'NONE',  ( 11.08355503943118769, 67.43981371789855928, 10.83675517735179028 ) ) ;
#32571=CARTESIAN_POINT ( 'NONE',  ( 5.233372021372432847, 101.5476862821014663, 8.152565276336710909 ) ) ;
#32574=CARTESIAN_POINT ( 'NONE',  ( 9.500000000000005329, 57.08981371789855075, -0.1745138560723090149 ) ) ;
#32576=CARTESIAN_POINT ( 'NONE',  ( 5.529263428287300108, 104.5273137178985650, 7.954856959092309943 ) ) ;
#32578=CARTESIAN_POINT ( 'NONE',  ( 4.944772684328420986, 49.61481371789855643, 11.48171059495408208 ) ) ;
#32580=CARTESIAN_POINT ( 'NONE',  ( 2.660918448318279950, 98.09768628210146346, -12.46528703574805697 ) ) ;
#32584=CARTESIAN_POINT ( 'NONE',  ( -10.49813415415989581, 133.1726862821014663, -7.228626920339068285 ) ) ;
#32587=CARTESIAN_POINT ( 'NONE',  ( -15.50000000000000533, 86.31018628210145494, -0.1745138560725808530 ) ) ;
#32592=CARTESIAN_POINT ( 'NONE',  ( -8.843639120294326972, 122.5351862821014493, 3.474262827703335166 ) ) ;
#32594=CARTESIAN_POINT ( 'NONE',  ( -10.83675517735155047, 4.660186282101435928, -11.08355503943142750 ) ) ;
#32606=CARTESIAN_POINT ( 'NONE',  ( -8.710071997420207879, 24.31481371789855217, 3.796722387233182339 ) ) ;
#32612=CARTESIAN_POINT ( 'NONE',  ( 8.715434833792128799, 28.33981371789855075, -8.962234695871567070 ) ) ;
#32614=CARTESIAN_POINT ( 'NONE',  ( -15.46528703574811736, 135.0023137178985166, 3.257655550456946436 ) ) ;
#32632=CARTESIAN_POINT ( 'NONE',  ( 14.38691631536194393, 11.66481371789854293, 5.770363421894124656 ) ) ;
#32634=CARTESIAN_POINT ( 'NONE',  ( 0.1745138560725194299, 125.4101862821014635, -9.500000000000005329 ) ) ;
#32636=CARTESIAN_POINT ( 'NONE',  ( 11.61527771782819940, 35.13518628210143646, -4.622313124798573369 ) ) ;
#32640=CARTESIAN_POINT ( 'NONE',  ( -14.25334919248782306, 123.6851862821014549, -6.092822981423979378 ) ) ;
#32642=CARTESIAN_POINT ( 'NONE',  ( 6.840914352311949109, 141.0398137178985678, 6.594114490232462877 ) ) ;
#32646=EDGE_CURVE ( 'NONE', #21615, #15372, #12942, .T. ) ;
#32649=CARTESIAN_POINT ( 'NONE',  ( 8.152565276336593669, 67.15231371789852233, 5.233372021372610483 ) ) ;
#32653=CARTESIAN_POINT ( 'NONE',  ( 11.48171059495408208, 84.11481371789855643, -4.944772684328420986 ) ) ;
#32655=CARTESIAN_POINT ( 'NONE',  ( -13.16328360146172116, 143.0000000000000284, 4.685063460632339805 ) ) ;
#32657=CARTESIAN_POINT ( 'NONE',  ( 4.944772684328420986, 49.61481371789855643, 11.48171059495408208 ) ) ;
#32663=CARTESIAN_POINT ( 'NONE',  ( -10.69584247140444866, 48.64768628210144641, 6.932735513423972762 ) ) ;
#32668=CARTESIAN_POINT ( 'NONE',  ( -6.932735513424201912, 87.85231371789855359, 10.69584247140429412 ) ) ;
#32673=CARTESIAN_POINT ( 'NONE',  ( 8.927990412390371944, 58.52731371789855785, 13.04141134922778811 ) ) ;
#32677=CARTESIAN_POINT ( 'NONE',  ( 10.49813415415989581, 91.77268628210144641, 7.228626920339068285 ) ) ;
#32678=CARTESIAN_POINT ( 'NONE',  ( 15.53471296425195369, 35.42268628210144499, -2.908627838312120684 ) ) ;
#32681=CARTESIAN_POINT ( 'NONE',  ( 0.1745138560725837118, 51.81018628210144783, -15.50000000000000533 ) ) ;
#32687=CARTESIAN_POINT ( 'NONE',  ( -12.46528703574805697, 12.99768628210143362, -2.660918448318280838 ) ) ;
#32689=CARTESIAN_POINT ( 'NONE',  ( 3.474262827703532341, 128.9648137178985792, -8.843639120294245259 ) ) ;
#32701=CARTESIAN_POINT ( 'NONE',  ( -12.53471296425194659, 58.42268628210145209, 2.311890736173176641 ) ) ;
#32710=CARTESIAN_POINT ( 'NONE',  ( -4.944772684328673229, 93.78518628210144925, 11.48171059495397728 ) ) ;
#32711=CARTESIAN_POINT ( 'NONE',  ( -6.092822981423666739, 26.61481371789854933, -14.25334919248795096 ) ) ;
#32717=CARTESIAN_POINT ( 'NONE',  ( -12.46528703574811558, 135.0023137178985735, 2.660918448318003726 ) ) ;
#32725=CARTESIAN_POINT ( 'NONE',  ( -11.08355503943118592, 108.8398137178985507, -10.83675517735179383 ) ) ;
#32728=CARTESIAN_POINT ( 'NONE',  ( -2.311890736173176641, 23.92268628210143788, -12.53471296425194836 ) ) ;
#32732=CARTESIAN_POINT ( 'NONE',  ( 13.23911966647218996, 99.24768628210145494, -8.632099005475504683 ) ) ;
#32736=CARTESIAN_POINT ( 'NONE',  ( 3.474262827703335166, 65.03518628210144925, 8.843639120294326972 ) ) ;
#32740=CARTESIAN_POINT ( 'NONE',  ( 7.228626920339068285, 80.27268628210146062, -10.49813415415989581 ) ) ;
#32743=CARTESIAN_POINT ( 'NONE',  ( 3.474262827703335166, 46.63518628210144357, 8.843639120294326972 ) ) ;
#32752=CARTESIAN_POINT ( 'NONE',  ( -4.944772684328424539, 100.2148137178985650, -11.48171059495408031 ) ) ;
#32753=CARTESIAN_POINT ( 'NONE',  ( -8.962234695871760692, 103.5601862821014549, 8.715434833791933400 ) ) ;
#32759=CARTESIAN_POINT ( 'NONE',  ( 15.50000000000000533, 84.68981371789855928, -0.1745138560722452326 ) ) ;
#32763=CARTESIAN_POINT ( 'NONE',  ( -8.152565276336710909, 103.8476862821014493, 5.233372021372435512 ) ) ;
#32765=CARTESIAN_POINT ( 'NONE',  ( -8.152565276336593669, 62.55231371789854222, -5.233372021372610483 ) ) ;
#32768=CARTESIAN_POINT ( 'NONE',  ( -2.064181346179062349, 118.9023137178985650, -9.465287035748106703 ) ) ;
#32770=CARTESIAN_POINT ( 'NONE',  ( 8.715434833792128799, 28.33981371789855075, -8.962234695871567070 ) ) ;
#32772=CARTESIAN_POINT ( 'NONE',  ( -12.46528703574805697, 86.59768628210144925, -2.660918448318280838 ) ) ;
#32776=CARTESIAN_POINT ( 'NONE',  ( 10.83675517735155225, 82.86018628210146630, 11.08355503943142573 ) ) ;
#32781=CARTESIAN_POINT ( 'NONE',  ( 8.843639120294328748, 117.9351862821014407, -3.474262827703334722 ) ) ;
#32783=CARTESIAN_POINT ( 'NONE',  ( 10.69584247140445221, 126.8476862821014635, -6.932735513423970097 ) ) ;
#32795=CARTESIAN_POINT ( 'NONE',  ( 9.534712964251900402, 20.57731371789854435, 1.715153634034445540 ) ) ;
#32800=CARTESIAN_POINT ( 'NONE',  ( -0.1745138560722763466, 17.98981371789853867, -12.50000000000000355 ) ) ;
#32802=CARTESIAN_POINT ( 'NONE',  ( 13.23911966647199812, 131.5523137178985564, 8.632099005475788900 ) ) ;
#32808=CARTESIAN_POINT ( 'NONE',  ( 7.228626920339068285, 135.4726862821014493, -10.49813415415989581 ) ) ;
#32814=CARTESIAN_POINT ( 'NONE',  ( 10.69584247140445221, 136.0476862821014379, -6.932735513423970097 ) ) ;
#32818=CARTESIAN_POINT ( 'NONE',  ( -15.50000000000000533, 132.3101862821014549, -0.1745138560725808530 ) ) ;
#32820=CARTESIAN_POINT ( 'NONE',  ( -0.1745138560725182642, 120.8101862821014691, 9.500000000000005329 ) ) ;
#32822=CARTESIAN_POINT ( 'NONE',  ( 11.48171059495397728, 36.28518628210144925, 4.944772684328674117 ) ) ;
#32827=CARTESIAN_POINT ( 'NONE',  ( 8.632099005475504683, 119.9476862821014294, 13.23911966647218996 ) ) ;
#32829=CARTESIAN_POINT ( 'NONE',  ( -2.064181346179062349, 137.3023137178985564, -9.465287035748106703 ) ) ;
#32836=CARTESIAN_POINT ( 'NONE',  ( 5.529263428287300108, 76.92731371789854222, 7.954856959092309943 ) ) ;
#32840=CARTESIAN_POINT ( 'NONE',  ( -11.48171059495408208, 88.71481371789855075, 4.944772684328421875 ) ) ;
#32844=CARTESIAN_POINT ( 'NONE',  ( 12.53471296425189330, 38.97731371789855359, 2.311890736173451977 ) ) ;
#32848=CARTESIAN_POINT ( 'NONE',  ( -2.660918448318275509, 19.89768628210143575, 12.46528703574805874 ) ) ;
#32854=CARTESIAN_POINT ( 'NONE',  ( -12.46528703574811558, 89.00231371789855928, 2.660918448318003726 ) ) ;
#32863=CARTESIAN_POINT ( 'NONE',  ( -15.53471296425188442, 52.77731371789855785, -2.908627838312459080 ) ) ;
#32866=CARTESIAN_POINT ( 'NONE',  ( -10.69584247140444866, 94.64768628210146062, 6.932735513423972762 ) ) ;
#32867=CARTESIAN_POINT ( 'NONE',  ( -15.46528703574804986, 31.39768628210144286, -3.257655550457287497 ) ) ;
#32872=CARTESIAN_POINT ( 'NONE',  ( 3.257655550457285720, 42.89768628210143220, -15.46528703574804986 ) ) ;
#32878=CARTESIAN_POINT ( 'NONE',  ( 2.311890736173175753, 19.32268628210144712, 12.53471296425194836 ) ) ;
#32880=CARTESIAN_POINT ( 'NONE',  ( 7.954856959092311719, 139.0273137178985507, -5.529263428287300108 ) ) ;
#32885=CARTESIAN_POINT ( 'NONE',  ( 11.61527771782809637, 131.2648137178985621, 4.622313124798827388 ) ) ;
#32890=CARTESIAN_POINT ( 'NONE',  ( -0.1745138560725500443, 56.41018628210145636, 12.50000000000000355 ) ) ;
#32898=CARTESIAN_POINT ( 'NONE',  ( -2.660918448318275509, 75.09768628210143504, 12.46528703574805874 ) ) ;
#32899=CARTESIAN_POINT ( 'NONE',  ( 8.632099005475788900, 18.85231371789855359, -13.23911966647199812 ) ) ;
#32905=CARTESIAN_POINT ( 'NONE',  ( -4.944772684328424539, 137.0148137178985621, -11.48171059495408031 ) ) ;
#32911=CARTESIAN_POINT ( 'NONE',  ( 0.1745138560722461762, 114.5898137178985650, 15.50000000000000533 ) ) ;
#32914=CARTESIAN_POINT ( 'NONE',  ( -11.61527771782819940, 30.53518628210144570, 4.622313124798574258 ) ) ;
#32919=CARTESIAN_POINT ( 'NONE',  ( 6.092822981423978490, 107.5851862821014748, -14.25334919248782306 ) ) ;
#32920=CARTESIAN_POINT ( 'NONE',  ( -12.46528703574811558, 43.00231371789854506, 2.660918448318003726 ) ) ;
#32923=CARTESIAN_POINT ( 'NONE',  ( 7.954856959092191815, 45.77268628210144641, 5.529263428287477744 ) ) ;
#32928=CARTESIAN_POINT ( 'NONE',  ( -7.228626920339069173, 75.67268628210146630, 10.49813415415989581 ) ) ;
#32931=CARTESIAN_POINT ( 'NONE',  ( -3.474262827703337830, 51.23518628210143788, -8.843639120294326972 ) ) ;
#32939=CARTESIAN_POINT ( 'NONE',  ( 8.962234695871567070, 95.03981371789856780, 8.715434833792127023 ) ) ;
#32940=CARTESIAN_POINT ( 'NONE',  ( 8.715434833791931624, 101.2601862821014578, 8.962234695871760692 ) ) ;
#32945=CARTESIAN_POINT ( 'NONE',  ( 3.257655550456945548, 77.50231371789855928, 15.46528703574811736 ) ) ;
#32948=CARTESIAN_POINT ( 'NONE',  ( -8.710071997420127943, 96.08518628210146062, -3.796722387233380402 ) ) ;
#32952=CARTESIAN_POINT ( 'NONE',  ( 9.500000000000005329, 66.28981371789855359, -0.1745138560723090149 ) ) ;
#32955=CARTESIAN_POINT ( 'NONE',  ( -9.465287035748106703, 116.6023137178985394, 2.064181346179061460 ) ) ;
#32957=CARTESIAN_POINT ( 'NONE',  ( 7.228626920338837358, 21.72731371789854649, 10.49813415416005036 ) ) ;
#32960=CARTESIAN_POINT ( 'NONE',  ( 4.622313124798573369, 83.43518628210145494, 11.61527771782819940 ) ) ;
#32968=CARTESIAN_POINT ( 'NONE',  ( 5.529263428287477744, 98.67268628210146630, -7.954856959092191815 ) ) ;
#32970=CARTESIAN_POINT ( 'NONE',  ( -11.48171059495397373, 132.8851862821014720, -4.944772684328680334 ) ) ;
#32983=CARTESIAN_POINT ( 'NONE',  ( -5.233372021372612259, 14.25231371789853618, 8.152565276336593669 ) ) ;
#32988=CARTESIAN_POINT ( 'NONE',  ( -11.48171059495408208, 24.31481371789855217, 4.944772684328421875 ) ) ;
#32990=CARTESIAN_POINT ( 'NONE',  ( -2.908627838312453306, 133.2773137178985507, 15.53471296425188797 ) ) ;
#32998=CARTESIAN_POINT ( 'NONE',  ( -11.48171059495397373, 132.8851862821014720, -4.944772684328680334 ) ) ;
#33011=CARTESIAN_POINT ( 'NONE',  ( -11.08355503943118592, 7.639813717898540801, -10.83675517735179383 ) ) ;
#33013=CARTESIAN_POINT ( 'NONE',  ( 9.534712964251941258, 109.0226862821014606, -1.715153634034235708 ) ) ;
#33015=CARTESIAN_POINT ( 'NONE',  ( -2.660918448318275509, 38.29768628210145920, 12.46528703574805874 ) ) ;
#33019=CARTESIAN_POINT ( 'NONE',  ( 15.53471296425195369, 118.2226862821014493, -2.908627838312120684 ) ) ;
#33022=CARTESIAN_POINT ( 'NONE',  ( -2.064181346179269738, 10.69768628210143646, 9.465287035748067623 ) ) ;
#33029=CARTESIAN_POINT ( 'NONE',  ( -6.840914352311947333, 81.23981371789855643, -6.594114490232462877 ) ) ;
#33033=CARTESIAN_POINT ( 'NONE',  ( -10.69584247140429412, 71.75231371789855928, -6.932735513424201024 ) ) ;
#33038=CARTESIAN_POINT ( 'NONE',  ( -12.53471296425189152, 52.77731371789855075, -2.311890736173453753 ) ) ;
#33041=ORIENTED_EDGE ( 'NONE', *, *, #23582, .T. ) ;
#33044=CARTESIAN_POINT ( 'NONE',  ( -2.311890736173176641, 14.72268628210143859, -12.53471296425194836 ) ) ;
#33050=CARTESIAN_POINT ( 'NONE',  ( -8.715434833792127023, 78.93981371789855928, 8.962234695871568846 ) ) ;
#33055=CARTESIAN_POINT ( 'NONE',  ( -11.08355503943118592, 53.63981371789855501, -10.83675517735179383 ) ) ;
#33059=CARTESIAN_POINT ( 'NONE',  ( 12.46528703574805874, 81.99768628210146915, 2.660918448318279950 ) ) ;
#33060=CARTESIAN_POINT ( 'NONE',  ( -0.1745138560725817967, 19.61018628210144144, 15.50000000000000533 ) ) ;
#33065=CARTESIAN_POINT ( 'NONE',  ( -14.25334919248782306, 40.88518628210145067, -6.092822981423979378 ) ) ;
#33072=CARTESIAN_POINT ( 'NONE',  ( -4.944772684328673229, 29.38518628210144712, 11.48171059495397728 ) ) ;
#33074=CARTESIAN_POINT ( 'NONE',  ( 2.064181346179061460, 132.7023137178985337, 9.465287035748106703 ) ) ;
#33079=CARTESIAN_POINT ( 'NONE',  ( 2.311890736173452421, 137.8773137178985735, -12.53471296425189152 ) ) ;
#33085=CARTESIAN_POINT ( 'NONE',  ( -2.311890736173176641, 51.52268628210145351, -12.53471296425194659 ) ) ;
#33092=CARTESIAN_POINT ( 'NONE',  ( 8.962234695871762469, 71.36018628210145209, -8.715434833791931624 ) ) ;
#33093=CARTESIAN_POINT ( 'NONE',  ( -0.1745138560725817967, 139.2101862821014890, 15.50000000000000533 ) ) ;
#33100=CARTESIAN_POINT ( 'NONE',  ( -8.715434833792127023, 134.1398137178985621, 8.962234695871568846 ) ) ;
#33105=CARTESIAN_POINT ( 'NONE',  ( 8.927990412390371944, 113.7273137178985678, 13.04141134922778811 ) ) ;
#33108=CARTESIAN_POINT ( 'NONE',  ( 12.53471296425194836, 26.22268628210144925, -2.311890736173178418 ) ) ;
#33112=CARTESIAN_POINT ( 'NONE',  ( 2.908627838312118019, 102.1226862821014549, 15.53471296425195369 ) ) ;
#33115=CARTESIAN_POINT ( 'NONE',  ( 9.534712964251941258, 35.42268628210144499, -1.715153634034235708 ) ) ;
#33120=CARTESIAN_POINT ( 'NONE',  ( 11.48171059495397728, 82.28518628210146346, 4.944772684328674117 ) ) ;
#33123=CARTESIAN_POINT ( 'NONE',  ( 5.529263428287477744, 43.47268628210144215, -7.954856959092191815 ) ) ;
#33135=CARTESIAN_POINT ( 'NONE',  ( -2.311890736173448424, 78.07731371789856212, 12.53471296425189330 ) ) ;
#33136=CARTESIAN_POINT ( 'NONE',  ( 6.932735513423970097, 101.5476862821014521, 10.69584247140445044 ) ) ;
#33143=CARTESIAN_POINT ( 'NONE',  ( 13.23911966647199812, 76.35231371789853938, 8.632099005475788900 ) ) ;
#33148=CARTESIAN_POINT ( 'NONE',  ( 5.529263428287300108, 49.32731371789854791, 7.954856959092309943 ) ) ;
#33150=CARTESIAN_POINT ( 'NONE',  ( -8.843639120294245259, 108.2648137178985621, -3.474262827703533230 ) ) ;
#33152=CARTESIAN_POINT ( 'NONE',  ( -12.50000000000000355, 34.08981371789854364, 0.1745138560722786503 ) ) ;
#33153=CARTESIAN_POINT ( 'NONE',  ( 7.228626920339068285, 80.27268628210146062, -10.49813415415989581 ) ) ;
#33161=CARTESIAN_POINT ( 'NONE',  ( -2.064181346179269738, 102.6976862821014294, 9.465287035748067623 ) ) ;
#33163=CARTESIAN_POINT ( 'NONE',  ( 4.622313124798573369, 138.6351862821014720, 11.61527771782819940 ) ) ;
#33164=CARTESIAN_POINT ( 'NONE',  ( -11.00000000000001243, 143.0000000000000000, -1.227709706637561792E-13 ) ) ;
#33176=CARTESIAN_POINT ( 'NONE',  ( -0.1745138560723084320, 27.18981371789855572, -9.500000000000005329 ) ) ;
#33181=CARTESIAN_POINT ( 'NONE',  ( -6.932735513424201912, 23.45231371789854791, 10.69584247140429412 ) ) ;
#33183=CARTESIAN_POINT ( 'NONE',  ( -0.1745138560722442889, 137.5898137178985792, -15.50000000000000533 ) ) ;
#33190=CARTESIAN_POINT ( 'NONE',  ( 12.46528703574805874, 137.1976862821014720, 2.660918448318279950 ) ) ;
#33203=CARTESIAN_POINT ( 'NONE',  ( -2.908627838312119351, 125.1226862821014691, -15.53471296425195369 ) ) ;
#33205=CARTESIAN_POINT ( 'NONE',  ( -9.500000000000005329, 113.9101862821014493, -0.1745138560725176813 ) ) ;
#33207=CARTESIAN_POINT ( 'NONE',  ( 12.46528703574805874, 8.397686282101442856, 2.660918448318279950 ) ) ;
#33211=CARTESIAN_POINT ( 'NONE',  ( -5.529263428287477744, 75.67268628210143788, 7.954856959092191815 ) ) ;
#33213=CARTESIAN_POINT ( 'NONE',  ( -3.796722387233375073, 10.98518628210143433, 8.710071997420127943 ) ) ;
#33220=CARTESIAN_POINT ( 'NONE',  ( -8.843639120294245259, 80.66481371789856780, -3.474262827703533230 ) ) ;
#33223=CARTESIAN_POINT ( 'NONE',  ( -12.53471296425189152, 80.37731371789854506, -2.311890736173453309 ) ) ;
#33227=CARTESIAN_POINT ( 'NONE',  ( -0.1745138560722763466, 45.58981371789855075, -12.50000000000000355 ) ) ;
#33232=CARTESIAN_POINT ( 'NONE',  ( -10.49813415415989581, 22.77268628210143575, -7.228626920339068285 ) ) ;
#33237=CARTESIAN_POINT ( 'NONE',  ( 4.944772684328420986, 68.01481371789854791, 11.48171059495408208 ) ) ;
#33241=CARTESIAN_POINT ( 'NONE',  ( -8.927990412390371944, 53.92731371789854222, -13.04141134922778988 ) ) ;
#33245=CARTESIAN_POINT ( 'NONE',  ( 4.622313124798573369, 65.03518628210144925, 11.61527771782819940 ) ) ;
#33246=CARTESIAN_POINT ( 'NONE',  ( -8.632099005475501130, 32.54768628210143788, -13.23911966647218996 ) ) ;
#33250=CARTESIAN_POINT ( 'NONE',  ( 10.83675517735155225, 36.86018628210144499, 11.08355503943142573 ) ) ;
#33257=CARTESIAN_POINT ( 'NONE',  ( 12.46528703574805874, 17.59768628210143859, 2.660918448318279950 ) ) ;
#33259=CARTESIAN_POINT ( 'NONE',  ( -8.843639120294245259, 126.6648137178985820, -3.474262827703533230 ) ) ;
#33271=CARTESIAN_POINT ( 'NONE',  ( 7.228626920339069173, 25.07268628210145067, -10.49813415415989404 ) ) ;
#33279=CARTESIAN_POINT ( 'NONE',  ( -11.61527771782819940, 76.53518628210146346, 4.622313124798574258 ) ) ;
#33280=CARTESIAN_POINT ( 'NONE',  ( -15.53471296425195369, 132.0226862821014322, 2.908627838312118019 ) ) ;
#33287=CARTESIAN_POINT ( 'NONE',  ( -0.1745138560722763466, 137.5898137178985792, -12.50000000000000355 ) ) ;
#33292=CARTESIAN_POINT ( 'NONE',  ( -3.257655550456946880, 118.9023137178985650, -15.46528703574811736 ) ) ;
#33298=CARTESIAN_POINT ( 'NONE',  ( -12.53471296425194836, 132.0226862821014606, 2.311890736173176641 ) ) ;
#33302=CARTESIAN_POINT ( 'NONE',  ( -15.46528703574804986, 95.79768628210145209, -3.257655550457287497 ) ) ;
#33305=CARTESIAN_POINT ( 'NONE',  ( 3.474262827703335166, 37.43518628210144072, 8.843639120294326972 ) ) ;
#33309=CARTESIAN_POINT ( 'NONE',  ( -6.932735513423968321, 69.34768628210143504, -10.69584247140445221 ) ) ;
#33312=CARTESIAN_POINT ( 'NONE',  ( -3.796722387233375073, 38.58518628210143930, 8.710071997420127943 ) ) ;
#33322=CARTESIAN_POINT ( 'NONE',  ( 7.228626920338837358, 76.92731371789857064, 10.49813415416005036 ) ) ;
#33323=CARTESIAN_POINT ( 'NONE',  ( -4.622313124798576922, 78.83518628210146062, -11.61527771782819762 ) ) ;
#33328=CARTESIAN_POINT ( 'NONE',  ( -0.1745138560722442889, 54.78981371789855359, -15.50000000000000533 ) ) ;
#33333=CARTESIAN_POINT ( 'NONE',  ( 8.710071997420211432, 65.71481371789855075, -3.796722387233181895 ) ) ;
#33337=CARTESIAN_POINT ( 'NONE',  ( 1.715153634034445762, 119.4773137178985678, -9.534712964251895073 ) ) ;
#33339=CARTESIAN_POINT ( 'NONE',  ( 2.311890736173452865, 27.47731371789855004, -12.53471296425189152 ) ) ;
#33341=CARTESIAN_POINT ( 'NONE',  ( -6.932735513423968321, 78.54768628210146630, -10.69584247140445221 ) ) ;
#33350=CARTESIAN_POINT ( 'NONE',  ( -3.796722387233375073, 93.78518628210144925, 8.710071997420127943 ) ) ;
#33352=CARTESIAN_POINT ( 'NONE',  ( 2.311890736173175753, 129.7226862821014777, 12.53471296425194836 ) ) ;
#33353=CARTESIAN_POINT ( 'NONE',  ( -10.07132003121360775, 143.0000000000000000, 4.865397298893943123 ) ) ;
#33363=CARTESIAN_POINT ( 'NONE',  ( 6.932735513424201024, 138.4523137178985621, -10.69584247140429412 ) ) ;
#33368=CARTESIAN_POINT ( 'NONE',  ( 4.944772684328420986, 22.01481371789855501, 11.48171059495408208 ) ) ;
#33370=CARTESIAN_POINT ( 'NONE',  ( 3.257655550456945548, 105.1023137178985678, 15.46528703574811736 ) ) ;
#33377=CARTESIAN_POINT ( 'NONE',  ( 2.660918448318279950, 125.6976862821014578, -12.46528703574805697 ) ) ;
#33386=CARTESIAN_POINT ( 'NONE',  ( 12.53471296425194836, 136.6226862821014834, -2.311890736173178418 ) ) ;
#33390=CARTESIAN_POINT ( 'NONE',  ( 14.38691631536207538, 117.9351862821014407, -5.770363421893813793 ) ) ;
#33391=CARTESIAN_POINT ( 'NONE',  ( 6.594114490232313663, 110.4601862821014606, 6.840914352312096547 ) ) ;
#33393=CARTESIAN_POINT ( 'NONE',  ( 12.50000000000000355, 8.110186282101444988, 0.1745138560725507937 ) ) ;
#33398=CARTESIAN_POINT ( 'NONE',  ( -9.534712964251941258, 86.02268628210144641, 1.715153634034234154 ) ) ;
#33399=CARTESIAN_POINT ( 'NONE',  ( -6.594114490232462877, 124.9398137178985451, 6.840914352311949109 ) ) ;
#33405=CARTESIAN_POINT ( 'NONE',  ( -8.152565276336593669, 62.55231371789854222, -5.233372021372610483 ) ) ;
#33409=CARTESIAN_POINT ( 'NONE',  ( -12.50000000000000355, 80.08981371789855075, 0.1745138560722786503 ) ) ;
#33413=CARTESIAN_POINT ( 'NONE',  ( 0.1745138560722779009, 40.98981371789854933, 12.50000000000000355 ) ) ;
#33416=CARTESIAN_POINT ( 'NONE',  ( 12.53471296425194836, 26.22268628210144925, -2.311890736173178418 ) ) ;
#33421=CARTESIAN_POINT ( 'NONE',  ( -12.50000000000000355, 61.68981371789855928, 0.1745138560722786503 ) ) ;
#33425=CARTESIAN_POINT ( 'NONE',  ( 8.632099005475788900, 37.25231371789855217, -13.23911966647199812 ) ) ;
#33428=CARTESIAN_POINT ( 'NONE',  ( 6.932735513423970097, 64.74768628210145494, 10.69584247140445044 ) ) ;
#33429=CARTESIAN_POINT ( 'NONE',  ( 0.1745138560725837118, 15.01018628210143291, -15.50000000000000533 ) ) ;
#33433=CARTESIAN_POINT ( 'NONE',  ( -13.04141134922759804, 22.77268628210143220, -8.927990412390657937 ) ) ;
#33441=CARTESIAN_POINT ( 'NONE',  ( 1.715153634034445762, 119.4773137178985678, -9.534712964251895073 ) ) ;
#33445=CARTESIAN_POINT ( 'NONE',  ( -2.311890736173447980, 142.4773137178985678, 12.53471296425189330 ) ) ;
#33453=CARTESIAN_POINT ( 'NONE',  ( -12.53471296425194659, 30.82268628210144001, 2.311890736173176641 ) ) ;
#33461=CARTESIAN_POINT ( 'NONE',  ( 4.944772684328679446, 70.78518628210144925, -11.48171059495397373 ) ) ;
#33462=CARTESIAN_POINT ( 'NONE',  ( -3.257655550456946880, 8.502313717898553946, -15.46528703574811736 ) ) ;
#33469=CARTESIAN_POINT ( 'NONE',  ( -11.48171059495408208, 125.5148137178985763, 4.944772684328421875 ) ) ;
#33474=CARTESIAN_POINT ( 'NONE',  ( -15.46528703574811736, 98.20231371789854791, 3.257655550456946436 ) ) ;
#33479=CARTESIAN_POINT ( 'NONE',  ( -11.61527771782819940, 122.5351862821014635, 4.622313124798574258 ) ) ;
#33480=CARTESIAN_POINT ( 'NONE',  ( -15.46528703574804986, 77.39768628210144641, -3.257655550457287497 ) ) ;
#33483=CARTESIAN_POINT ( 'NONE',  ( 0.1745138560725837118, 88.61018628210146630, -15.50000000000000533 ) ) ;
#33486=CARTESIAN_POINT ( 'NONE',  ( 1.715153634034233487, 46.92268628210143788, 9.534712964251941258 ) ) ;
#33490=CARTESIAN_POINT ( 'NONE',  ( -11.48171059495397373, 50.08518628210144641, -4.944772684328680334 ) ) ;
#33493=CARTESIAN_POINT ( 'NONE',  ( 9.465287035748067623, 35.99768628210143362, 2.064181346179272847 ) ) ;
#33503=CARTESIAN_POINT ( 'NONE',  ( -11.61527771782809282, 80.66481371789856780, -4.622313124798832717 ) ) ;
#33504=CARTESIAN_POINT ( 'NONE',  ( 0.1745138560725515708, 88.61018628210146630, -12.50000000000000355 ) ) ;
#33510=CARTESIAN_POINT ( 'NONE',  ( 2.908627838312458636, 64.27731371789853654, -15.53471296425188442 ) ) ;
#33516=CARTESIAN_POINT ( 'NONE',  ( -2.064181346179062349, 45.30231371789854933, -9.465287035748106703 ) ) ;
#33519=CARTESIAN_POINT ( 'NONE',  ( 2.064181346179061460, 95.90231371789855075, 9.465287035748106703 ) ) ;
#33521=CARTESIAN_POINT ( 'NONE',  ( -4.622313124798826500, 32.36481371789854933, 11.61527771782809637 ) ) ;
#33522=CARTESIAN_POINT ( 'NONE',  ( -4.944772684328673229, 75.38518628210144357, 11.48171059495397728 ) ) ;
#33531=CARTESIAN_POINT ( 'NONE',  ( -8.152565276336710909, 94.64768628210147483, 5.233372021372435512 ) ) ;
#33535=CARTESIAN_POINT ( 'NONE',  ( -11.48171059495397373, 123.6851862821014549, -4.944772684328680334 ) ) ;
#33546=CARTESIAN_POINT ( 'NONE',  ( -8.843639120294245259, 7.064813717898548617, -3.474262827703533230 ) ) ;
#33547=CARTESIAN_POINT ( 'NONE',  ( -12.53471296425194659, 141.2226862821014777, 2.311890736173176641 ) ) ;
#33557=CARTESIAN_POINT ( 'NONE',  ( 10.83675517735179206, 120.3398137178985507, -11.08355503943118769 ) ) ;
#33565=CARTESIAN_POINT ( 'NONE',  ( -11.61527771782819940, 140.9351862821014834, 4.622313124798574258 ) ) ;
#33573=CARTESIAN_POINT ( 'NONE',  ( -4.944772684328673229, 130.5851862821014606, 11.48171059495397728 ) ) ;
#33578=CARTESIAN_POINT ( 'NONE',  ( -8.927990412390661490, 121.6726862821014521, 13.04141134922759804 ) ) ;
#33580=CARTESIAN_POINT ( 'NONE',  ( 10.69584247140445221, 16.44768628210144001, -6.932735513423970097 ) ) ;
#33584=CARTESIAN_POINT ( 'NONE',  ( -0.1745138560725182642, 84.01018628210145778, 9.500000000000005329 ) ) ;
#33585=CARTESIAN_POINT ( 'NONE',  ( 5.529263428287300108, 132.1273137178985735, 7.954856959092309943 ) ) ;
#33592=CARTESIAN_POINT ( 'NONE',  ( 8.710071997420211432, 56.51481371789856212, -3.796722387233181895 ) ) ;
#33596=CARTESIAN_POINT ( 'NONE',  ( -2.311890736173447980, 68.87731371789855928, 12.53471296425189330 ) ) ;
#33600=CARTESIAN_POINT ( 'NONE',  ( 8.962234695871567070, 21.43981371789854862, 8.715434833792127023 ) ) ;
#33604=CARTESIAN_POINT ( 'NONE',  ( 12.53471296425194836, 7.822686282101448896, -2.311890736173178418 ) ) ;
#33610=CARTESIAN_POINT ( 'NONE',  ( 6.932735513424201024, 74.05231371789855643, -10.69584247140429412 ) ) ;
#33615=CARTESIAN_POINT ( 'NONE',  ( 6.092822981423662299, 31.21481371789855430, 14.25334919248795096 ) ) ;
#33618=CARTESIAN_POINT ( 'NONE',  ( 2.311890736173175753, 74.52268628210146062, 12.53471296425194836 ) ) ;
#33619=CARTESIAN_POINT ( 'NONE',  ( 6.092822981423978490, 15.58518628210145351, -14.25334919248782306 ) ) ;
#33623=CARTESIAN_POINT ( 'NONE',  ( 5.770363421893814682, 37.43518628210144072, 14.38691631536207183 ) ) ;
#33630=CARTESIAN_POINT ( 'NONE',  ( -12.46528703574805697, 3.797686282101447652, -2.660918448318280838 ) ) ;
#33633=CARTESIAN_POINT ( 'NONE',  ( -9.500000000000005329, 116.8898137178985621, 0.1745138560723101806 ) ) ;
#33637=CARTESIAN_POINT ( 'NONE',  ( -11.48171059495408208, 134.7148137178985507, 4.944772684328421875 ) ) ;
#33643=CARTESIAN_POINT ( 'NONE',  ( -0.1745138560725500443, 28.81018628210144072, 12.50000000000000355 ) ) ;
#33650=CARTESIAN_POINT ( 'NONE',  ( -10.49813415415989581, 68.77268628210146062, -7.228626920339068285 ) ) ;
#33651=CARTESIAN_POINT ( 'NONE',  ( 13.23911966647218996, 136.0476862821014379, -8.632099005475504683 ) ) ;
#33657=CARTESIAN_POINT ( 'NONE',  ( -4.622313124798826500, 115.1648137178985678, 11.61527771782809637 ) ) ;
#33662=CARTESIAN_POINT ( 'NONE',  ( 6.092822981423662299, 95.61481371789857064, 14.25334919248795096 ) ) ;
#33666=CARTESIAN_POINT ( 'NONE',  ( 11.61527771782819940, 117.9351862821014549, -4.622313124798573369 ) ) ;
#33668=CARTESIAN_POINT ( 'NONE',  ( -15.50000000000000533, 67.91018628210144925, -0.1745138560725808530 ) ) ;
#33671=CARTESIAN_POINT ( 'NONE',  ( -6.092822981423970496, 93.78518628210144925, 14.25334919248782661 ) ) ;
#33674=CARTESIAN_POINT ( 'NONE',  ( 2.064181346179272847, 33.69768628210143646, -9.465287035748065847 ) ) ;
#33678=CARTESIAN_POINT ( 'NONE',  ( -11.61527771782819940, 48.93518628210144783, 4.622313124798574258 ) ) ;
#33681=CARTESIAN_POINT ( 'NONE',  ( 6.594114490232313663, 27.66018628210143859, 6.840914352312096547 ) ) ;
#33692=CARTESIAN_POINT ( 'NONE',  ( 12.53471296425189330, 84.97731371789855359, 2.311890736173451977 ) ) ;
#33693=CARTESIAN_POINT ( 'NONE',  ( -12.53471296425194659, 86.02268628210146062, 2.311890736173176641 ) ) ;
#33698=CARTESIAN_POINT ( 'NONE',  ( -15.46528703574811736, 61.40231371789855785, 3.257655550456946436 ) ) ;
#33703=CARTESIAN_POINT ( 'NONE',  ( -5.233372021372612259, 41.85231371789854649, 8.152565276336593669 ) ) ;
#33705=CARTESIAN_POINT ( 'NONE',  ( 8.710071997420211432, 93.31481371789855928, -3.796722387233181895 ) ) ;
#33707=CARTESIAN_POINT ( 'NONE',  ( -4.944772684328424539, 8.214813717898532985, -11.48171059495408031 ) ) ;
#33708=CARTESIAN_POINT ( 'NONE',  ( -2.660918448318275509, 56.69768628210145067, 12.46528703574805874 ) ) ;
#33718=CARTESIAN_POINT ( 'NONE',  ( -9.465287035748065847, 95.79768628210145209, -2.064181346179273735 ) ) ;
#33720=CARTESIAN_POINT ( 'NONE',  ( -4.944772684328673229, 112.1851862821014549, 11.48171059495397728 ) ) ;
#33734=CARTESIAN_POINT ( 'NONE',  ( 12.46528703574811558, 139.6023137178985394, -2.660918448318005503 ) ) ;
#33736=ORIENTED_EDGE ( 'NONE', *, *, #32646, .F. ) ;
#33742=CARTESIAN_POINT ( 'NONE',  ( -3.257655550456946880, 118.9023137178985650, -15.46528703574811736 ) ) ;
#33749=CARTESIAN_POINT ( 'NONE',  ( -12.53471296425194836, 113.6226862821014407, 2.311890736173176641 ) ) ;
#33756=CARTESIAN_POINT ( 'NONE',  ( 8.715434833791931624, 110.4601862821014606, 8.962234695871760692 ) ) ;
#33762=CARTESIAN_POINT ( 'NONE',  ( 15.50000000000000533, 118.5101862821014720, 0.1745138560725827404 ) ) ;
#33766=CARTESIAN_POINT ( 'NONE',  ( -12.50000000000000355, 3.510186282101451560, -0.1745138560725492671 ) ) ;
#33769=CARTESIAN_POINT ( 'NONE',  ( -12.50000000000000355, 3.510186282101451560, -0.1745138560725492671 ) ) ;
#33770=CARTESIAN_POINT ( 'NONE',  ( -3.474262827703337830, 88.03518628210144925, -8.843639120294326972 ) ) ;
#33772=CARTESIAN_POINT ( 'NONE',  ( 9.534712964251900402, 130.9773137178985394, 1.715153634034445540 ) ) ;
#33776=CARTESIAN_POINT ( 'NONE',  ( -11.00000000000001243, 143.0000000000000000, -1.227709706637561792E-13 ) ) ;
#33778=CARTESIAN_POINT ( 'NONE',  ( 9.465287035748106703, 66.00231371789855928, -2.064181346179063237 ) ) ;
#33783=CARTESIAN_POINT ( 'NONE',  ( -2.311890736173447980, 59.67731371789855643, 12.53471296425189330 ) ) ;
#33787=CARTESIAN_POINT ( 'NONE',  ( -8.962234695871565293, 35.23981371789855643, -8.715434833792128799 ) ) ;
#33796=CARTESIAN_POINT ( 'NONE',  ( -2.311890736173448424, 59.67731371789855643, 12.53471296425189330 ) ) ;
#33803=CARTESIAN_POINT ( 'NONE',  ( 13.04141134922778988, 47.02731371789855075, -8.927990412390371944 ) ) ;
#33805=CARTESIAN_POINT ( 'NONE',  ( -10.69584247140444866, 21.04768628210144854, 6.932735513423972762 ) ) ;
#33806=CARTESIAN_POINT ( 'NONE',  ( 8.715434833791931624, 73.66018628210144925, 8.962234695871760692 ) ) ;
#33808=CARTESIAN_POINT ( 'NONE',  ( -14.38691631536207183, 12.13518628210144712, 5.770363421893814682 ) ) ;
#33812=CARTESIAN_POINT ( 'NONE',  ( 5.770363421893814682, 28.23518628210144854, 14.38691631536207183 ) ) ;
#33820=CARTESIAN_POINT ( 'NONE',  ( 9.465287035748106703, 121.2023137178985479, -2.064181346179063237 ) ) ;
#33826=CARTESIAN_POINT ( 'NONE',  ( -2.311890736173447980, 124.0773137178985621, 12.53471296425189330 ) ) ;
#33832=CARTESIAN_POINT ( 'NONE',  ( -8.715434833791929847, 32.26018628210145067, -8.962234695871762469 ) ) ;
#33833=VERTEX_POINT ( 'NONE', #33776 ) ;
#33840=CARTESIAN_POINT ( 'NONE',  ( -4.944772684328673229, 66.18518628210144072, 11.48171059495397728 ) ) ;
#33845=CARTESIAN_POINT ( 'NONE',  ( -8.962234695871565293, 118.0398137178985678, -8.715434833792128799 ) ) ;
#33850=CARTESIAN_POINT ( 'NONE',  ( -15.53471296425188442, 98.77731371789855075, -2.908627838312459080 ) ) ;
#33854=CARTESIAN_POINT ( 'NONE',  ( -8.715434833791929847, 115.0601862821014549, -8.962234695871762469 ) ) ;
#33855=CARTESIAN_POINT ( 'NONE',  ( -15.46528703574804986, 58.99768628210144783, -3.257655550457287497 ) ) ;
#33858=CARTESIAN_POINT ( 'NONE',  ( -8.927990412390661490, 84.87268628210145494, 13.04141134922759804 ) ) ;
#33861=CARTESIAN_POINT ( 'NONE',  ( 8.843639120294328748, 25.93518628210144072, -3.474262827703334722 ) ) ;
#33865=CARTESIAN_POINT ( 'NONE',  ( 2.311890736173175753, 65.32268628210144357, 12.53471296425194836 ) ) ;
#33868=CARTESIAN_POINT ( 'NONE',  ( 6.594114490232313663, 18.46018628210144286, 6.840914352312096547 ) ) ;
#33879=CARTESIAN_POINT ( 'NONE',  ( -8.962234695871565293, 81.23981371789855643, -8.715434833792128799 ) ) ;
#33880=CARTESIAN_POINT ( 'NONE',  ( -2.311890736173176641, 88.32268628210145778, -12.53471296425194659 ) ) ;
#33885=CARTESIAN_POINT ( 'NONE',  ( 2.908627838312458636, 55.07731371789854080, -15.53471296425188442 ) ) ;
#33890=CARTESIAN_POINT ( 'NONE',  ( -9.534712964251895073, 43.57731371789854080, -1.715153634034446428 ) ) ;
#33892=CARTESIAN_POINT ( 'NONE',  ( -7.954856959092309943, 97.62731371789854506, 5.529263428287300108 ) ) ;
#33894=CARTESIAN_POINT ( 'NONE',  ( -2.660918448318004614, 17.70231371789854435, -12.46528703574811558 ) ) ;
#33895=CARTESIAN_POINT ( 'NONE',  ( -8.962234695871760692, 57.56018628210145494, 8.715434833791933400 ) ) ;
#33904=CARTESIAN_POINT ( 'NONE',  ( 5.529263428287477744, 80.27268628210143220, -7.954856959092191815 ) ) ;
#33906=CARTESIAN_POINT ( 'NONE',  ( -4.944772684328673229, 121.3851862821014578, 11.48171059495397728 ) ) ;
#33918=CARTESIAN_POINT ( 'NONE',  ( -10.69584247140429412, 136.1523137178985792, -6.932735513424201024 ) ) ;
#33919=CARTESIAN_POINT ( 'NONE',  ( 8.962234695871762469, 135.7601862821014720, -8.715434833791931624 ) ) ;
#33924=CARTESIAN_POINT ( 'NONE',  ( 4.944772684328420986, 12.81481371789855395, 11.48171059495408208 ) ) ;
#33926=CARTESIAN_POINT ( 'NONE',  ( 11.08355503943118769, 113.4398137178985593, 10.83675517735179028 ) ) ;
#33933=CARTESIAN_POINT ( 'NONE',  ( 11.48171059495397728, 109.8851862821014436, 4.944772684328674117 ) ) ;
#33939=CARTESIAN_POINT ( 'NONE',  ( 2.660918448318279950, 125.6976862821014578, -12.46528703574805697 ) ) ;
#33944=CARTESIAN_POINT ( 'NONE',  ( 14.25334919248782661, 128.2851862821014493, 6.092822981423971385 ) ) ;
#33947=CARTESIAN_POINT ( 'NONE',  ( -12.50000000000000355, 12.71018628210143753, -0.1745138560725492671 ) ) ;
#33952=CARTESIAN_POINT ( 'NONE',  ( -8.152565276336710909, 76.24768628210145494, 5.233372021372435512 ) ) ;
#33959=CARTESIAN_POINT ( 'NONE',  ( -3.474262827703527901, 59.96481371789855075, 8.843639120294245259 ) ) ;
#33963=CARTESIAN_POINT ( 'NONE',  ( 11.61527771782809637, 57.66481371789855359, 4.622313124798827388 ) ) ;
#33966=CARTESIAN_POINT ( 'NONE',  ( 2.660918448318002838, 31.50231371789854862, 12.46528703574811558 ) ) ;
#33969=UNCERTAINTY_MEASURE_WITH_UNIT (LENGTH_MEASURE( 1.000000000000000082E-05 ), #32358, 'distance_accuracy_value', 'NONE');
#33977=CARTESIAN_POINT ( 'NONE',  ( -6.932735513424201912, 69.45231371789856212, 10.69584247140429412 ) ) ;
#33981=CARTESIAN_POINT ( 'NONE',  ( 6.092822981423662299, 40.41481371789855359, 14.25334919248795096 ) ) ;
#33983=CARTESIAN_POINT ( 'NONE',  ( -4.622313124798576922, 14.43518628210144250, -11.61527771782819762 ) ) ;
#33985=CARTESIAN_POINT ( 'NONE',  ( -10.69584247140444866, 67.04768628210145209, 6.932735513423972762 ) ) ;
#33986=CARTESIAN_POINT ( 'NONE',  ( -5.770363421893818234, 5.235186282101429001, -14.38691631536207005 ) ) ;
#33990=CARTESIAN_POINT ( 'NONE',  ( 13.04141134922759804, 27.37268628210144428, 8.927990412390657937 ) ) ;
#33998=CARTESIAN_POINT ( 'NONE',  ( 8.152565276336593669, 113.1523137178985650, 5.233372021372610483 ) ) ;
#34004=CARTESIAN_POINT ( 'NONE',  ( 2.311890736173452421, 119.4773137178985678, -12.53471296425189152 ) ) ;
#34018=CARTESIAN_POINT ( 'NONE',  ( -11.48171059495397373, 59.28518628210144215, -4.944772684328680334 ) ) ;
#34026=CARTESIAN_POINT ( 'NONE',  ( 8.715434833792128799, 129.5398137178985678, -8.962234695871567070 ) ) ;
#34033=CARTESIAN_POINT ( 'NONE',  ( 10.83675517735179206, 101.9398137178985735, -11.08355503943118769 ) ) ;
#34037=CARTESIAN_POINT ( 'NONE',  ( 11.48171059495397728, 128.2851862821014493, 4.944772684328674117 ) ) ;
#34038=CARTESIAN_POINT ( 'NONE',  ( -2.908627838312119351, 60.72268628210144925, -15.53471296425195369 ) ) ;
#34041=CARTESIAN_POINT ( 'NONE',  ( 15.46528703574804986, 81.99768628210142651, 3.257655550457285720 ) ) ;
#34044=CARTESIAN_POINT ( 'NONE',  ( 6.840914352312096547, 25.36018628210144854, -6.594114490232313663 ) ) ;
#34048=CARTESIAN_POINT ( 'NONE',  ( 6.932735513423970097, 64.74768628210145494, 10.69584247140445044 ) ) ;
#34051=CARTESIAN_POINT ( 'NONE',  ( 8.843639120294328748, 35.13518628210143646, -3.474262827703334722 ) ) ;
#34062=CARTESIAN_POINT ( 'NONE',  ( 2.311890736173175753, 92.92268628210145209, 12.53471296425194659 ) ) ;
#34067=CARTESIAN_POINT ( 'NONE',  ( -6.092822981423666739, 63.41481371789855359, -14.25334919248795096 ) ) ;
#34072=CARTESIAN_POINT ( 'NONE',  ( 5.233372021372610483, 37.25231371789855217, -8.152565276336593669 ) ) ;
#34075=CARTESIAN_POINT ( 'NONE',  ( -5.233372021372612259, 87.85231371789855359, 8.152565276336593669 ) ) ;
#34077=CARTESIAN_POINT ( 'NONE',  ( -4.944772684328424539, 17.41481371789854649, -11.48171059495408031 ) ) ;
#34078=CARTESIAN_POINT ( 'NONE',  ( -11.61527771782819940, 67.33518628210144641, 4.622313124798574258 ) ) ;
#34087=CARTESIAN_POINT ( 'NONE',  ( -6.840914352312096547, 85.16018628210146346, 6.594114490232313663 ) ) ;
#34090=CARTESIAN_POINT ( 'NONE',  ( 4.622313124798573369, 111.0351862821014635, 11.61527771782819940 ) ) ;
#34102=CARTESIAN_POINT ( 'NONE',  ( 2.660918448318002838, 123.5023137178985735, 12.46528703574811558 ) ) ;
#34108=CARTESIAN_POINT ( 'NONE',  ( 14.25334919248795451, 111.7148137178985792, -6.092822981423661410 ) ) ;
#34114=CARTESIAN_POINT ( 'NONE',  ( 4.944772684328679446, 116.7851862821014635, -11.48171059495397373 ) ) ;
#34121=CARTESIAN_POINT ( 'NONE',  ( -11.61527771782819940, 122.5351862821014635, 4.622313124798574258 ) ) ;
#34126=CARTESIAN_POINT ( 'NONE',  ( -13.23911966647218463, 103.8476862821014493, 8.632099005475506459 ) ) ;
#34127=CARTESIAN_POINT ( 'NONE',  ( 11.61527771782819940, 16.73518628210143788, -4.622313124798573369 ) ) ;
#34129=CARTESIAN_POINT ( 'NONE',  ( 5.233372021372432847, 129.1476862821014322, 8.152565276336710909 ) ) ;
#34136=CARTESIAN_POINT ( 'NONE',  ( -8.710071997420127943, 59.28518628210144925, -3.796722387233380402 ) ) ;
#34144=CARTESIAN_POINT ( 'NONE',  ( 9.534712964251900402, 48.17731371789854222, 1.715153634034445540 ) ) ;
#34148=CARTESIAN_POINT ( 'NONE',  ( -11.61527771782809282, 71.46481371789856496, -4.622313124798832717 ) ) ;
#34151=CARTESIAN_POINT ( 'NONE',  ( -8.715434833792127023, 23.73981371789854578, 8.962234695871568846 ) ) ;
#34153=ORIENTED_EDGE ( 'NONE', *, *, #6580, .F. ) ;
#34169=CARTESIAN_POINT ( 'NONE',  ( -3.257655550456946880, 45.30231371789854933, -15.46528703574811736 ) ) ;
#34171=CARTESIAN_POINT ( 'NONE',  ( -10.69584247140444866, 11.84768628210144925, 6.932735513423972762 ) ) ;
#34173=CARTESIAN_POINT ( 'NONE',  ( -10.49813415415989581, 50.37268628210145494, -7.228626920339068285 ) ) ;
#34174=CARTESIAN_POINT ( 'NONE',  ( -15.46528703574804986, 12.99768628210143362, -3.257655550457287497 ) ) ;
#34178=CARTESIAN_POINT ( 'NONE',  ( 0.1745138560725837118, 5.810186282101448718, -15.50000000000000533 ) ) ;
#34186=CARTESIAN_POINT ( 'NONE',  ( 9.500000000000005329, 112.2898137178985678, -0.1745138560723090149 ) ) ;
#34191=CARTESIAN_POINT ( 'NONE',  ( -11.61527771782809282, 126.6648137178985678, -4.622313124798832717 ) ) ;
#34207=CARTESIAN_POINT ( 'NONE',  ( 7.228626920339068285, 52.67268628210144499, -10.49813415415989581 ) ) ;
#34212=CARTESIAN_POINT ( 'NONE',  ( 12.50000000000000355, 130.6898137178985735, -0.1745138560722771515 ) ) ;
#34218=CARTESIAN_POINT ( 'NONE',  ( -10.83675517735179028, 88.13981371789856212, 11.08355503943118947 ) ) ;
#34222=CARTESIAN_POINT ( 'NONE',  ( -4.944772684328673229, 121.3851862821014578, 11.48171059495397728 ) ) ;
#34223=CARTESIAN_POINT ( 'NONE',  ( 2.908627838312118019, 56.12268628210142651, 15.53471296425195369 ) ) ;
#34227=CARTESIAN_POINT ( 'NONE',  ( -14.25334919248782306, 77.68518628210145494, -6.092822981423979378 ) ) ;
#34230=CARTESIAN_POINT ( 'NONE',  ( -6.594114490232312775, 23.06018628210144783, -6.840914352312096547 ) ) ;
#34234=CARTESIAN_POINT ( 'NONE',  ( 12.53471296425194836, 53.82268628210144357, -2.311890736173178418 ) ) ;
#34237=CARTESIAN_POINT ( 'NONE',  ( -8.152565276336710909, 21.04768628210144499, 5.233372021372435512 ) ) ;
#34249=CARTESIAN_POINT ( 'NONE',  ( -12.50000000000000355, 77.11018628210145209, -0.1745138560725492671 ) ) ;
#34254=CARTESIAN_POINT ( 'NONE',  ( 0.1745138560722461762, 40.98981371789854933, 15.50000000000000533 ) ) ;
#34261=CARTESIAN_POINT ( 'NONE',  ( -0.1745138560723084320, 36.38981371789855501, -9.500000000000005329 ) ) ;
#34264=CARTESIAN_POINT ( 'NONE',  ( 3.474262827703532341, 101.3648137178985706, -8.843639120294245259 ) ) ;
#34266=CARTESIAN_POINT ( 'NONE',  ( 11.08355503943118769, 141.0398137178985678, 10.83675517735179028 ) ) ;
#34268=CARTESIAN_POINT ( 'NONE',  ( 8.962234695871762469, 71.36018628210145209, -8.715434833791931624 ) ) ;
#34270=DIRECTION ( 'NONE',  ( 0.000000000000000000, -0.9932091452657081376, -0.1163425707149433747 ) ) ;
#34276=CARTESIAN_POINT ( 'NONE',  ( 3.796722387233379514, 79.98518628210145209, -8.710071997420127943 ) ) ;
#34280=CARTESIAN_POINT ( 'NONE',  ( -12.46528703574805697, 114.1976862821014720, -2.660918448318280838 ) ) ;
#34293=CARTESIAN_POINT ( 'NONE',  ( 8.962234695871567070, 122.6398137178985621, 8.715434833792127023 ) ) ;
#34299=CARTESIAN_POINT ( 'NONE',  ( -5.770363421894122880, 96.76481371789854791, 14.38691631536194393 ) ) ;
#34300=CARTESIAN_POINT ( 'NONE',  ( 7.228626920339068285, 98.67268628210145209, -10.49813415415989581 ) ) ;
#34303=CARTESIAN_POINT ( 'NONE',  ( -4.944772684328673229, 121.3851862821014578, 11.48171059495397728 ) ) ;
#34309=CARTESIAN_POINT ( 'NONE',  ( 4.622313124798573369, 120.2351862821014663, 11.61527771782819940 ) ) ;
#34314=CARTESIAN_POINT ( 'NONE',  ( 10.83675517735155225, 101.2601862821014436, 11.08355503943142573 ) ) ;
#34316=CARTESIAN_POINT ( 'NONE',  ( -10.49813415415989404, 22.77268628210143930, -7.228626920339069173 ) ) ;
#34317=CARTESIAN_POINT ( 'NONE',  ( -9.465287035748065847, 123.3976862821014606, -2.064181346179273735 ) ) ;
#34322=CARTESIAN_POINT ( 'NONE',  ( 2.064181346179272847, 61.29768628210142367, -9.465287035748065847 ) ) ;
#34330=CARTESIAN_POINT ( 'NONE',  ( -1.715153634034442431, 32.07731371789855501, 9.534712964251900402 ) ) ;
#34334=CARTESIAN_POINT ( 'NONE',  ( 10.49813415416005213, 65.42731371789855643, -7.228626920338837358 ) ) ;
#34337=CARTESIAN_POINT ( 'NONE',  ( 11.48171059495408208, 38.11481371789854222, -4.944772684328420986 ) ) ;
#34341=CARTESIAN_POINT ( 'NONE',  ( 11.61527771782819940, 7.535186282101452804, -4.622313124798573369 ) ) ;
#34354=CARTESIAN_POINT ( 'NONE',  ( -11.08355503943118592, 16.83981371789855430, -10.83675517735179383 ) ) ;
#34356=CARTESIAN_POINT ( 'NONE',  ( 8.962234695871762469, 6.960186282101432198, -8.715434833791931624 ) ) ;
#34357=CARTESIAN_POINT ( 'NONE',  ( -12.53471296425194836, 49.22268628210144215, 2.311890736173176641 ) ) ;
#34360=CARTESIAN_POINT ( 'NONE',  ( -8.927990412390661490, 11.27268628210142865, 13.04141134922759804 ) ) ;
#34370=CARTESIAN_POINT ( 'NONE',  ( -8.710071997420207879, 97.91481371789856780, 3.796722387233182339 ) ) ;
#34378=CARTESIAN_POINT ( 'NONE',  ( 7.228626920338837358, 113.7273137178985820, 10.49813415416005036 ) ) ;
#34390=CARTESIAN_POINT ( 'NONE',  ( 8.715434833791931624, 55.26018628210144357, 8.962234695871760692 ) ) ;
#34399=CARTESIAN_POINT ( 'NONE',  ( -12.50000000000000355, 107.6898137178985735, 0.1745138560722786503 ) ) ;
#34405=CARTESIAN_POINT ( 'NONE',  ( -13.23911966647199812, 71.75231371789854506, -8.632099005475788900 ) ) ;
#34409=CARTESIAN_POINT ( 'NONE',  ( -6.932735513423968321, 96.94768628210145778, -10.69584247140445221 ) ) ;
#34410=CARTESIAN_POINT ( 'NONE',  ( 10.83675517735155225, 64.46018628210146062, 11.08355503943142573 ) ) ;
#34413=CARTESIAN_POINT ( 'NONE',  ( -11.08355503943142573, 66.76018628210144357, 10.83675517735155402 ) ) ;
#34419=CARTESIAN_POINT ( 'NONE',  ( -12.53471296425194836, 30.82268628210144001, 2.311890736173176641 ) ) ;
#34423=CARTESIAN_POINT ( 'NONE',  ( 9.534712964251941258, 17.02268628210144996, -1.715153634034235708 ) ) ;
#34433=CARTESIAN_POINT ( 'NONE',  ( 2.311890736173175753, 65.32268628210144357, 12.53471296425194659 ) ) ;
#34438=CARTESIAN_POINT ( 'NONE',  ( -8.927990412390371944, 44.72731371789853938, -13.04141134922778988 ) ) ;
#34445=CARTESIAN_POINT ( 'NONE',  ( -9.465287035748106703, 15.40231371789854720, 2.064181346179061460 ) ) ;
#34450=CARTESIAN_POINT ( 'NONE',  ( -11.61527771782809282, 16.26481371789853370, -4.622313124798832717 ) ) ;
#34452=CARTESIAN_POINT ( 'NONE',  ( 0.1745138560725515708, 61.01018628210145067, -12.50000000000000355 ) ) ;
#34460=CARTESIAN_POINT ( 'NONE',  ( -9.534712964251941258, 76.82268628210144357, 1.715153634034234154 ) ) ;
#34462=CARTESIAN_POINT ( 'NONE',  ( -12.53471296425194836, 104.4226862821014379, 2.311890736173176641 ) ) ;
#34474=CARTESIAN_POINT ( 'NONE',  ( -4.622313124798826500, 124.3648137178985706, 11.61527771782809637 ) ) ;
#34475=CARTESIAN_POINT ( 'NONE',  ( 11.48171059495397728, 119.0851862821014606, 4.944772684328674117 ) ) ;
#34482=CARTESIAN_POINT ( 'NONE',  ( -6.092822981423666739, 91.01481371789856212, -14.25334919248795096 ) ) ;
#34483=CARTESIAN_POINT ( 'NONE',  ( -6.932735513423968321, 96.94768628210145778, -10.69584247140445221 ) ) ;
#34487=CARTESIAN_POINT ( 'NONE',  ( 8.715434833791931624, 110.4601862821014606, 8.962234695871760692 ) ) ;
#34492=CARTESIAN_POINT ( 'NONE',  ( -8.962234695871760692, 112.7601862821014720, 8.715434833791933400 ) ) ;
#34497=CARTESIAN_POINT ( 'NONE',  ( -15.53471296425195369, 104.4226862821014521, 2.908627838312118019 ) ) ;
#34498=CARTESIAN_POINT ( 'NONE',  ( -10.69584247140444866, 21.04768628210144854, 6.932735513423972762 ) ) ;
#34502=CARTESIAN_POINT ( 'NONE',  ( 1.715153634034233487, 138.9226862821014663, 9.534712964251941258 ) ) ;
#34507=CARTESIAN_POINT ( 'NONE',  ( -0.1745138560725182642, 65.61018628210146630, 9.500000000000005329 ) ) ;
#34513=CARTESIAN_POINT ( 'NONE',  ( -12.50000000000000355, 5.000000000000004441, -1.353084311261909534E-13 ) ) ;
#34514=CARTESIAN_POINT ( 'NONE',  ( 8.152565276336593669, 30.35231371789855359, 5.233372021372610483 ) ) ;
#34520=CARTESIAN_POINT ( 'NONE',  ( 10.69584247140429589, 48.75231371789855217, 6.932735513424201024 ) ) ;
#34523=CARTESIAN_POINT ( 'NONE',  ( 2.311890736173452865, 9.077313717898549683, -12.53471296425189152 ) ) ;
#34539=CARTESIAN_POINT ( 'NONE',  ( -6.092822981423666739, 26.61481371789854933, -14.25334919248795096 ) ) ;
#34541=CARTESIAN_POINT ( 'NONE',  ( 10.69584247140445221, 16.44768628210144001, -6.932735513423970097 ) ) ;
#34542=CARTESIAN_POINT ( 'NONE',  ( -12.46528703574805697, 49.79768628210145209, -2.660918448318280838 ) ) ;
#34552=CARTESIAN_POINT ( 'NONE',  ( 8.710071997420211432, 102.5148137178985621, -3.796722387233181895 ) ) ;
#34560=CARTESIAN_POINT ( 'NONE',  ( 11.61527771782809637, 94.46481371789855075, 4.622313124798827388 ) ) ;
#34564=CARTESIAN_POINT ( 'NONE',  ( -8.715434833792127023, 60.53981371789856070, 8.962234695871568846 ) ) ;
#34573=CARTESIAN_POINT ( 'NONE',  ( -8.715434833791929847, 50.66018628210144925, -8.962234695871762469 ) ) ;
#34579=CARTESIAN_POINT ( 'NONE',  ( 10.69584247140429589, 103.9523137178985621, 6.932735513424201024 ) ) ;
#34584=CARTESIAN_POINT ( 'NONE',  ( -15.46528703574811736, 79.80231371789852801, 3.257655550456946436 ) ) ;
#34588=CARTESIAN_POINT ( 'NONE',  ( -2.311890736173176641, 106.7226862821014635, -12.53471296425194836 ) ) ;
#34589=CARTESIAN_POINT ( 'NONE',  ( 6.092822981423978490, 43.18518628210144072, -14.25334919248782306 ) ) ;
#34592=CARTESIAN_POINT ( 'NONE',  ( -11.08355503943142573, 75.96018628210144641, 10.83675517735155402 ) ) ;
#34598=CARTESIAN_POINT ( 'NONE',  ( 12.50000000000000355, 44.91018628210144215, 0.1745138560725507937 ) ) ;
#34601=CARTESIAN_POINT ( 'NONE',  ( 0.1745138560725194299, 5.810186282101448718, -9.500000000000005329 ) ) ;
#34612=CARTESIAN_POINT ( 'NONE',  ( -12.50000000000000355, 67.91018628210144925, -0.1745138560725492671 ) ) ;
#34617=CARTESIAN_POINT ( 'NONE',  ( 14.25334919248795451, 38.11481371789853512, -6.092822981423661410 ) ) ;
#34624=CARTESIAN_POINT ( 'NONE',  ( -6.594114490232462877, 23.73981371789854222, 6.840914352311949109 ) ) ;
#34629=CARTESIAN_POINT ( 'NONE',  ( 0.1745138560722461762, 132.9898137178985564, 15.50000000000000533 ) ) ;
#34631=CARTESIAN_POINT ( 'NONE',  ( -8.962234695871760692, 48.36018628210145209, 8.715434833791933400 ) ) ;
#34638=CARTESIAN_POINT ( 'NONE',  ( 8.152565276336714462, 80.84768628210143504, -5.233372021372432847 ) ) ;
#34641=CARTESIAN_POINT ( 'NONE',  ( -6.932735513423968321, 96.94768628210145778, -10.69584247140445221 ) ) ;
#34654=CARTESIAN_POINT ( 'NONE',  ( 11.61527771782809637, 122.0648137178985735, 4.622313124798827388 ) ) ;
#34655=CARTESIAN_POINT ( 'NONE',  ( 8.715434833791931624, 128.8601862821014663, 8.962234695871760692 ) ) ;
#34662=CARTESIAN_POINT ( 'NONE',  ( -14.25334919248795096, 97.91481371789856780, 6.092822981423662299 ) ) ;
#34667=CARTESIAN_POINT ( 'NONE',  ( 5.233372021372610483, 83.25231371789854506, -8.152565276336593669 ) ) ;
#34670=CARTESIAN_POINT ( 'NONE',  ( 11.61527771782809637, 57.66481371789855359, 4.622313124798827388 ) ) ;
#34673=CARTESIAN_POINT ( 'NONE',  ( -12.53471296425194836, 104.4226862821014379, 2.311890736173176641 ) ) ;
#34678=CARTESIAN_POINT ( 'NONE',  ( 6.092822981423978490, 107.5851862821014748, -14.25334919248782306 ) ) ;
#34679=CARTESIAN_POINT ( 'NONE',  ( -2.311890736173176641, 23.92268628210143788, -12.53471296425194659 ) ) ;
#34682=CARTESIAN_POINT ( 'NONE',  ( -9.500000000000005329, 132.3101862821014549, -0.1745138560725176813 ) ) ;
#34687=CARTESIAN_POINT ( 'NONE',  ( 3.474262827703335166, 65.03518628210144925, 8.843639120294326972 ) ) ;
#34694=DIRECTION ( 'NONE',  ( 0.000000000000000000, -0.9932091452657081376, -0.1163425707149433747 ) ) ;
#34695=CARTESIAN_POINT ( 'NONE',  ( -9.465287035748106703, 43.00231371789853796, 2.064181346179061460 ) ) ;
#34700=CARTESIAN_POINT ( 'NONE',  ( 4.622313124798831829, 46.16481371789854649, -11.61527771782809282 ) ) ;
#34703=CARTESIAN_POINT ( 'NONE',  ( -12.50000000000000355, 15.68981371789854329, 0.1745138560722786503 ) ) ;
#34720=CARTESIAN_POINT ( 'NONE',  ( 15.46528703574811736, 29.20231371789855501, -3.257655550456947768 ) ) ;
#34723=CARTESIAN_POINT ( 'NONE',  ( 10.69584247140445221, 7.247686282101428290, -6.932735513423970097 ) ) ;
#34725=CARTESIAN_POINT ( 'NONE',  ( -0.1745138560725500443, 56.41018628210145636, 12.50000000000000355 ) ) ;
#34739=CARTESIAN_POINT ( 'NONE',  ( -2.064181346179062349, 100.5023137178985451, -9.465287035748106703 ) ) ;
#34746=CARTESIAN_POINT ( 'NONE',  ( 12.46528703574811558, 102.8023137178985564, -2.660918448318005947 ) ) ;
#34750=CARTESIAN_POINT ( 'NONE',  ( -11.48171059495408208, 70.31481371789854506, 4.944772684328421875 ) ) ;
#34759=CARTESIAN_POINT ( 'NONE',  ( 8.715434833791931624, 36.86018628210144499, 8.962234695871760692 ) ) ;
#34766=CARTESIAN_POINT ( 'NONE',  ( 6.932735513424201024, 110.8523137178985394, -10.69584247140429412 ) ) ;
#34771=CARTESIAN_POINT ( 'NONE',  ( 0.1745138560722461762, 77.78981371789853938, 15.50000000000000533 ) ) ;
#34775=CARTESIAN_POINT ( 'NONE',  ( 12.50000000000000355, 109.3101862821014549, 0.1745138560725507937 ) ) ;
#34776=CARTESIAN_POINT ( 'NONE',  ( -0.1745138560725817967, 38.01018628210144357, 15.50000000000000533 ) ) ;
#34778=CARTESIAN_POINT ( 'NONE',  ( 3.257655550457285720, 70.49768628210145494, -15.46528703574804986 ) ) ;
#34784=CARTESIAN_POINT ( 'NONE',  ( -12.50000000000000355, 40.31018628210144783, -0.1745138560725492671 ) ) ;
#34787=CARTESIAN_POINT ( 'NONE',  ( 9.500000000000005329, 139.8898137178985621, -0.1745138560723090149 ) ) ;
#34797=CARTESIAN_POINT ( 'NONE',  ( -2.660918448318275509, 75.09768628210144925, 12.46528703574805874 ) ) ;
#34803=CARTESIAN_POINT ( 'NONE',  ( -0.1745138560722442889, 45.58981371789855785, -15.50000000000000533 ) ) ;
#34809=CARTESIAN_POINT ( 'NONE',  ( -0.1745138560723084320, 27.18981371789855572, -9.500000000000005329 ) ) ;
#34816=CARTESIAN_POINT ( 'NONE',  ( -5.770363421894122880, 133.5648137178985735, 14.38691631536194393 ) ) ;
#34818=CARTESIAN_POINT ( 'NONE',  ( 4.944772684328679446, 43.18518628210144072, -11.48171059495397373 ) ) ;
#34825=CARTESIAN_POINT ( 'NONE',  ( 6.840914352312096547, 62.16018628210144925, -6.594114490232313663 ) ) ;
#34829=CARTESIAN_POINT ( 'NONE',  ( 11.48171059495397728, 100.6851862821014691, 4.944772684328674117 ) ) ;
#34844=CARTESIAN_POINT ( 'NONE',  ( -0.1745138560722763466, 119.1898137178985593, -12.50000000000000355 ) ) ;
#34845=CARTESIAN_POINT ( 'NONE',  ( 8.715434833791931624, 119.6601862821014493, 8.962234695871760692 ) ) ;
#34850=CARTESIAN_POINT ( 'NONE',  ( -6.092822981423666739, 100.2148137178985650, -14.25334919248795096 ) ) ;
#34854=CARTESIAN_POINT ( 'NONE',  ( 2.064181346179061460, 77.50231371789855928, 9.465287035748106703 ) ) ;
#34857=CARTESIAN_POINT ( 'NONE',  ( -6.932735513424201912, 41.85231371789855359, 10.69584247140429412 ) ) ;
#34860=CARTESIAN_POINT ( 'NONE',  ( -2.660918448318275509, 93.49768628210145494, 12.46528703574805874 ) ) ;
#34864=CARTESIAN_POINT ( 'NONE',  ( 12.46528703574805874, 137.1976862821014720, 2.660918448318279950 ) ) ;
#34866=CARTESIAN_POINT ( 'NONE',  ( 5.770363421893814682, 92.63518628210147199, 14.38691631536207183 ) ) ;
#34867=CARTESIAN_POINT ( 'NONE',  ( 4.944772684328679446, 15.58518628210145351, -11.48171059495397373 ) ) ;
#34871=CARTESIAN_POINT ( 'NONE',  ( 9.465287035748067623, 137.1976862821014436, 2.064181346179272847 ) ) ;
#34877=CARTESIAN_POINT ( 'NONE',  ( 8.710071997420127943, 54.68518628210145494, 3.796722387233375073 ) ) ;
#34885=CARTESIAN_POINT ( 'NONE',  ( 2.064181346179061460, 40.70231371789854791, 9.465287035748106703 ) ) ;
#34890=CARTESIAN_POINT ( 'NONE',  ( -4.944772684328424539, 45.01481371789854791, -11.48171059495408031 ) ) ;
#34893=CARTESIAN_POINT ( 'NONE',  ( 12.50000000000000355, 20.28981371789855004, -0.1745138560722771515 ) ) ;
#34909=CARTESIAN_POINT ( 'NONE',  ( -10.83675517735179028, 14.53981371789855892, 11.08355503943118947 ) ) ;
#34911=CARTESIAN_POINT ( 'NONE',  ( -1.715153634034234598, 134.3226862821014436, -9.534712964251941258 ) ) ;
#34912=CARTESIAN_POINT ( 'NONE',  ( -8.715434833791929847, 50.66018628210144925, -8.962234695871762469 ) ) ;
#34917=CARTESIAN_POINT ( 'NONE',  ( 7.954856959092191815, 18.17268628210144499, 5.529263428287477744 ) ) ;
#34924=CARTESIAN_POINT ( 'NONE',  ( -7.954856959092309943, 88.42731371789855643, 5.529263428287300108 ) ) ;
#34929=CARTESIAN_POINT ( 'NONE',  ( 2.660918448318003282, 95.90231371789856496, 12.46528703574811558 ) ) ;
#34933=CARTESIAN_POINT ( 'NONE',  ( 10.49813415416005213, 74.62731371789855928, -7.228626920338837358 ) ) ;
#34940=CARTESIAN_POINT ( 'NONE',  ( -8.715434833791929847, 32.26018628210145067, -8.962234695871762469 ) ) ;
#34947=CARTESIAN_POINT ( 'NONE',  ( 12.50000000000000355, 112.2898137178985678, -0.1745138560722771515 ) ) ;
#34953=CARTESIAN_POINT ( 'NONE',  ( 15.46528703574811736, 75.20231371789854791, -3.257655550456947768 ) ) ;
#34957=CARTESIAN_POINT ( 'NONE',  ( 8.962234695871762469, 98.96018628210146062, -8.715434833791931624 ) ) ;
#34958=CARTESIAN_POINT ( 'NONE',  ( 11.08355503943142750, 52.96018628210144641, -10.83675517735155225 ) ) ;
#34963=CARTESIAN_POINT ( 'NONE',  ( -3.257655550457281723, 65.89768628210143220, 15.46528703574804986 ) ) ;
#34969=CARTESIAN_POINT ( 'NONE',  ( -12.53471296425194836, 40.02268628210143930, 2.311890736173176641 ) ) ;
#34972=CARTESIAN_POINT ( 'NONE',  ( 5.233372021372432847, 9.547686282101452093, 8.152565276336710909 ) ) ;
#34976=PRODUCT ( 'follower spring', 'follower spring', '', ( #14918 ) ) ;
#34983=CARTESIAN_POINT ( 'NONE',  ( 12.53471296425194659, 63.02268628210144641, -2.311890736173178418 ) ) ;
#34991=CARTESIAN_POINT ( 'NONE',  ( 8.927990412390371944, 30.92731371789853867, 13.04141134922778811 ) ) ;
#34998=CARTESIAN_POINT ( 'NONE',  ( 8.710071997420211432, 19.71481371789854720, -3.796722387233181895 ) ) ;
#35001=SHAPE_DEFINITION_REPRESENTATION ( #9273, #36285 ) ;
#35004=CARTESIAN_POINT ( 'NONE',  ( 6.092822981423662299, 132.4148137178985678, 14.25334919248795096 ) ) ;
#35008=CARTESIAN_POINT ( 'NONE',  ( -8.715434833791929847, 50.66018628210144925, -8.962234695871762469 ) ) ;
#35014=( NAMED_UNIT ( * ) SI_UNIT ( $, .STERADIAN. ) SOLID_ANGLE_UNIT ( ) );
#35016=CARTESIAN_POINT ( 'NONE',  ( -7.954856959092191815, 59.57268628210145067, -5.529263428287477744 ) ) ;
#35018=CARTESIAN_POINT ( 'NONE',  ( -8.962234695871760692, 103.5601862821014549, 8.715434833791933400 ) ) ;
#35030=CARTESIAN_POINT ( 'NONE',  ( -7.228626920338836470, 109.1273137178985735, -10.49813415416005213 ) ) ;
#35031=CARTESIAN_POINT ( 'NONE',  ( -11.61527771782819940, 131.7351862821014663, 4.622313124798574258 ) ) ;
#35036=CARTESIAN_POINT ( 'NONE',  ( 15.46528703574811736, 102.8023137178985422, -3.257655550456947768 ) ) ;
#35040=CARTESIAN_POINT ( 'NONE',  ( -8.843639120294245259, 80.66481371789856780, -3.474262827703533230 ) ) ;
#35043=CARTESIAN_POINT ( 'NONE',  ( 7.228626920338837358, 40.12731371789853796, 10.49813415416005036 ) ) ;
#35045=CARTESIAN_POINT ( 'NONE',  ( 2.311890736173175753, 102.1226862821014691, 12.53471296425194836 ) ) ;
#35048=CARTESIAN_POINT ( 'NONE',  ( -2.660918448318275509, 139.4976862821014549, 12.46528703574805874 ) ) ;
#35050=CARTESIAN_POINT ( 'NONE',  ( 6.092822981423978490, 89.18518628210145494, -14.25334919248782306 ) ) ;
#35054=CARTESIAN_POINT ( 'NONE',  ( -7.954856959092191815, 114.7726862821014322, -5.529263428287477744 ) ) ;
#35056=CARTESIAN_POINT ( 'NONE',  ( 5.770363421893814682, 9.835186282101449962, 14.38691631536207183 ) ) ;
#35061=CARTESIAN_POINT ( 'NONE',  ( -7.954856959092191815, 50.37268628210144783, -5.529263428287477744 ) ) ;
#35069=CARTESIAN_POINT ( 'NONE',  ( -8.843639120294245259, 34.66481371789854649, -3.474262827703533230 ) ) ;
#35073=CARTESIAN_POINT ( 'NONE',  ( -0.1745138560722763466, 45.58981371789855075, -12.50000000000000355 ) ) ;
#35075=CARTESIAN_POINT ( 'NONE',  ( 6.932735513424201024, 9.652313717898541867, -10.69584247140429412 ) ) ;
#35084=SURFACE_SIDE_STYLE ('',( #3628 ) ) ;
#35093=CARTESIAN_POINT ( 'NONE',  ( 6.092822981423662299, 12.81481371789855217, 14.25334919248795096 ) ) ;
#35095=CARTESIAN_POINT ( 'NONE',  ( 3.474262827703335166, 129.4351862821014549, 8.843639120294326972 ) ) ;
#35096=CARTESIAN_POINT ( 'NONE',  ( -7.228626920339069173, 38.87268628210144072, 10.49813415415989581 ) ) ;
#35101=CARTESIAN_POINT ( 'NONE',  ( -1.715153634034234598, 14.72268628210143859, -9.534712964251941258 ) ) ;
#35109=CARTESIAN_POINT ( 'NONE',  ( 5.529263428287300108, 86.12731371789853085, 7.954856959092309943 ) ) ;
#35114=CARTESIAN_POINT ( 'NONE',  ( -0.1745138560722763466, 100.7898137178985536, -12.50000000000000355 ) ) ;
#35118=CARTESIAN_POINT ( 'NONE',  ( -7.228626920338836470, 63.12731371789855217, -10.49813415416005213 ) ) ;
#35125=CARTESIAN_POINT ( 'NONE',  ( 4.622313124798573369, 46.63518628210145067, 11.61527771782819940 ) ) ;
#35129=CARTESIAN_POINT ( 'NONE',  ( -2.660918448318004614, 100.5023137178985593, -12.46528703574811558 ) ) ;
#35134=CARTESIAN_POINT ( 'NONE',  ( -15.46528703574811736, 70.60231371789853938, 3.257655550456946436 ) ) ;
#35138=CARTESIAN_POINT ( 'NONE',  ( -12.53471296425194836, 95.22268628210146346, 2.311890736173176641 ) ) ;
#35139=CARTESIAN_POINT ( 'NONE',  ( 8.632099005475504683, 46.34768628210144925, 13.23911966647218996 ) ) ;
#35144=CARTESIAN_POINT ( 'NONE',  ( 13.23911966647218996, 62.44768628210144357, -8.632099005475504683 ) ) ;
#35150=CARTESIAN_POINT ( 'NONE',  ( 11.61527771782819940, 44.33518628210145351, -4.622313124798573369 ) ) ;
#35152=CARTESIAN_POINT ( 'NONE',  ( -8.710071997420127943, 4.085186282101443744, -3.796722387233380402 ) ) ;
#35165=CARTESIAN_POINT ( 'NONE',  ( 2.660918448318279950, 42.89768628210144641, -12.46528703574805874 ) ) ;
#35172=CARTESIAN_POINT ( 'NONE',  ( -10.69584247140444866, 94.64768628210146062, 6.932735513423972762 ) ) ;
#35173=CARTESIAN_POINT ( 'NONE',  ( -10.83675517735179028, 14.53981371789855892, 11.08355503943118947 ) ) ;
#35180=CARTESIAN_POINT ( 'NONE',  ( 0.1745138560723095977, 13.38981371789854613, 9.500000000000005329 ) ) ;
#35187=CARTESIAN_POINT ( 'NONE',  ( -10.83675517735179028, 124.9398137178985451, 11.08355503943118947 ) ) ;
#35190=CARTESIAN_POINT ( 'NONE',  ( 11.61527771782819940, 44.33518628210145351, -4.622313124798573369 ) ) ;
#35196=CARTESIAN_POINT ( 'NONE',  ( 8.843639120294328748, 62.73518628210145920, -3.474262827703334722 ) ) ;
#35199=CARTESIAN_POINT ( 'NONE',  ( -2.311890736173176641, 97.52268628210144641, -12.53471296425194836 ) ) ;
#35213=CARTESIAN_POINT ( 'NONE',  ( 8.962234695871567070, 104.2398137178985564, 8.715434833792127023 ) ) ;
#35214=CARTESIAN_POINT ( 'NONE',  ( -8.715434833791929847, 105.8601862821014521, -8.962234695871762469 ) ) ;
#35219=CARTESIAN_POINT ( 'NONE',  ( -11.08355503943118592, 81.23981371789855643, -10.83675517735179383 ) ) ;
#35222=CARTESIAN_POINT ( 'NONE',  ( -1.715153634034234598, 97.52268628210144641, -9.534712964251941258 ) ) ;
#35226=CARTESIAN_POINT ( 'NONE',  ( 8.710071997420211432, 74.91481371789855359, -3.796722387233181895 ) ) ;
#35229=CARTESIAN_POINT ( 'NONE',  ( -10.49813415416004858, 51.62731371789855217, 7.228626920338839135 ) ) ;
#35231=CARTESIAN_POINT ( 'NONE',  ( -11.48171059495397373, 105.2851862821014493, -4.944772684328680334 ) ) ;
#35236=CARTESIAN_POINT ( 'NONE',  ( -8.632099005475501130, 87.74768628210144072, -13.23911966647218996 ) ) ;
#35238=CARTESIAN_POINT ( 'NONE',  ( -12.46528703574805874, 3.797686282101447652, -2.660918448318280838 ) ) ;
#35240=CARTESIAN_POINT ( 'NONE',  ( -3.474262827703337830, 106.4351862821014691, -8.843639120294326972 ) ) ;
#35242=CARTESIAN_POINT ( 'NONE',  ( 13.04141134922759804, 8.972686282101431487, 8.927990412390657937 ) ) ;
#35252=CARTESIAN_POINT ( 'NONE',  ( 2.064181346179061460, 13.10231371789855181, 9.465287035748106703 ) ) ;
#35256=CARTESIAN_POINT ( 'NONE',  ( -11.61527771782809282, 43.86481371789854933, -4.622313124798832717 ) ) ;
#35258=CARTESIAN_POINT ( 'NONE',  ( 15.50000000000000533, 130.6898137178985451, -0.1745138560722452326 ) ) ;
#35274=CARTESIAN_POINT ( 'NONE',  ( -3.257655550456946880, 8.502313717898553946, -15.46528703574811736 ) ) ;
#35276=CARTESIAN_POINT ( 'NONE',  ( 7.954856959092191815, 137.7726862821014606, 5.529263428287477744 ) ) ;
#35278=CARTESIAN_POINT ( 'NONE',  ( -8.962234695871760692, 29.96018628210143930, 8.715434833791933400 ) ) ;
#35282=CARTESIAN_POINT ( 'NONE',  ( -14.38691631536207183, 122.5351862821014493, 5.770363421893814682 ) ) ;
#35284=CARTESIAN_POINT ( 'NONE',  ( -0.1745138560723084320, 137.5898137178985792, -9.500000000000005329 ) ) ;
#35292=CARTESIAN_POINT ( 'NONE',  ( -3.474262827703527901, 69.16481371789853938, 8.843639120294245259 ) ) ;
#35296=CARTESIAN_POINT ( 'NONE',  ( -2.660918448318005058, 100.5023137178985593, -12.46528703574811558 ) ) ;
#35300=CARTESIAN_POINT ( 'NONE',  ( -8.962234695871565293, 62.83981371789855785, -8.715434833792128799 ) ) ;
#35309=CARTESIAN_POINT ( 'NONE',  ( 2.660918448318279950, 33.69768628210145067, -12.46528703574805697 ) ) ;
#35314=CARTESIAN_POINT ( 'NONE',  ( -0.1745138560722763466, 91.58981371789856496, -12.50000000000000355 ) ) ;
#35320=CARTESIAN_POINT ( 'NONE',  ( 15.50000000000000533, 57.08981371789855075, -0.1745138560722452326 ) ) ;
#35324=CARTESIAN_POINT ( 'NONE',  ( 0.1745138560725515708, 88.61018628210146630, -12.50000000000000355 ) ) ;
#35325=CARTESIAN_POINT ( 'NONE',  ( -5.770363421893818234, 51.23518628210143788, -14.38691631536207005 ) ) ;
#35328=CARTESIAN_POINT ( 'NONE',  ( -0.1745138560725817967, 47.21018628210144641, 15.50000000000000533 ) ) ;
#35334=CARTESIAN_POINT ( 'NONE',  ( 8.962234695871762469, 16.16018628210144570, -8.715434833791931624 ) ) ;
#35335=CARTESIAN_POINT ( 'NONE',  ( 9.534712964251941258, 7.822686282101448896, -1.715153634034235708 ) ) ;
#35350=CARTESIAN_POINT ( 'NONE',  ( -10.49813415415989404, 41.17268628210143788, -7.228626920339069173 ) ) ;
#35358=CARTESIAN_POINT ( 'NONE',  ( -12.50000000000000355, 95.51018628210144357, -0.1745138560725492671 ) ) ;
#35359=CARTESIAN_POINT ( 'NONE',  ( -3.257655550456946880, 26.90231371789854364, -15.46528703574811736 ) ) ;
#35365=CARTESIAN_POINT ( 'NONE',  ( -6.932735513424201912, 143.0523137178985564, 10.69584247140429412 ) ) ;
#35371=CARTESIAN_POINT ( 'NONE',  ( -2.908627838312453306, 124.0773137178985621, 15.53471296425188797 ) ) ;
#35375=CARTESIAN_POINT ( 'NONE',  ( -12.53471296425194836, 40.02268628210143930, 2.311890736173176641 ) ) ;
#35379=CARTESIAN_POINT ( 'NONE',  ( -14.38691631536207183, 94.93518628210146915, 5.770363421893814682 ) ) ;
#35383=CARTESIAN_POINT ( 'NONE',  ( -2.064181346179269738, 65.89768628210143220, 9.465287035748067623 ) ) ;
#35386=CARTESIAN_POINT ( 'NONE',  ( 4.622313124798573369, 101.8351862821014464, 11.61527771782819940 ) ) ;
#35399=CARTESIAN_POINT ( 'NONE',  ( 6.932735513424201024, 110.8523137178985394, -10.69584247140429412 ) ) ;
#35400=CARTESIAN_POINT ( 'NONE',  ( 8.962234695871762469, 108.1601862821014635, -8.715434833791931624 ) ) ;
#35404=CARTESIAN_POINT ( 'NONE',  ( -8.632099005475794229, 69.45231371789853370, 13.23911966647199812 ) ) ;
#35409=CARTESIAN_POINT ( 'NONE',  ( -8.843639120294326972, 104.1351862821014720, 3.474262827703335166 ) ) ;
#35411=CARTESIAN_POINT ( 'NONE',  ( -9.534712964251895073, 61.97731371789853938, -1.715153634034446428 ) ) ;
#35413=CARTESIAN_POINT ( 'NONE',  ( 3.796722387233182339, 104.8148137178985593, 8.710071997420207879 ) ) ;
#35415=CARTESIAN_POINT ( 'NONE',  ( 6.932735513424201024, 46.45231371789855501, -10.69584247140429412 ) ) ;
#35417=CARTESIAN_POINT ( 'NONE',  ( 11.61527771782819940, 108.7351862821014663, -4.622313124798573369 ) ) ;
#35421=CARTESIAN_POINT ( 'NONE',  ( 2.660918448318279950, 134.8976862821014890, -12.46528703574805697 ) ) ;
#35423=CARTESIAN_POINT ( 'NONE',  ( 15.46528703574804986, 91.19768628210145778, 3.257655550457285720 ) ) ;
#35430=CARTESIAN_POINT ( 'NONE',  ( 8.152565276336714462, 108.4476862821014294, -5.233372021372432847 ) ) ;
#35432=CARTESIAN_POINT ( 'NONE',  ( 13.23911966647218996, 16.44768628210144001, -8.632099005475504683 ) ) ;
#35444=CARTESIAN_POINT ( 'NONE',  ( -6.594114490232462877, 23.73981371789854222, 6.840914352311949109 ) ) ;
#35449=CARTESIAN_POINT ( 'NONE',  ( 4.944772684328420986, 31.21481371789855430, 11.48171059495408208 ) ) ;
#35451=CARTESIAN_POINT ( 'NONE',  ( -8.632099005475794229, 133.8523137178985394, 13.23911966647199812 ) ) ;
#35468=CARTESIAN_POINT ( 'NONE',  ( 15.53471296425195369, 136.6226862821014549, -2.908627838312120684 ) ) ;
#35471=CARTESIAN_POINT ( 'NONE',  ( -1.715153634034234598, 125.1226862821014691, -9.534712964251941258 ) ) ;
#35473=CARTESIAN_POINT ( 'NONE',  ( -10.49813415415989581, 31.97268628210143859, -7.228626920339068285 ) ) ;
#35478=CARTESIAN_POINT ( 'NONE',  ( 13.04141134922759804, 119.3726862821014265, 8.927990412390657937 ) ) ;
#35480=CARTESIAN_POINT ( 'NONE',  ( -9.500000000000005329, 135.2898137178985394, 0.1745138560723101806 ) ) ;
#35486=CARTESIAN_POINT ( 'NONE',  ( -6.594114490232462877, 69.73981371789855643, 6.840914352311949109 ) ) ;
#35490=CARTESIAN_POINT ( 'NONE',  ( 2.311890736173452421, 73.47731371789856780, -12.53471296425189152 ) ) ;
#35494=CARTESIAN_POINT ( 'NONE',  ( 2.311890736173452865, 45.87731371789854506, -12.53471296425189152 ) ) ;
#35503=CARTESIAN_POINT ( 'NONE',  ( -4.944772684328673229, 47.78518628210144925, 11.48171059495397728 ) ) ;
#35509=CARTESIAN_POINT ( 'NONE',  ( -12.50000000000000355, 89.28981371789855359, 0.1745138560722786503 ) ) ;
#35515=CARTESIAN_POINT ( 'NONE',  ( 8.632099005475788900, 55.65231371789855785, -13.23911966647199812 ) ) ;
#35519=CARTESIAN_POINT ( 'NONE',  ( 10.49813415415989581, 82.57268628210145778, 7.228626920339068285 ) ) ;
#35520=CARTESIAN_POINT ( 'NONE',  ( 14.25334919248782661, 27.08518628210144996, 6.092822981423971385 ) ) ;
#35524=CARTESIAN_POINT ( 'NONE',  ( -15.46528703574804986, 49.79768628210144499, -3.257655550457287497 ) ) ;
#35531=CARTESIAN_POINT ( 'NONE',  ( 11.48171059495397728, 27.08518628210144996, 4.944772684328674117 ) ) ;
#35533=CARTESIAN_POINT ( 'NONE',  ( 9.500000000000005329, 121.4898137178985564, -0.1745138560723090149 ) ) ;
#35544=CARTESIAN_POINT ( 'NONE',  ( -0.1745138560725500443, 47.21018628210143930, 12.50000000000000355 ) ) ;
#35549=CARTESIAN_POINT ( 'NONE',  ( -12.50000000000000178, 143.0000000000000000, -1.385339325893353291E-13 ) ) ;
#35552=CARTESIAN_POINT ( 'NONE',  ( -11.61527771782819940, 94.93518628210145494, 4.622313124798574258 ) ) ;
#35553=CARTESIAN_POINT ( 'NONE',  ( 0.1745138560722461762, 22.58981371789854364, 15.50000000000000533 ) ) ;
#35560=CARTESIAN_POINT ( 'NONE',  ( -10.69584247140429412, 136.1523137178985792, -6.932735513424201024 ) ) ;
#35565=CARTESIAN_POINT ( 'NONE',  ( -6.092822981423666739, 109.4148137178985536, -14.25334919248795096 ) ) ;
#35569=CARTESIAN_POINT ( 'NONE',  ( 11.48171059495397728, 27.08518628210144996, 4.944772684328674117 ) ) ;
#35573=CARTESIAN_POINT ( 'NONE',  ( -0.1745138560725817967, 102.4101862821014493, 15.50000000000000533 ) ) ;
#35576=CARTESIAN_POINT ( 'NONE',  ( -8.710071997420127943, 50.08518628210143930, -3.796722387233380402 ) ) ;
#35579=CARTESIAN_POINT ( 'NONE',  ( 4.622313124798573369, 83.43518628210145494, 11.61527771782819940 ) ) ;
#35591=CARTESIAN_POINT ( 'NONE',  ( -7.228626920338836470, 99.92731371789855643, -10.49813415416005213 ) ) ;
#35592=CARTESIAN_POINT ( 'NONE',  ( -7.228626920339070061, 112.4726862821014350, 10.49813415415989404 ) ) ;
#35598=CARTESIAN_POINT ( 'NONE',  ( -3.257655550456946880, 82.10231371789853938, -15.46528703574811736 ) ) ;
#35601=CARTESIAN_POINT ( 'NONE',  ( 9.534712964251941258, 99.82268628210142936, -1.715153634034235708 ) ) ;
#35603=CARTESIAN_POINT ( 'NONE',  ( -8.843639120294245259, 62.26481371789854791, -3.474262827703533230 ) ) ;
#35607=CARTESIAN_POINT ( 'NONE',  ( 3.474262827703532341, 110.5648137178985593, -8.843639120294245259 ) ) ;
#35609=CARTESIAN_POINT ( 'NONE',  ( 0.1745138560722779009, 31.78981371789854649, 12.50000000000000355 ) ) ;
#35611=CARTESIAN_POINT ( 'NONE',  ( 2.660918448318279950, 79.69768628210144357, -12.46528703574805697 ) ) ;
#35615=CARTESIAN_POINT ( 'NONE',  ( 15.53471296425195369, 81.42268628210145209, -2.908627838312120684 ) ) ;
#35619=CARTESIAN_POINT ( 'NONE',  ( -5.233372021372430183, 106.1476862821014322, -8.152565276336710909 ) ) ;
#35621=CARTESIAN_POINT ( 'NONE',  ( 11.48171059495397728, 128.2851862821014493, 4.944772684328674117 ) ) ;
#35632=CARTESIAN_POINT ( 'NONE',  ( 1.715153634034445762, 18.27731371789853299, -9.534712964251895073 ) ) ;
#35637=CARTESIAN_POINT ( 'NONE',  ( 2.660918448318003282, 22.30231371789854933, 12.46528703574811558 ) ) ;
#35640=CARTESIAN_POINT ( 'NONE',  ( 10.83675517735179206, 138.7398137178985564, -11.08355503943118769 ) ) ;
#35648=CARTESIAN_POINT ( 'NONE',  ( 2.660918448318279950, 134.8976862821014890, -12.46528703574805697 ) ) ;
#35659=CARTESIAN_POINT ( 'NONE',  ( 13.04141134922778988, 10.22731371789853405, -8.927990412390371944 ) ) ;
#35661=CARTESIAN_POINT ( 'NONE',  ( -3.796722387233375073, 121.3851862821014578, 8.710071997420127943 ) ) ;
#35663=CARTESIAN_POINT ( 'NONE',  ( -11.61527771782819940, 21.33518628210144641, 4.622313124798574258 ) ) ;
#35666=CARTESIAN_POINT ( 'NONE',  ( 14.25334919248782661, 128.2851862821014493, 6.092822981423971385 ) ) ;
#35669=CARTESIAN_POINT ( 'NONE',  ( 9.465287035748106703, 139.6023137178985394, -2.064181346179063237 ) ) ;
#35676=CARTESIAN_POINT ( 'NONE',  ( -9.500000000000005329, 70.88981371789854791, 0.1745138560723101806 ) ) ;
#35680=CARTESIAN_POINT ( 'NONE',  ( -4.622313124798826500, 78.36481371789855643, 11.61527771782809637 ) ) ;
#35684=CARTESIAN_POINT ( 'NONE',  ( 2.311890736173452865, 55.07731371789855501, -12.53471296425189152 ) ) ;
#35688=CARTESIAN_POINT ( 'NONE',  ( 8.962234695871762469, 25.36018628210144499, -8.715434833791931624 ) ) ;
#35693=CARTESIAN_POINT ( 'NONE',  ( 12.50000000000000355, 84.68981371789854506, -0.1745138560722771515 ) ) ;
#35698=CARTESIAN_POINT ( 'NONE',  ( -15.50000000000000533, 52.48981371789855643, 0.1745138560722471477 ) ) ;
#35700=CIRCLE ( 'NONE', #4240, 1.499999999999990452 ) ;
#35702=CARTESIAN_POINT ( 'NONE',  ( 11.61527771782819940, 90.33518628210144641, -4.622313124798573369 ) ) ;
#35703=CARTESIAN_POINT ( 'NONE',  ( 13.04141134922759804, 36.57268628210144357, 8.927990412390657937 ) ) ;
#35707=CARTESIAN_POINT ( 'NONE',  ( -11.08355503943142573, 48.36018628210145209, 10.83675517735155402 ) ) ;
#35714=CARTESIAN_POINT ( 'NONE',  ( 10.69584247140445221, 25.64768628210143930, -6.932735513423970097 ) ) ;
#35716=CARTESIAN_POINT ( 'NONE',  ( 2.064181346179061460, 123.5023137178985451, 9.465287035748106703 ) ) ;
#35722=CARTESIAN_POINT ( 'NONE',  ( 8.715434833792128799, 138.7398137178985564, -8.962234695871567070 ) ) ;
#35727=CARTESIAN_POINT ( 'NONE',  ( -4.944772684328673229, 56.98518628210144499, 11.48171059495397728 ) ) ;
#35736=CARTESIAN_POINT ( 'NONE',  ( -10.49813415415989581, 77.97268628210144925, -7.228626920339068285 ) ) ;
#35737=CARTESIAN_POINT ( 'NONE',  ( -13.23911966647199812, 16.55231371789855643, -8.632099005475788900 ) ) ;
#35743=CARTESIAN_POINT ( 'NONE',  ( 8.715434833792128799, 138.7398137178985564, -8.962234695871567070 ) ) ;
#35749=CARTESIAN_POINT ( 'NONE',  ( -8.927990412390371944, 118.3273137178985763, -13.04141134922778988 ) ) ;
#35752=CARTESIAN_POINT ( 'NONE',  ( -8.962234695871760692, 20.76018628210144001, 8.715434833791933400 ) ) ;
#35757=CARTESIAN_POINT ( 'NONE',  ( -15.53471296425195369, 104.4226862821014521, 2.908627838312118019 ) ) ;
#35760=CARTESIAN_POINT ( 'NONE',  ( 6.594114490232313663, 36.86018628210144499, 6.840914352312096547 ) ) ;
#35765=CARTESIAN_POINT ( 'NONE',  ( 8.962234695871762469, 71.36018628210145209, -8.715434833791931624 ) ) ;
#35768=CARTESIAN_POINT ( 'NONE',  ( -8.152565276336710909, 39.44768628210144357, 5.233372021372435512 ) ) ;
#35778=CARTESIAN_POINT ( 'NONE',  ( 0.1745138560722779009, 96.18981371789855928, 12.50000000000000355 ) ) ;
#35779=CARTESIAN_POINT ( 'NONE',  ( 12.50000000000000355, 109.3101862821014549, 0.1745138560725507937 ) ) ;
#35786=CARTESIAN_POINT ( 'NONE',  ( -10.83675517735179028, 69.73981371789855643, 11.08355503943118947 ) ) ;
#35789=CARTESIAN_POINT ( 'NONE',  ( -8.152565276336710909, 94.64768628210147483, 5.233372021372435512 ) ) ;
#35791=CARTESIAN_POINT ( 'NONE',  ( 8.152565276336593669, 57.95231371789854791, 5.233372021372610483 ) ) ;
#35793=CARTESIAN_POINT ( 'NONE',  ( 8.152565276336593669, 113.1523137178985650, 5.233372021372610483 ) ) ;
#35795=CARTESIAN_POINT ( 'NONE',  ( -2.660918448318004614, 36.10231371789853938, -12.46528703574811558 ) ) ;
#35798=CARTESIAN_POINT ( 'NONE',  ( 2.311890736173175753, 83.72268628210143504, 12.53471296425194836 ) ) ;
#35806=CARTESIAN_POINT ( 'NONE',  ( -9.534712964251941258, 104.4226862821014521, 1.715153634034234154 ) ) ;
#35809=CARTESIAN_POINT ( 'NONE',  ( -2.311890736173176641, 125.1226862821014549, -12.53471296425194836 ) ) ;
#35810=CARTESIAN_POINT ( 'NONE',  ( -6.396089478038519793, 142.9999999999984652, 10.57287770549605632 ) ) ;
#35821=CARTESIAN_POINT ( 'NONE',  ( -9.465287035748106703, 15.40231371789854720, 2.064181346179061460 ) ) ;
#35827=CARTESIAN_POINT ( 'NONE',  ( -12.46528703574811558, 24.60231371789854649, 2.660918448318004170 ) ) ;
#35829=CARTESIAN_POINT ( 'NONE',  ( -11.08355503943118592, 136.4398137178985735, -10.83675517735179383 ) ) ;
#35836=CARTESIAN_POINT ( 'NONE',  ( -0.1745138560725500443, 130.0101862821014436, 12.50000000000000355 ) ) ;
#35842=CARTESIAN_POINT ( 'NONE',  ( 11.61527771782819940, 136.3351862821014606, -4.622313124798573369 ) ) ;
#35846=CARTESIAN_POINT ( 'NONE',  ( -14.25334919248782306, 132.8851862821014436, -6.092822981423979378 ) ) ;
#35848=CARTESIAN_POINT ( 'NONE',  ( 8.710071997420127943, 109.8851862821014720, 3.796722387233375073 ) ) ;
#35851=CARTESIAN_POINT ( 'NONE',  ( 12.53471296425194836, 26.22268628210144925, -2.311890736173178418 ) ) ;
#35855=CARTESIAN_POINT ( 'NONE',  ( -8.632099005475501130, 115.3476862821014493, -13.23911966647218996 ) ) ;
#35857=CARTESIAN_POINT ( 'NONE',  ( -8.152565276336593669, 136.1523137178985507, -5.233372021372610483 ) ) ;
#35864=CARTESIAN_POINT ( 'NONE',  ( -3.796722387233185003, 81.81481371789855928, -8.710071997420207879 ) ) ;
#35867=CARTESIAN_POINT ( 'NONE',  ( -12.50000000000000355, 89.28981371789855359, 0.1745138560722786503 ) ) ;
#35869=CARTESIAN_POINT ( 'NONE',  ( -6.474010430066216237, 143.0000000000000284, 10.78258735713080796 ) ) ;
#35871=CARTESIAN_POINT ( 'NONE',  ( 12.50000000000000355, 47.88981371789854791, -0.1745138560722771515 ) ) ;
#35875=CARTESIAN_POINT ( 'NONE',  ( 2.311890736173175753, 19.32268628210144712, 12.53471296425194836 ) ) ;
#35880=CARTESIAN_POINT ( 'NONE',  ( -12.53471296425189152, 80.37731371789854506, -2.311890736173453753 ) ) ;
#35886=CARTESIAN_POINT ( 'NONE',  ( 6.092822981423662299, 49.61481371789856354, 14.25334919248795096 ) ) ;
#35890=CARTESIAN_POINT ( 'NONE',  ( 11.61527771782819940, 81.13518628210145778, -4.622313124798573369 ) ) ;
#35892=CARTESIAN_POINT ( 'NONE',  ( 14.25334919248782661, 36.28518628210144215, 6.092822981423971385 ) ) ;
#35896=CARTESIAN_POINT ( 'NONE',  ( -10.83675517735155047, 41.46018628210145351, -11.08355503943142750 ) ) ;
#35902=CARTESIAN_POINT ( 'NONE',  ( -10.69584247140444866, 30.24768628210144783, 6.932735513423972762 ) ) ;
#35904=CARTESIAN_POINT ( 'NONE',  ( -7.954856959092309943, 134.4273137178984996, 5.529263428287300108 ) ) ;
#35909=CARTESIAN_POINT ( 'NONE',  ( 6.932735513424201024, 129.2523137178985451, -10.69584247140429412 ) ) ;
#35915=CARTESIAN_POINT ( 'NONE',  ( -11.61527771782819940, 48.93518628210144783, 4.622313124798574258 ) ) ;
#35924=CARTESIAN_POINT ( 'NONE',  ( 12.53471296425194836, 81.42268628210145209, -2.311890736173178418 ) ) ;
#35925=CARTESIAN_POINT ( 'NONE',  ( -13.23911966647218463, 140.6476862821014322, 8.632099005475506459 ) ) ;
#35931=CARTESIAN_POINT ( 'NONE',  ( 11.48171059495408208, 139.3148137178985451, -4.944772684328420986 ) ) ;
#35938=CARTESIAN_POINT ( 'NONE',  ( -8.632099005475794229, 106.2523137178985451, 13.23911966647199812 ) ) ;
#35942=CARTESIAN_POINT ( 'NONE',  ( 12.46528703574805874, 26.79768628210144144, 2.660918448318279950 ) ) ;
#35946=CARTESIAN_POINT ( 'NONE',  ( -8.632099005475501130, 106.1476862821014322, -13.23911966647218996 ) ) ;
#35950=CARTESIAN_POINT ( 'NONE',  ( 6.840914352312096547, 43.76018628210144357, -6.594114490232313663 ) ) ;
#35955=CARTESIAN_POINT ( 'NONE',  ( 8.962234695871762469, 80.56018628210145494, -8.715434833791931624 ) ) ;
#35958=CARTESIAN_POINT ( 'NONE',  ( 8.710071997420127943, 45.48518628210144499, 3.796722387233375073 ) ) ;
#35969=CARTESIAN_POINT ( 'NONE',  ( 4.944772684328420986, 86.41481371789855359, 11.48171059495408208 ) ) ;
#35970=CARTESIAN_POINT ( 'NONE',  ( 11.61527771782819940, 108.7351862821014663, -4.622313124798573369 ) ) ;
#35975=CARTESIAN_POINT ( 'NONE',  ( -0.1745138560722442889, 82.38981371789856212, -15.50000000000000533 ) ) ;
#35982=CARTESIAN_POINT ( 'NONE',  ( 0.1745138560723095977, 50.18981371789855217, 9.500000000000005329 ) ) ;
#35984=CARTESIAN_POINT ( 'NONE',  ( -0.1745138560723084320, 119.1898137178985593, -9.500000000000005329 ) ) ;
#35986=CARTESIAN_POINT ( 'NONE',  ( -11.48171059495408208, 33.51481371789854791, 4.944772684328421875 ) ) ;
#35987=CARTESIAN_POINT ( 'NONE',  ( 12.53471296425194836, 90.62268628210146915, -2.311890736173178418 ) ) ;
#35995=CARTESIAN_POINT ( 'NONE',  ( -9.534712964251941258, 86.02268628210144641, 1.715153634034234154 ) ) ;
#35998=CARTESIAN_POINT ( 'NONE',  ( 11.61527771782819940, 127.1351862821014578, -4.622313124798573369 ) ) ;
#36010=CARTESIAN_POINT ( 'NONE',  ( 3.796722387233182339, 12.81481371789855217, 8.710071997420207879 ) ) ;
#36015=CARTESIAN_POINT ( 'NONE',  ( -12.46528703574811558, 33.80231371789854933, 2.660918448318004170 ) ) ;
#36017=CARTESIAN_POINT ( 'NONE',  ( -13.23911966647199812, 136.1523137178985507, -8.632099005475788900 ) ) ;
#36023=CARTESIAN_POINT ( 'NONE',  ( 8.715434833791931624, 128.8601862821014663, 8.962234695871760692 ) ) ;
#36030=FACE_OUTER_BOUND ( 'NONE', #15020, .T. ) ;
#36035=CARTESIAN_POINT ( 'NONE',  ( 2.908627838312118019, 129.7226862821014208, 15.53471296425195369 ) ) ;
#36038=CARTESIAN_POINT ( 'NONE',  ( 8.843639120294328748, 117.9351862821014407, -3.474262827703334722 ) ) ;
#36040=CARTESIAN_POINT ( 'NONE',  ( 12.53471296425194836, 7.822686282101448896, -2.311890736173178418 ) ) ;
#36044=CARTESIAN_POINT ( 'NONE',  ( 15.50000000000000533, 118.5101862821014720, 0.1745138560725827404 ) ) ;
#36046=CARTESIAN_POINT ( 'NONE',  ( -1.715153634034234598, 5.522686282101450850, -9.534712964251941258 ) ) ;
#36052=CARTESIAN_POINT ( 'NONE',  ( 5.529263428287300108, 67.72731371789853938, 7.954856959092309943 ) ) ;
#36056=CARTESIAN_POINT ( 'NONE',  ( -4.622313124798826500, 87.56481371789855928, 11.61527771782809637 ) ) ;
#36058=CARTESIAN_POINT ( 'NONE',  ( -6.580120243182696171, 142.9999999999999432, 10.82695099271156280 ) ) ;
#36060=CARTESIAN_POINT ( 'NONE',  ( 11.61527771782809637, 48.46481371789855785, 4.622313124798827388 ) ) ;
#36065=CARTESIAN_POINT ( 'NONE',  ( 12.53471296425194836, 17.02268628210144996, -2.311890736173178418 ) ) ;
#36070=CARTESIAN_POINT ( 'NONE',  ( 4.622313124798831829, 73.76481371789856212, -11.61527771782809282 ) ) ;
#36075=CARTESIAN_POINT ( 'NONE',  ( -3.257655550456946880, 63.70231371789854791, -15.46528703574811736 ) ) ;
#36078=CARTESIAN_POINT ( 'NONE',  ( -7.228626920339069173, 94.07268628210145778, 10.49813415415989581 ) ) ;
#36079=CARTESIAN_POINT ( 'NONE',  ( -5.770363421893818234, 23.63518628210144357, -14.38691631536207005 ) ) ;
#36084=CARTESIAN_POINT ( 'NONE',  ( 15.50000000000000533, 35.71018628210144641, 0.1745138560725827404 ) ) ;
#36090=CARTESIAN_POINT ( 'NONE',  ( 6.932735513423970097, 18.74768628210143717, 10.69584247140445044 ) ) ;
#36092=CARTESIAN_POINT ( 'NONE',  ( 5.233372021372610483, 129.2523137178985451, -8.152565276336593669 ) ) ;
#36097=CARTESIAN_POINT ( 'NONE',  ( 10.49813415416005213, 129.8273137178985621, -7.228626920338837358 ) ) ;
#36104=CARTESIAN_POINT ( 'NONE',  ( 8.962234695871762469, 34.56018628210144783, -8.715434833791931624 ) ) ;
#36112=CARTESIAN_POINT ( 'NONE',  ( 10.49813415415989581, 73.37268628210144072, 7.228626920339068285 ) ) ;
#36114=CARTESIAN_POINT ( 'NONE',  ( -15.50000000000000533, 132.3101862821014549, -0.1745138560725808530 ) ) ;
#36121=CARTESIAN_POINT ( 'NONE',  ( -9.500000000000005329, 6.489813717898557321, 0.1745138560723101806 ) ) ;
#36126=CARTESIAN_POINT ( 'NONE',  ( -15.46528703574811736, 116.6023137178985394, 3.257655550456946436 ) ) ;
#36131=CARTESIAN_POINT ( 'NONE',  ( -4.622313124798576922, 134.0351862821014493, -11.61527771782819762 ) ) ;
#36134=CARTESIAN_POINT ( 'NONE',  ( -8.632099005475501130, 96.94768628210147199, -13.23911966647218996 ) ) ;
#36137=CARTESIAN_POINT ( 'NONE',  ( -8.710071997420127943, 40.88518628210145067, -3.796722387233380402 ) ) ;
#36141=CARTESIAN_POINT ( 'NONE',  ( -6.932735513423968321, 78.54768628210146630, -10.69584247140445221 ) ) ;
#36143=CARTESIAN_POINT ( 'NONE',  ( -9.500000000000005329, 40.31018628210145494, -0.1745138560725176813 ) ) ;
#36152=CARTESIAN_POINT ( 'NONE',  ( 4.944772684328420986, 77.21481371789855075, 11.48171059495408208 ) ) ;
#36153=CARTESIAN_POINT ( 'NONE',  ( 8.715434833791931624, 82.86018628210145209, 8.962234695871760692 ) ) ;
#36158=CARTESIAN_POINT ( 'NONE',  ( -5.770363421894122880, 59.96481371789855075, 14.38691631536194393 ) ) ;
#36163=CARTESIAN_POINT ( 'NONE',  ( -1.715153634034442431, 59.67731371789855643, 9.534712964251900402 ) ) ;
#36166=CARTESIAN_POINT ( 'NONE',  ( -9.534712964251895073, 117.1773137178985706, -1.715153634034446428 ) ) ;
#36168=CARTESIAN_POINT ( 'NONE',  ( 11.48171059495408208, 38.11481371789854222, -4.944772684328420986 ) ) ;
#36169=CARTESIAN_POINT ( 'NONE',  ( 12.46528703574805874, 81.99768628210146915, 2.660918448318279950 ) ) ;
#36177=CARTESIAN_POINT ( 'NONE',  ( -8.152565276336710909, 103.8476862821014493, 5.233372021372435512 ) ) ;
#36180=CARTESIAN_POINT ( 'NONE',  ( -12.50000000000000355, 132.3101862821014549, -0.1745138560725492671 ) ) ;
#36191=CARTESIAN_POINT ( 'NONE',  ( 2.311890736173452865, 137.8773137178986019, -12.53471296425189152 ) ) ;
#36196=CARTESIAN_POINT ( 'NONE',  ( -4.622313124798826500, 23.16481371789855359, 11.61527771782809637 ) ) ;
#36198=CARTESIAN_POINT ( 'NONE',  ( 13.04141134922778988, 111.4273137178985422, -8.927990412390371944 ) ) ;
#36205=CARTESIAN_POINT ( 'NONE',  ( -12.50000000000000355, 132.3101862821014549, -0.1745138560725492671 ) ) ;
#36214=CARTESIAN_POINT ( 'NONE',  ( -0.1745138560725500443, 139.2101862821014606, 12.50000000000000355 ) ) ;
#36218=CARTESIAN_POINT ( 'NONE',  ( -0.1745138560725817967, 111.6101862821014521, 15.50000000000000533 ) ) ;
#36221=CARTESIAN_POINT ( 'NONE',  ( -0.1745138560725182642, 111.6101862821014521, 9.500000000000005329 ) ) ;
#36223=CARTESIAN_POINT ( 'NONE',  ( 10.69584247140445221, 7.247686282101428290, -6.932735513423970097 ) ) ;
#36229=CARTESIAN_POINT ( 'NONE',  ( 3.796722387233379514, 89.18518628210145494, -8.710071997420127943 ) ) ;
#36231=CARTESIAN_POINT ( 'NONE',  ( -9.465287035748106703, 125.8023137178985706, 2.064181346179061460 ) ) ;
#36237=CARTESIAN_POINT ( 'NONE',  ( -1.715153634034442431, 59.67731371789855643, 9.534712964251900402 ) ) ;
#36240=CARTESIAN_POINT ( 'NONE',  ( 2.660918448318003282, 86.70231371789854791, 12.46528703574811558 ) ) ;
#36242=CARTESIAN_POINT ( 'NONE',  ( -9.164001878794323375, 143.0000000000000000, 9.815649414211552681 ) ) ;
#36244=CARTESIAN_POINT ( 'NONE',  ( -8.715434833792127023, 42.13981371789854791, 8.962234695871568846 ) ) ;
#36248=CARTESIAN_POINT ( 'NONE',  ( 12.46528703574805874, 26.79768628210144144, 2.660918448318279950 ) ) ;
#36253=CARTESIAN_POINT ( 'NONE',  ( 12.46528703574811558, 66.00231371789855928, -2.660918448318005503 ) ) ;
#36259=CARTESIAN_POINT ( 'NONE',  ( -10.83675517735179028, 42.13981371789854791, 11.08355503943118947 ) ) ;
#36262=CARTESIAN_POINT ( 'NONE',  ( -12.50000000000000355, 67.91018628210144925, -0.1745138560725492671 ) ) ;
#36263=CARTESIAN_POINT ( 'NONE',  ( 14.38691631536207538, 35.13518628210143646, -5.770363421893813793 ) ) ;
#36266=CARTESIAN_POINT ( 'NONE',  ( -2.908627838312119351, 33.12268628210143362, -15.53471296425195369 ) ) ;
#36274=CARTESIAN_POINT ( 'NONE',  ( -6.594114490232462877, 124.9398137178985451, 6.840914352311949109 ) ) ;
#36285=SHAPE_REPRESENTATION ( 'follower spring', ( #17215 ), #1426 ) ;
#36286=CARTESIAN_POINT ( 'NONE',  ( 11.48171059495397728, 36.28518628210144925, 4.944772684328674117 ) ) ;
#36293=CARTESIAN_POINT ( 'NONE',  ( 12.50000000000000355, 72.51018628210145778, 0.1745138560725507937 ) ) ;
#36294=CARTESIAN_POINT ( 'NONE',  ( -15.50000000000000533, 141.5101862821014720, -0.1745138560725808530 ) ) ;
#36300=CARTESIAN_POINT ( 'NONE',  ( 10.49813415416005213, 129.8273137178985905, -7.228626920338837358 ) ) ;
#36306=CARTESIAN_POINT ( 'NONE',  ( 8.632099005475788900, 120.0523137178985280, -13.23911966647199812 ) ) ;
#36310=CARTESIAN_POINT ( 'NONE',  ( 6.932735513423970097, 129.1476862821014890, 10.69584247140445044 ) ) ;
#36311=CARTESIAN_POINT ( 'NONE',  ( -8.632099005475501130, 78.54768628210145209, -13.23911966647218996 ) ) ;
#36315=CARTESIAN_POINT ( 'NONE',  ( -14.25334919248782306, 86.88518628210145778, -6.092822981423979378 ) ) ;
#36319=CARTESIAN_POINT ( 'NONE',  ( -9.465287035748065847, 40.59768628210144215, -2.064181346179273735 ) ) ;
#36323=CARTESIAN_POINT ( 'NONE',  ( -2.311890736173176641, 79.12268628210145494, -12.53471296425194836 ) ) ;
#36326=CARTESIAN_POINT ( 'NONE',  ( 9.500000000000005329, 35.71018628210144641, 0.1745138560725188748 ) ) ;
#36336=CARTESIAN_POINT ( 'NONE',  ( 10.49813415416005213, 83.82731371789856212, -7.228626920338837358 ) ) ;
#36337=CARTESIAN_POINT ( 'NONE',  ( -12.46528703574805874, 77.39768628210144641, -2.660918448318280838 ) ) ;
#36343=CARTESIAN_POINT ( 'NONE',  ( -8.632099005475794229, 60.25231371789854506, 13.23911966647199812 ) ) ;
#36349=CARTESIAN_POINT ( 'NONE',  ( 9.500000000000005329, 47.88981371789855501, -0.1745138560723090149 ) ) ;
#36351=CARTESIAN_POINT ( 'NONE',  ( 9.534712964251900402, 103.3773137178985451, 1.715153634034445540 ) ) ;
#36353=CARTESIAN_POINT ( 'NONE',  ( -10.49813415416004858, 24.02731371789855785, 7.228626920338839135 ) ) ;
#36355=CARTESIAN_POINT ( 'NONE',  ( -12.50000000000000355, 86.31018628210145494, -0.1745138560725492671 ) ) ;
#36363=CARTESIAN_POINT ( 'NONE',  ( -5.529263428287477744, 94.07268628210144357, 7.954856959092191815 ) ) ;
#36366=CARTESIAN_POINT ( 'NONE',  ( 6.932735513423970097, 129.1476862821014890, 10.69584247140445044 ) ) ;
#36378=CARTESIAN_POINT ( 'NONE',  ( -9.534712964251895073, 6.777313717898553413, -1.715153634034446428 ) ) ;
#36383=CARTESIAN_POINT ( 'NONE',  ( -10.49813415416004858, 14.82731371789855501, 7.228626920338840023 ) ) ;
#36385=CARTESIAN_POINT ( 'NONE',  ( -15.46528703574811736, 107.4023137178985650, 3.257655550456946436 ) ) ;
#36392=CARTESIAN_POINT ( 'NONE',  ( -11.48171059495397373, 123.6851862821014549, -4.944772684328680334 ) ) ;
#36399=CARTESIAN_POINT ( 'NONE',  ( -8.962234695871760692, 131.1601862821014777, 8.715434833791933400 ) ) ;
#36405=CARTESIAN_POINT ( 'NONE',  ( 13.04141134922759804, 119.3726862821014265, 8.927990412390657937 ) ) ;
#36407=CARTESIAN_POINT ( 'NONE',  ( -2.660918448318275509, 10.69768628210143646, 12.46528703574805874 ) ) ;
#36411=CARTESIAN_POINT ( 'NONE',  ( 6.594114490232313663, 73.66018628210144925, 6.840914352312096547 ) ) ;
#36413=CARTESIAN_POINT ( 'NONE',  ( -7.954856959092309943, 134.4273137178984996, 5.529263428287300108 ) ) ;
#36419=CARTESIAN_POINT ( 'NONE',  ( -0.1745138560723084320, 54.78981371789855359, -9.500000000000005329 ) ) ;
#36424=CARTESIAN_POINT ( 'NONE',  ( -10.69584247140429412, 53.35231371789856070, -6.932735513424201024 ) ) ;
#36428=CARTESIAN_POINT ( 'NONE',  ( -10.49813415416004858, 24.02731371789855785, 7.228626920338839135 ) ) ;
#36431=CARTESIAN_POINT ( 'NONE',  ( 12.46528703574805874, 17.59768628210143859, 2.660918448318279950 ) ) ;
#36439=CARTESIAN_POINT ( 'NONE',  ( -2.660918448318004614, 63.70231371789855501, -12.46528703574811558 ) ) ;
#36444=CARTESIAN_POINT ( 'NONE',  ( -5.770363421894122880, 32.36481371789854933, 14.38691631536194393 ) ) ;
#36447=CARTESIAN_POINT ( 'NONE',  ( 10.69584247140445221, 71.64768628210146062, -6.932735513423970097 ) ) ;
#36448=CARTESIAN_POINT ( 'NONE',  ( 15.50000000000000533, 17.31018628210144428, 0.1745138560725827404 ) ) ;
#36453=CARTESIAN_POINT ( 'NONE',  ( 8.632099005475504683, 27.94768628210144001, 13.23911966647218996 ) ) ;
#36459=CARTESIAN_POINT ( 'NONE',  ( 10.49813415415989581, 8.972686282101431487, 7.228626920339068285 ) ) ;
#36461=CARTESIAN_POINT ( 'NONE',  ( -9.465287035748106703, 116.6023137178985394, 2.064181346179061460 ) ) ;
#36473=CARTESIAN_POINT ( 'NONE',  ( 7.228626920339069173, 34.27268628210144641, -10.49813415415989404 ) ) ;
#36481=CARTESIAN_POINT ( 'NONE',  ( -6.932735513423968321, 69.34768628210143504, -10.69584247140445221 ) ) ;
#36482=CARTESIAN_POINT ( 'NONE',  ( -15.53471296425195369, 141.2226862821014493, 2.908627838312118019 ) ) ;
#36488=CARTESIAN_POINT ( 'NONE',  ( -11.48171059495408208, 116.3148137178985593, 4.944772684328421875 ) ) ;
#36494=CARTESIAN_POINT ( 'NONE',  ( -6.092822981423666739, 91.01481371789856212, -14.25334919248795096 ) ) ;
#36499=CARTESIAN_POINT ( 'NONE',  ( 6.932735513423970097, 119.9476862821014578, 10.69584247140445044 ) ) ;
#36500=CARTESIAN_POINT ( 'NONE',  ( -8.632099005475501130, 60.14768628210144641, -13.23911966647218996 ) ) ;
#36502=CARTESIAN_POINT ( 'NONE',  ( -8.927990412390661490, 94.07268628210144357, 13.04141134922759804 ) ) ;
#36507=CARTESIAN_POINT ( 'NONE',  ( 5.529263428287477744, 34.27268628210144641, -7.954856959092191815 ) ) ;
#36511=CARTESIAN_POINT ( 'NONE',  ( 10.69584247140445221, 53.24768628210144072, -6.932735513423970097 ) ) ;
#36514=CARTESIAN_POINT ( 'NONE',  ( 1.715153634034233487, 19.32268628210144001, 9.534712964251941258 ) ) ;
#36524=CARTESIAN_POINT ( 'NONE',  ( -2.660918448318004614, 91.30231371789857064, -12.46528703574811558 ) ) ;
#36525=CARTESIAN_POINT ( 'NONE',  ( -8.715434833791929847, 87.46018628210144641, -8.962234695871762469 ) ) ;
#36530=CARTESIAN_POINT ( 'NONE',  ( 10.83675517735179206, 55.93981371789855217, -11.08355503943118769 ) ) ;
#36537=CARTESIAN_POINT ( 'NONE',  ( 9.465287035748106703, 38.40231371789853654, -2.064181346179063237 ) ) ;
#36539=CARTESIAN_POINT ( 'NONE',  ( -6.840914352311947333, 90.43981371789854506, -6.594114490232462877 ) ) ;
#36541=CARTESIAN_POINT ( 'NONE',  ( 2.311890736173452865, 9.077313717898549683, -12.53471296425189152 ) ) ;
#36542=CARTESIAN_POINT ( 'NONE',  ( -7.228626920339069173, 57.27268628210144641, 10.49813415415989581 ) ) ;
#36551=CARTESIAN_POINT ( 'NONE',  ( 8.152565276336714462, 90.04768628210145209, -5.233372021372432847 ) ) ;
#36553=CARTESIAN_POINT ( 'NONE',  ( 12.50000000000000355, 118.5101862821014578, 0.1745138560725507937 ) ) ;
#36554=CARTESIAN_POINT ( 'NONE',  ( -6.392720816132698936, 142.9999999999999147, 10.60379120543304055 ) ) ;
#36565=CARTESIAN_POINT ( 'NONE',  ( 7.954856959092311719, 10.22731371789853405, -5.529263428287300108 ) ) ;
#36571=CARTESIAN_POINT ( 'NONE',  ( -2.311890736173447980, 13.67731371789854222, 12.53471296425189330 ) ) ;
#36574=CARTESIAN_POINT ( 'NONE',  ( -14.38691631536193860, 117.4648137178985650, -5.770363421894132649 ) ) ;
#36581=CARTESIAN_POINT ( 'NONE',  ( 12.50000000000000355, 109.3101862821014549, 0.1745138560725507937 ) ) ;
#36589=CARTESIAN_POINT ( 'NONE',  ( -0.1745138560725500443, 130.0101862821014436, 12.50000000000000355 ) ) ;
#36594=CARTESIAN_POINT ( 'NONE',  ( 6.092822981423978490, 125.9851862821014521, -14.25334919248782306 ) ) ;
#36596=CARTESIAN_POINT ( 'NONE',  ( -12.46528703574805697, 3.797686282101447652, -2.660918448318280838 ) ) ;
#36600=CARTESIAN_POINT ( 'NONE',  ( -9.500000000000005329, 86.31018628210145494, -0.1745138560725176813 ) ) ;
#36601=CARTESIAN_POINT ( 'NONE',  ( 9.500000000000005329, 130.6898137178985451, -0.1745138560723090149 ) ) ;
#36608=CARTESIAN_POINT ( 'NONE',  ( -9.500000000000005329, 61.68981371789855928, 0.1745138560723101806 ) ) ;
#36612=CARTESIAN_POINT ( 'NONE',  ( 11.48171059495408208, 65.71481371789855075, -4.944772684328420986 ) ) ;
#36616=CARTESIAN_POINT ( 'NONE',  ( 4.944772684328420986, 31.21481371789855430, 11.48171059495408208 ) ) ;
#36620=CARTESIAN_POINT ( 'NONE',  ( 4.622313124798573369, 9.835186282101449962, 11.61527771782819940 ) ) ;
#36627=CARTESIAN_POINT ( 'NONE',  ( -12.46528703574811558, 61.40231371789855785, 2.660918448318003726 ) ) ;
#36633=CARTESIAN_POINT ( 'NONE',  ( -13.23911966647199812, 44.15231371789854364, -8.632099005475788900 ) ) ;
#36635=CARTESIAN_POINT ( 'NONE',  ( 0.1745138560725515708, 24.21018628210144641, -12.50000000000000355 ) ) ;
#36637=CARTESIAN_POINT ( 'NONE',  ( -12.46528703574805697, 58.99768628210144783, -2.660918448318280838 ) ) ;
#36638=CARTESIAN_POINT ( 'NONE',  ( 14.25334919248782661, 8.685186282101437172, 6.092822981423971385 ) ) ;
#36642=CARTESIAN_POINT ( 'NONE',  ( -11.08355503943142573, 39.16018628210144215, 10.83675517735155402 ) ) ;
#36649=CARTESIAN_POINT ( 'NONE',  ( -8.962234695871760692, 11.56018628210145316, 8.715434833791933400 ) ) ;
#36652=CARTESIAN_POINT ( 'NONE',  ( 8.710071997420211432, 120.9148137178985678, -3.796722387233181895 ) ) ;
#36658=CARTESIAN_POINT ( 'NONE',  ( 4.944772684328420986, 114.0148137178985621, 11.48171059495408208 ) ) ;
#36664=CARTESIAN_POINT ( 'NONE',  ( 10.69584247140445221, 25.64768628210144286, -6.932735513423970097 ) ) ;
#36673=CARTESIAN_POINT ( 'NONE',  ( -4.622313124798576922, 51.23518628210143788, -11.61527771782819762 ) ) ;
#36674=CARTESIAN_POINT ( 'NONE',  ( -10.83675517735155047, 133.4601862821014606, -11.08355503943142750 ) ) ;
#36680=CARTESIAN_POINT ( 'NONE',  ( 4.622313124798831829, 128.9648137178985507, -11.61527771782809282 ) ) ;
#36685=CARTESIAN_POINT ( 'NONE',  ( -0.1745138560722442889, 100.7898137178985536, -15.50000000000000533 ) ) ;
#36689=CARTESIAN_POINT ( 'NONE',  ( -4.622313124798576922, 124.8351862821014748, -11.61527771782819762 ) ) ;
#36690=CARTESIAN_POINT ( 'NONE',  ( -13.23911966647218463, 67.04768628210143788, 8.632099005475506459 ) ) ;
#36693=CARTESIAN_POINT ( 'NONE',  ( 6.092822981423978490, 79.98518628210145209, -14.25334919248782306 ) ) ;
#36696=CARTESIAN_POINT ( 'NONE',  ( -6.594114490232312775, 13.86018628210145032, -6.840914352312096547 ) ) ;
#36701=CARTESIAN_POINT ( 'NONE',  ( 8.715434833791931624, 64.46018628210146062, 8.962234695871760692 ) ) ;
#36704=CARTESIAN_POINT ( 'NONE',  ( -9.465287035748065847, 22.19768628210144001, -2.064181346179273735 ) ) ;
#36715=CARTESIAN_POINT ( 'NONE',  ( -7.228626920338836470, 90.72731371789853938, -10.49813415416005213 ) ) ;
#36716=CARTESIAN_POINT ( 'NONE',  ( -8.962234695871760692, 85.16018628210144925, 8.715434833791933400 ) ) ;
#36721=CARTESIAN_POINT ( 'NONE',  ( -15.50000000000000533, 52.48981371789855643, 0.1745138560722471477 ) ) ;
#36727=CARTESIAN_POINT ( 'NONE',  ( -9.465287035748106703, 33.80231371789854222, 2.064181346179061460 ) ) ;
#36729=CARTESIAN_POINT ( 'NONE',  ( -3.474262827703527901, 87.56481371789857349, 8.843639120294245259 ) ) ;
#36731=CARTESIAN_POINT ( 'NONE',  ( -10.69584247140429412, 7.352313717898545598, -6.932735513424201024 ) ) ;
#36732=CARTESIAN_POINT ( 'NONE',  ( -8.715434833791929847, 69.06018628210145494, -8.962234695871762469 ) ) ;
#36741=CARTESIAN_POINT ( 'NONE',  ( -9.500000000000005329, 86.31018628210145494, -0.1745138560725176813 ) ) ;
#36743=CARTESIAN_POINT ( 'NONE',  ( -8.962234695871760692, 121.9601862821014464, 8.715434833791933400 ) ) ;
#36756=CARTESIAN_POINT ( 'NONE',  ( -4.944772684328424539, 137.0148137178985621, -11.48171059495408031 ) ) ;
#36763=CARTESIAN_POINT ( 'NONE',  ( -0.1745138560722442889, 119.1898137178985593, -15.50000000000000533 ) ) ;
#36768=CARTESIAN_POINT ( 'NONE',  ( 2.660918448318279950, 107.2976862821014521, -12.46528703574805697 ) ) ;
#36773=CARTESIAN_POINT ( 'NONE',  ( -11.61527771782819940, 113.3351862821014606, 4.622313124798574258 ) ) ;
#36779=CARTESIAN_POINT ( 'NONE',  ( -13.04141134922759804, 114.7726862821014322, -8.927990412390657937 ) ) ;
#36781=CARTESIAN_POINT ( 'NONE',  ( 12.53471296425194836, 17.02268628210144996, -2.311890736173178418 ) ) ;
#36785=CARTESIAN_POINT ( 'NONE',  ( -5.233372021372430183, 78.54768628210145209, -8.152565276336710909 ) ) ;
#36794=CARTESIAN_POINT ( 'NONE',  ( -5.233372021372612259, 51.05231371789854222, 8.152565276336593669 ) ) ;
#36798=CARTESIAN_POINT ( 'NONE',  ( -4.944772684328424539, 63.41481371789856070, -11.48171059495408031 ) ) ;
#36802=CARTESIAN_POINT ( 'NONE',  ( 12.46528703574811558, 29.20231371789855501, -2.660918448318005503 ) ) ;
#36807=CARTESIAN_POINT ( 'NONE',  ( 6.932735513423970097, 9.547686282101453870, 10.69584247140445044 ) ) ;
#36813=CARTESIAN_POINT ( 'NONE',  ( 2.660918448318002838, 68.30231371789854222, 12.46528703574811558 ) ) ;
#36819=CARTESIAN_POINT ( 'NONE',  ( -15.50000000000000533, 43.28981371789856070, 0.1745138560722471477 ) ) ;
#36821=CARTESIAN_POINT ( 'NONE',  ( -0.1745138560725500443, 19.61018628210144144, 12.50000000000000355 ) ) ;
#36823=CARTESIAN_POINT ( 'NONE',  ( -8.715434833791929847, 59.86018628210145209, -8.962234695871762469 ) ) ;
#36824=CARTESIAN_POINT ( 'NONE',  ( -14.25334919248782306, 4.085186282101443744, -6.092822981423979378 ) ) ;
#36828=CARTESIAN_POINT ( 'NONE',  ( -5.770363421893818234, 23.63518628210144357, -14.38691631536207005 ) ) ;
#36833=CARTESIAN_POINT ( 'NONE',  ( -6.932735513423968321, 4.947686282101432909, -10.69584247140445221 ) ) ;
#36835=CARTESIAN_POINT ( 'NONE',  ( 6.840914352311949109, 113.4398137178985593, 6.594114490232462877 ) ) ;
#36841=CARTESIAN_POINT ( 'NONE',  ( -12.53471296425189152, 126.3773137178985593, -2.311890736173453309 ) ) ;
#36854=CARTESIAN_POINT ( 'NONE',  ( 2.660918448318279950, 61.29768628210143788, -12.46528703574805697 ) ) ;
#36860=CARTESIAN_POINT ( 'NONE',  ( -2.311890736173448424, 124.0773137178985621, 12.53471296425189330 ) ) ;
#36865=CARTESIAN_POINT ( 'NONE',  ( -14.38691631536193860, 89.86481371789855643, -5.770363421894132649 ) ) ;
#36869=CARTESIAN_POINT ( 'NONE',  ( 10.49813415415989581, 119.3726862821014549, 7.228626920339068285 ) ) ;
#36870=CARTESIAN_POINT ( 'NONE',  ( 14.25334919248782661, 63.88518628210145778, 6.092822981423971385 ) ) ;
#36873=CARTESIAN_POINT ( 'NONE',  ( 15.53471296425195369, 90.62268628210145494, -2.908627838312120684 ) ) ;
#36876=CARTESIAN_POINT ( 'NONE',  ( -1.715153634034234598, 23.92268628210143788, -9.534712964251941258 ) ) ;
#36880=CARTESIAN_POINT ( 'NONE',  ( -11.48171059495397373, 59.28518628210144215, -4.944772684328680334 ) ) ;
#36883=CARTESIAN_POINT ( 'NONE',  ( 7.954856959092191815, 18.17268628210144499, 5.529263428287477744 ) ) ;
#36894=CARTESIAN_POINT ( 'NONE',  ( 0.1745138560725515708, 79.41018628210144925, -12.50000000000000355 ) ) ;
#36899=CARTESIAN_POINT ( 'NONE',  ( -13.23911966647199812, 62.55231371789854222, -8.632099005475788900 ) ) ;
#36903=CARTESIAN_POINT ( 'NONE',  ( -3.474262827703527901, 32.36481371789854933, 8.843639120294245259 ) ) ;
#36907=CARTESIAN_POINT ( 'NONE',  ( 8.843639120294245259, 103.6648137178985678, 3.474262827703527901 ) ) ;
#36909=CARTESIAN_POINT ( 'NONE',  ( -15.50000000000000533, 144.4898137178985280, 0.1745138560722471477 ) ) ;
#36910=CARTESIAN_POINT ( 'NONE',  ( -4.944772684328673229, 66.18518628210144072, 11.48171059495397728 ) ) ;
#36919=CARTESIAN_POINT ( 'NONE',  ( -9.465287035748065847, 68.19768628210142936, -2.064181346179273735 ) ) ;
#36922=CARTESIAN_POINT ( 'NONE',  ( -2.311890736173176641, 115.9226862821014521, -12.53471296425194836 ) ) ;
#36936=CARTESIAN_POINT ( 'NONE',  ( 11.61527771782809637, 131.2648137178985621, 4.622313124798827388 ) ) ;
#36937=CARTESIAN_POINT ( 'NONE',  ( -6.932735513423968321, 133.7476862821014549, -10.69584247140445221 ) ) ;
#36944=CARTESIAN_POINT ( 'NONE',  ( -8.632099005475794229, 115.4523137178985479, 13.23911966647199812 ) ) ;
#36949=CARTESIAN_POINT ( 'NONE',  ( -10.49813415415989581, 105.5726862821014578, -7.228626920339068285 ) ) ;
#36957=CARTESIAN_POINT ( 'NONE',  ( 11.61527771782819940, 127.1351862821014578, -4.622313124798573369 ) ) ;
#36964=CARTESIAN_POINT ( 'NONE',  ( -13.04141134922759804, 123.9726862821014493, -8.927990412390657937 ) ) ;
#36965=CARTESIAN_POINT ( 'NONE',  ( 2.660918448318279950, 24.49768628210144428, -12.46528703574805874 ) ) ;
#36968=CARTESIAN_POINT ( 'NONE',  ( -3.474262827703337830, 134.0351862821014493, -8.843639120294326972 ) ) ;
#36973=CARTESIAN_POINT ( 'NONE',  ( -2.064181346179269738, 75.09768628210143504, 9.465287035748067623 ) ) ;
#36981=CARTESIAN_POINT ( 'NONE',  ( 6.840914352311949109, 49.03981371789855359, 6.594114490232462877 ) ) ;
#36985=CARTESIAN_POINT ( 'NONE',  ( 4.622313124798831829, 64.56481371789855928, -11.61527771782809282 ) ) ;
#36988=CARTESIAN_POINT ( 'NONE',  ( -12.46528703574811558, 24.60231371789854649, 2.660918448318003726 ) ) ;
#36992=CARTESIAN_POINT ( 'NONE',  ( 11.48171059495397728, 8.685186282101437172, 4.944772684328674117 ) ) ;
#37003=CARTESIAN_POINT ( 'NONE',  ( -14.38691631536193860, 34.66481371789854649, -5.770363421894132649 ) ) ;
#37005=CARTESIAN_POINT ( 'NONE',  ( -8.962234695871760692, 11.56018628210145316, 8.715434833791933400 ) ) ;
#37007=CARTESIAN_POINT ( 'NONE',  ( -10.49813415415989581, 68.77268628210146062, -7.228626920339068285 ) ) ;
#37008=CARTESIAN_POINT ( 'NONE',  ( -8.632099005475501130, 14.14768628210144286, -13.23911966647218996 ) ) ;
#37012=CARTESIAN_POINT ( 'NONE',  ( -12.50000000000000355, 141.5101862821014720, -0.1745138560725492671 ) ) ;
#37017=CARTESIAN_POINT ( 'NONE',  ( -8.715434833791929847, 4.660186282101435928, -8.962234695871762469 ) ) ;
#37019=CARTESIAN_POINT ( 'NONE',  ( -9.534712964251895073, 107.9773137178985394, -1.715153634034446428 ) ) ;
#37025=CARTESIAN_POINT ( 'NONE',  ( 0.1745138560722779009, 114.5898137178985650, 12.50000000000000355 ) ) ;
#37038=CARTESIAN_POINT ( 'NONE',  ( 2.311890736173175753, 65.32268628210144357, 12.53471296425194836 ) ) ;
#37046=CARTESIAN_POINT ( 'NONE',  ( 7.228626920338837358, 113.7273137178985820, 10.49813415416005036 ) ) ;
#37052=CARTESIAN_POINT ( 'NONE',  ( -13.23911966647199812, 99.35231371789856780, -8.632099005475788900 ) ) ;
#37057=CARTESIAN_POINT ( 'NONE',  ( 4.622313124798573369, 129.4351862821014549, 11.61527771782819940 ) ) ;
#37058=CARTESIAN_POINT ( 'NONE',  ( 8.927990412390657937, 61.87268628210144783, -13.04141134922759804 ) ) ;
#37061=CARTESIAN_POINT ( 'NONE',  ( -2.908627838312119351, 79.12268628210145494, -15.53471296425195369 ) ) ;
#37063=CARTESIAN_POINT ( 'NONE',  ( 9.465287035748067623, 26.79768628210144144, 2.064181346179272847 ) ) ;
#37067=CARTESIAN_POINT ( 'NONE',  ( 4.622313124798573369, 55.83518628210144641, 11.61527771782819940 ) ) ;
#37070=CARTESIAN_POINT ( 'NONE',  ( -7.954856959092191815, 22.77268628210143220, -5.529263428287477744 ) ) ;
#37082=CARTESIAN_POINT ( 'NONE',  ( -8.715434833791929847, 69.06018628210145494, -8.962234695871762469 ) ) ;
#37087=CARTESIAN_POINT ( 'NONE',  ( 0.1745138560722461762, 31.78981371789855004, 15.50000000000000533 ) ) ;
#37093=CARTESIAN_POINT ( 'NONE',  ( 9.534712964251900402, 48.17731371789854222, 1.715153634034445540 ) ) ;
#37096=CARTESIAN_POINT ( 'NONE',  ( 5.529263428287300108, 86.12731371789853085, 7.954856959092309943 ) ) ;
#37098=CARTESIAN_POINT ( 'NONE',  ( -12.53471296425189152, 15.97731371789853760, -2.311890736173453753 ) ) ;
#37099=CARTESIAN_POINT ( 'NONE',  ( 12.53471296425194836, 72.22268628210143504, -2.311890736173178418 ) ) ;
#37108=CARTESIAN_POINT ( 'NONE',  ( -8.710071997420127943, 77.68518628210145494, -3.796722387233380402 ) ) ;
#37110=CARTESIAN_POINT ( 'NONE',  ( 7.228626920339068285, 107.8726862821014549, -10.49813415415989581 ) ) ;
#37123=CARTESIAN_POINT ( 'NONE',  ( 10.49813415416005213, 120.6273137178985735, -7.228626920338837358 ) ) ;
#37124=CARTESIAN_POINT ( 'NONE',  ( -12.46528703574805874, 132.5976862821014777, -2.660918448318280838 ) ) ;
#37130=CARTESIAN_POINT ( 'NONE',  ( 5.770363421894130873, 101.3648137178985706, -14.38691631536193860 ) ) ;
#37136=CARTESIAN_POINT ( 'NONE',  ( -7.228626920339069173, 121.6726862821014521, 10.49813415415989581 ) ) ;
#37138=AXIS2_PLACEMENT_3D ( 'NONE', #25477, #25292, #19628 ) ;
#37144=CARTESIAN_POINT ( 'NONE',  ( -12.46528703574805697, 123.3976862821014606, -2.660918448318280838 ) ) ;
#37150=CARTESIAN_POINT ( 'NONE',  ( 6.092822981423978490, 98.38518628210145778, -14.25334919248782306 ) ) ;
#37151=CARTESIAN_POINT ( 'NONE',  ( 2.311890736173175753, 19.32268628210144357, 12.53471296425194659 ) ) ;
#37154=CARTESIAN_POINT ( 'NONE',  ( -8.843639120294326972, 140.9351862821014549, 3.474262827703335166 ) ) ;
#37160=CARTESIAN_POINT ( 'NONE',  ( 0.1745138560725194299, 70.21018628210144641, -9.500000000000005329 ) ) ;
#37168=CARTESIAN_POINT ( 'NONE',  ( -6.594114490232462877, 32.93981371789854506, 6.840914352311949109 ) ) ;
#37172=CARTESIAN_POINT ( 'NONE',  ( 10.49813415416005213, 56.22731371789854649, -7.228626920338837358 ) ) ;
#37175=CARTESIAN_POINT ( 'NONE',  ( 7.228626920338837358, 21.72731371789854649, 10.49813415416005036 ) ) ;
#37179=CARTESIAN_POINT ( 'NONE',  ( -7.228626920339069173, 11.27268628210143042, 10.49813415415989581 ) ) ;
#37190=CARTESIAN_POINT ( 'NONE',  ( -15.46528703574811736, 15.40231371789854720, 3.257655550456946436 ) ) ;
#37192=CARTESIAN_POINT ( 'NONE',  ( -11.61527771782819940, 12.13518628210144534, 4.622313124798574258 ) ) ;
#37193=CARTESIAN_POINT ( 'NONE',  ( 11.48171059495397728, 45.48518628210145209, 4.944772684328674117 ) ) ;
#37197=CARTESIAN_POINT ( 'NONE',  ( 13.04141134922759804, 18.17268628210144499, 8.927990412390657937 ) ) ;
#37204=CARTESIAN_POINT ( 'NONE',  ( 8.710071997420211432, 111.7148137178985792, -3.796722387233181895 ) ) ;
#37212=CARTESIAN_POINT ( 'NONE',  ( -12.53471296425189152, 117.1773137178985706, -2.311890736173453309 ) ) ;
#37227=CARTESIAN_POINT ( 'NONE',  ( 10.69584247140445221, 62.44768628210145778, -6.932735513423970097 ) ) ;
#37232=CARTESIAN_POINT ( 'NONE',  ( -11.61527771782809282, 99.06481371789855928, -4.622313124798832717 ) ) ;
#37237=CARTESIAN_POINT ( 'NONE',  ( 2.908627838312458636, 82.67731371789852801, -15.53471296425188442 ) ) ;
#37241=CARTESIAN_POINT ( 'NONE',  ( -2.311890736173176641, 97.52268628210144641, -12.53471296425194836 ) ) ;
#37242=CARTESIAN_POINT ( 'NONE',  ( -8.927990412390661490, 66.47268628210146346, 13.04141134922759804 ) ) ;
#37246=CARTESIAN_POINT ( 'NONE',  ( -13.04141134922759804, 68.77268628210143220, -8.927990412390657937 ) ) ;
#37249=CARTESIAN_POINT ( 'NONE',  ( -8.710071997420127943, 22.48518628210144499, -3.796722387233380402 ) ) ;
#37253=CARTESIAN_POINT ( 'NONE',  ( 4.622313124798573369, 37.43518628210144783, 11.61527771782819940 ) ) ;
#37256=CARTESIAN_POINT ( 'NONE',  ( 7.954856959092191815, 27.37268628210144428, 5.529263428287477744 ) ) ;
#37268=CARTESIAN_POINT ( 'NONE',  ( 12.50000000000000355, 72.51018628210145778, 0.1745138560725507937 ) ) ;
#37273=CARTESIAN_POINT ( 'NONE',  ( -13.04141134922778456, 42.42731371789855643, 8.927990412390377273 ) ) ;
#37280=CARTESIAN_POINT ( 'NONE',  ( -6.840914352311947333, 16.83981371789855430, -6.594114490232462877 ) ) ;
#37284=CARTESIAN_POINT ( 'NONE',  ( 4.944772684328420986, 12.81481371789855395, 11.48171059495408208 ) ) ;
#37287=CARTESIAN_POINT ( 'NONE',  ( 7.228626920339068285, 61.87268628210145494, -10.49813415415989581 ) ) ;
#37294=CARTESIAN_POINT ( 'NONE',  ( -5.529263428287477744, 84.87268628210145494, 7.954856959092191815 ) ) ;
#37296=CARTESIAN_POINT ( 'NONE',  ( 11.61527771782819940, 108.7351862821014663, -4.622313124798573369 ) ) ;
#37308=CARTESIAN_POINT ( 'NONE',  ( 12.50000000000000355, 130.6898137178985735, -0.1745138560722771515 ) ) ;
#37309=CARTESIAN_POINT ( 'NONE',  ( -2.660918448318275509, 121.0976862821014635, 12.46528703574805874 ) ) ;
#37315=CARTESIAN_POINT ( 'NONE',  ( 13.04141134922778988, 102.2273137178985678, -8.927990412390371944 ) ) ;
#37316=CARTESIAN_POINT ( 'NONE',  ( -12.53471296425194836, 95.22268628210146346, 2.311890736173176641 ) ) ;
#37319=CARTESIAN_POINT ( 'NONE',  ( -10.69584247140444866, 113.0476862821014663, 6.932735513423972762 ) ) ;
#37324=CARTESIAN_POINT ( 'NONE',  ( -10.69584247140444866, 113.0476862821014663, 6.932735513423972762 ) ) ;
#37329=CARTESIAN_POINT ( 'NONE',  ( -5.770363421893818234, 106.4351862821014691, -14.38691631536207005 ) ) ;
#37330=CARTESIAN_POINT ( 'NONE',  ( 11.48171059495397728, 17.88518628210143646, 4.944772684328674117 ) ) ;
#37333=CARTESIAN_POINT ( 'NONE',  ( 8.152565276336714462, 136.0476862821014379, -5.233372021372432847 ) ) ;
#37337=CARTESIAN_POINT ( 'NONE',  ( -6.840914352312096547, 66.76018628210144357, 6.594114490232313663 ) ) ;
#37344=CARTESIAN_POINT ( 'NONE',  ( 8.710071997420211432, 38.11481371789853512, -3.796722387233181895 ) ) ;
#37349=CARTESIAN_POINT ( 'NONE',  ( -12.46528703574811558, 43.00231371789854506, 2.660918448318004170 ) ) ;
#37352=CARTESIAN_POINT ( 'NONE',  ( 0.1745138560722461762, 142.1898137178985451, 15.50000000000000533 ) ) ;
#37369=CARTESIAN_POINT ( 'NONE',  ( -5.770363421894122880, 23.16481371789855359, 14.38691631536194393 ) ) ;
#37372=CARTESIAN_POINT ( 'NONE',  ( -7.228626920339069173, 11.27268628210143042, 10.49813415415989581 ) ) ;
#37373=CARTESIAN_POINT ( 'NONE',  ( 8.715434833791931624, 55.26018628210144357, 8.962234695871760692 ) ) ;
#37384=CARTESIAN_POINT ( 'NONE',  ( 8.710071997420211432, 93.31481371789855928, -3.796722387233181895 ) ) ;
#37393=CARTESIAN_POINT ( 'NONE',  ( -6.932735513424201912, 115.4523137178985621, 10.69584247140429412 ) ) ;
#37397=CARTESIAN_POINT ( 'NONE',  ( 10.69584247140429589, 57.95231371789854791, 6.932735513424201024 ) ) ;
#37406=CARTESIAN_POINT ( 'NONE',  ( 4.944772684328679446, 61.58518628210145351, -11.48171059495397373 ) ) ;
#37413=CARTESIAN_POINT ( 'NONE',  ( -4.622313124798826500, 96.76481371789854791, 11.61527771782809637 ) ) ;
#37418=CARTESIAN_POINT ( 'NONE',  ( 11.08355503943118769, 67.43981371789855928, 10.83675517735179028 ) ) ;
#37423=CARTESIAN_POINT ( 'NONE',  ( -7.228626920339069173, 103.2726862821014606, 10.49813415415989581 ) ) ;
#37424=CARTESIAN_POINT ( 'NONE',  ( -8.927990412390661490, 48.07268628210143646, 13.04141134922759804 ) ) ;
#37427=CARTESIAN_POINT ( 'NONE',  ( 14.38691631536207538, 62.73518628210145920, -5.770363421893813793 ) ) ;
#37433=CARTESIAN_POINT ( 'NONE',  ( -8.962234695871760692, 48.36018628210145209, 8.715434833791933400 ) ) ;
#37437=CARTESIAN_POINT ( 'NONE',  ( -7.954856959092191815, 13.57268628210145422, -5.529263428287477744 ) ) ;
#37447=CARTESIAN_POINT ( 'NONE',  ( 12.53471296425194659, 72.22268628210144925, -2.311890736173178418 ) ) ;
#37453=CARTESIAN_POINT ( 'NONE',  ( -8.632099005475794229, 32.65231371789855075, 13.23911966647199812 ) ) ;
#37459=CARTESIAN_POINT ( 'NONE',  ( -7.954856959092309943, 14.82731371789855324, 5.529263428287300108 ) ) ;
#37464=CARTESIAN_POINT ( 'NONE',  ( 11.08355503943118769, 131.8398137178985792, 10.83675517735179028 ) ) ;
#37467=CARTESIAN_POINT ( 'NONE',  ( 6.932735513423970097, 37.14768628210143930, 10.69584247140445044 ) ) ;
#37474=CARTESIAN_POINT ( 'NONE',  ( 5.529263428287477744, 71.07268628210144357, -7.954856959092191815 ) ) ;
#37476=CARTESIAN_POINT ( 'NONE',  ( -0.1745138560725500443, 93.21018628210146062, 12.50000000000000355 ) ) ;
#37488=CARTESIAN_POINT ( 'NONE',  ( 6.932735513424201024, 129.2523137178985451, -10.69584247140429412 ) ) ;
#37489=CARTESIAN_POINT ( 'NONE',  ( -12.50000000000000355, 123.1101862821014663, -0.1745138560725492671 ) ) ;
#37495=CARTESIAN_POINT ( 'NONE',  ( -13.23911966647199812, 99.35231371789856780, -8.632099005475788900 ) ) ;
#37498=CARTESIAN_POINT ( 'NONE',  ( -2.064181346179062349, 72.90231371789855075, -9.465287035748106703 ) ) ;
#37500=CARTESIAN_POINT ( 'NONE',  ( 3.796722387233379514, 135.1851862821014549, -8.710071997420127943 ) ) ;
#37536=COLOUR_RGB('Grey',0.48,0.52,0.57);
#37537=FILL_AREA_STYLE_COLOUR('',#37536);
#37538=FILL_AREA_STYLE('',(#37537));
#37539=SURFACE_STYLE_FILL_AREA(#37538);
#37540=SURFACE_SIDE_STYLE('',(#37539));
#37541=SURFACE_STYLE_USAGE(.BOTH.,#37540);
#37542=PRESENTATION_STYLE_ASSIGNMENT((#37541));
ENDSEC;
END-ISO-10303-21;
